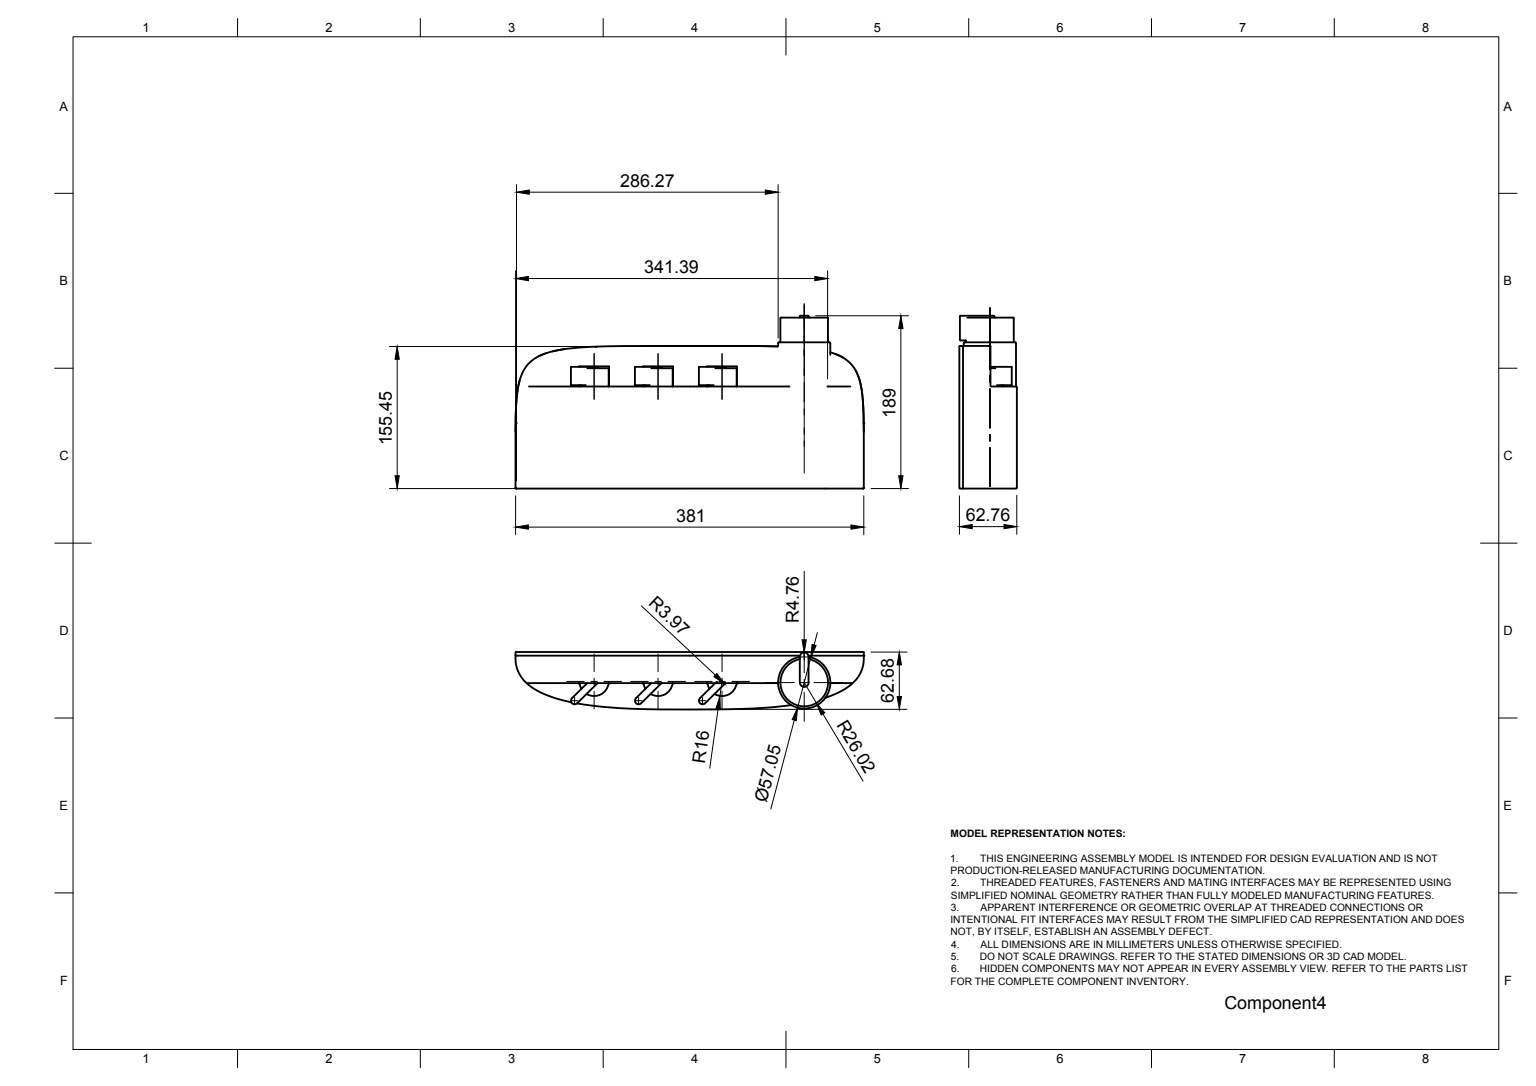
ISO-10303-21;
HEADER;
/* Generated by software containing ST-Developer
 * from STEP Tools, Inc. (www.steptools.com) 
 */

FILE_DESCRIPTION(
/* description */ ('STEP AP214'),
/* implementation_level */ '2;1');

FILE_NAME(
/* name */ 'Component4.step',
/* time_stamp */ '2026-10-06T11:02:40-07:00',
/* author */ (''),
/* organization */ (''),
/* preprocessor_version */ 'ST-DEVELOPER v20.2',
/* originating_system */ 'Autodesk Translation Framework v15.15.0.0',
/* authorisation */ '');

FILE_SCHEMA (('AUTOMOTIVE_DESIGN { 1 0 10303 214 3 1 1 }'));
ENDSEC;

DATA;
#10=MECHANICAL_DESIGN_GEOMETRIC_PRESENTATION_REPRESENTATION('',(#2939),#130910);
#50=B_SPLINE_SURFACE_WITH_KNOTS('',3,1,((#87618,#87619),(#87620,#87621),
(#87622,#87623),(#87624,#87625)),.UNSPECIFIED.,.F.,.F.,.F.,(4,4),(2,2),
(0.0749476459249852,1.),(0.,0.360000000000005),.UNSPECIFIED.);
#51=B_SPLINE_SURFACE_WITH_KNOTS('',3,1,((#88063,#88064),(#88065,#88066),
(#88067,#88068),(#88069,#88070)),.UNSPECIFIED.,.F.,.F.,.F.,(4,4),(2,2),
(0.,0.925052354075012),(0.,0.360000000000003),.UNSPECIFIED.);
#52=B_SPLINE_SURFACE_WITH_KNOTS('',3,1,((#96549,#96550),(#96551,#96552),
(#96553,#96554),(#96555,#96556)),.UNSPECIFIED.,.F.,.F.,.F.,(4,4),(2,2),
(0.0749476459249852,1.),(0.,3.46611820003485),.UNSPECIFIED.);
#53=B_SPLINE_SURFACE_WITH_KNOTS('',3,1,((#96558,#96559),(#96560,#96561),
(#96562,#96563),(#96564,#96565)),.UNSPECIFIED.,.F.,.F.,.F.,(4,4),(2,2),
(0.309194334580351,0.92505235407501),(0.,1.8569103791729),.UNSPECIFIED.);
#54=B_SPLINE_SURFACE_WITH_KNOTS('',3,1,((#96571,#96572),(#96573,#96574),
(#96575,#96576),(#96577,#96578)),.UNSPECIFIED.,.F.,.F.,.F.,(4,4),(2,2),
(0.62139116379009,1.),(0.,13.1529900906224),.UNSPECIFIED.);
#55=B_SPLINE_SURFACE_WITH_KNOTS('',3,1,((#96579,#96580),(#96581,#96582),
(#96583,#96584),(#96585,#96586)),.UNSPECIFIED.,.F.,.F.,.F.,(4,4),(2,2),
(0.,1.),(0.,13.1529900906224),.UNSPECIFIED.);
#56=B_SPLINE_SURFACE_WITH_KNOTS('',3,1,((#96901,#96902),(#96903,#96904),
(#96905,#96906),(#96907,#96908)),.UNSPECIFIED.,.F.,.F.,.F.,(4,4),(2,2),
(0.,0.448741420101952),(0.,13.1529900906224),.UNSPECIFIED.);
#57=B_SPLINE_SURFACE_WITH_KNOTS('',3,1,((#96909,#96910),(#96911,#96912),
(#96913,#96914),(#96915,#96916)),.UNSPECIFIED.,.F.,.F.,.F.,(4,4),(2,2),
(0.,0.274332977827422),(0.,3.42421373123634),.UNSPECIFIED.);
#60=SPHERICAL_SURFACE('',#48303,0.5);
#61=SPHERICAL_SURFACE('',#48305,0.5);
#62=SPHERICAL_SURFACE('',#48314,0.5);
#63=SPHERICAL_SURFACE('',#48316,0.5);
#64=SPHERICAL_SURFACE('',#48525,1.);
#65=SPHERICAL_SURFACE('',#48533,1.);
#717=FACE_BOUND('',#15125,.T.);
#718=FACE_BOUND('',#15135,.T.);
#719=FACE_BOUND('',#15136,.T.);
#720=FACE_BOUND('',#15137,.T.);
#1607=(
BOUNDED_SURFACE()
B_SPLINE_SURFACE(3,2,((#88517,#88518,#88519),(#88520,#88521,#88522),(#88523,
#88524,#88525),(#88526,#88527,#88528),(#88529,#88530,#88531),(#88532,#88533,
#88534),(#88535,#88536,#88537),(#88538,#88539,#88540),(#88541,#88542,#88543),
(#88544,#88545,#88546),(#88547,#88548,#88549),(#88550,#88551,#88552),(#88553,
#88554,#88555),(#88556,#88557,#88558),(#88559,#88560,#88561),(#88562,#88563,
#88564),(#88565,#88566,#88567),(#88568,#88569,#88570),(#88571,#88572,#88573),
(#88574,#88575,#88576),(#88577,#88578,#88579),(#88580,#88581,#88582),(#88583,
#88584,#88585),(#88586,#88587,#88588),(#88589,#88590,#88591),(#88592,#88593,
#88594),(#88595,#88596,#88597),(#88598,#88599,#88600),(#88601,#88602,#88603),
(#88604,#88605,#88606),(#88607,#88608,#88609),(#88610,#88611,#88612),(#88613,
#88614,#88615),(#88616,#88617,#88618),(#88619,#88620,#88621),(#88622,#88623,
#88624),(#88625,#88626,#88627),(#88628,#88629,#88630),(#88631,#88632,#88633),
(#88634,#88635,#88636),(#88637,#88638,#88639),(#88640,#88641,#88642),(#88643,
#88644,#88645),(#88646,#88647,#88648),(#88649,#88650,#88651),(#88652,#88653,
#88654),(#88655,#88656,#88657),(#88658,#88659,#88660),(#88661,#88662,#88663),
(#88664,#88665,#88666),(#88667,#88668,#88669),(#88670,#88671,#88672),(#88673,
#88674,#88675),(#88676,#88677,#88678),(#88679,#88680,#88681),(#88682,#88683,
#88684),(#88685,#88686,#88687),(#88688,#88689,#88690)),.UNSPECIFIED.,.F.,
 .F.,.F.)
B_SPLINE_SURFACE_WITH_KNOTS((4,2,2,2,2,2,2,2,2,2,2,2,2,2,2,2,2,2,2,2,2,
2,2,2,2,2,2,2,4),(3,3),(0.,0.0321349777273596,0.0642699554547192,0.080337444318399,
0.0964049331820788,0.112472422045759,0.128539910909438,0.136573655341278,
0.140590527557198,0.144607399773118,0.152641144204958,0.156658016420878,
0.160674888636798,0.168708633068638,0.172725505284558,0.174733941392518,
0.176742377500478,0.184776121932318,0.186784558040278,0.188792994148238,
0.192809866364158,0.200843610795998,0.204860483011918,0.208877355227837,
0.216911099659677,0.224944844091517,0.232978588523357,0.241012332955197,
0.25739509415827),(0.295972225728062,1.),.UNSPECIFIED.)
GEOMETRIC_REPRESENTATION_ITEM()
RATIONAL_B_SPLINE_SURFACE(((0.877938117508499,0.793795039059425,1.),(0.877938117508499,
0.793795039059425,1.),(0.877938117508498,0.793795039059421,1.),(0.877938117508498,
0.793795039059421,1.),(0.877938117508498,0.793795039059421,1.),(0.877938117508498,
0.793795039059421,1.),(0.877938117508498,0.793795039059421,1.),(0.877938117508498,
0.793795039059421,1.),(0.877938117508499,0.793795039059425,1.),(0.877938117508499,
0.793795039059425,1.),(0.877938117508489,0.793795039059407,1.),(0.877938117508489,
0.793795039059407,1.),(0.877938117508506,0.793795039059435,1.),(0.877938117508506,
0.793795039059435,1.),(0.877938117508499,0.793795039059425,1.),(0.877938117508499,
0.793795039059425,1.),(0.877938117508499,0.793795039059425,1.),(0.877938117508499,
0.793795039059425,1.),(0.877938117508498,0.793795039059421,1.),(0.877938117508498,
0.793795039059421,1.),(0.877938117508485,0.793795039059401,1.),(0.877938117508485,
0.793795039059401,1.),(0.877938117508505,0.793795039059434,1.),(0.877938117508505,
0.793795039059434,1.),(0.87793811750849,0.793795039059408,1.),(0.87793811750849,
0.793795039059408,1.),(0.87793811750849,0.793795039059409,1.),(0.87793811750849,
0.793795039059409,1.),(0.877938117508486,0.793795039059402,1.),(0.877938117508486,
0.793795039059402,1.),(0.877938117508504,0.793795039059432,1.),(0.877938117508504,
0.793795039059432,1.),(0.877938117508498,0.793795039059421,1.),(0.877938117508498,
0.793795039059421,1.),(0.877938117508506,0.793795039059436,1.),(0.877938117508506,
0.793795039059436,1.),(0.877938117508498,0.793795039059421,1.),(0.877938117508498,
0.793795039059421,1.),(0.877938117508493,0.793795039059414,1.),(0.877938117508493,
0.793795039059414,1.),(0.877938117508498,0.793795039059421,1.),(0.877938117508498,
0.793795039059421,1.),(0.877938117508498,0.793795039059421,1.),(0.877938117508498,
0.793795039059421,1.),(0.877938117508489,0.793795039059408,1.),(0.877938117508489,
0.793795039059408,1.),(0.877938117508506,0.793795039059435,1.),(0.877938117508506,
0.793795039059435,1.),(0.877938117508489,0.793795039059408,1.),(0.877938117508489,
0.793795039059408,1.),(0.877938117508498,0.793795039059421,1.),(0.877938117508498,
0.793795039059421,1.),(0.877938117508506,0.793795039059435,1.),(0.877938117508506,
0.793795039059435,1.),(0.877938117508506,0.793795039059435,1.),(0.877938117508506,
0.793795039059435,1.),(0.877938117508499,0.793795039059424,1.),(0.877938117508499,
0.793795039059425,1.)))
REPRESENTATION_ITEM('')
SURFACE()
);
#1608=(
BOUNDED_SURFACE()
B_SPLINE_SURFACE(3,2,((#88828,#88829,#88830),(#88831,#88832,#88833),(#88834,
#88835,#88836),(#88837,#88838,#88839),(#88840,#88841,#88842),(#88843,#88844,
#88845),(#88846,#88847,#88848),(#88849,#88850,#88851),(#88852,#88853,#88854),
(#88855,#88856,#88857),(#88858,#88859,#88860),(#88861,#88862,#88863),(#88864,
#88865,#88866),(#88867,#88868,#88869),(#88870,#88871,#88872),(#88873,#88874,
#88875),(#88876,#88877,#88878),(#88879,#88880,#88881),(#88882,#88883,#88884),
(#88885,#88886,#88887),(#88888,#88889,#88890),(#88891,#88892,#88893),(#88894,
#88895,#88896),(#88897,#88898,#88899),(#88900,#88901,#88902),(#88903,#88904,
#88905),(#88906,#88907,#88908),(#88909,#88910,#88911),(#88912,#88913,#88914),
(#88915,#88916,#88917),(#88918,#88919,#88920),(#88921,#88922,#88923),(#88924,
#88925,#88926),(#88927,#88928,#88929),(#88930,#88931,#88932),(#88933,#88934,
#88935),(#88936,#88937,#88938),(#88939,#88940,#88941),(#88942,#88943,#88944),
(#88945,#88946,#88947),(#88948,#88949,#88950),(#88951,#88952,#88953),(#88954,
#88955,#88956),(#88957,#88958,#88959),(#88960,#88961,#88962),(#88963,#88964,
#88965),(#88966,#88967,#88968),(#88969,#88970,#88971),(#88972,#88973,#88974),
(#88975,#88976,#88977),(#88978,#88979,#88980),(#88981,#88982,#88983),(#88984,
#88985,#88986),(#88987,#88988,#88989),(#88990,#88991,#88992),(#88993,#88994,
#88995)),.UNSPECIFIED.,.F.,.F.,.F.)
B_SPLINE_SURFACE_WITH_KNOTS((4,2,2,2,2,2,2,2,2,2,2,2,2,2,2,2,2,2,2,2,2,
2,2,2,2,2,2,4),(3,3),(0.,0.0161428187212414,0.0242142280818621,0.0322856374424828,
0.0403570468031035,0.0484284561637242,0.0564998655243449,0.0605355702046552,
0.0645712748849656,0.0686069795652759,0.0706248319054311,0.0726426842455863,
0.0807140936062069,0.0847497982865173,0.0867676506266725,0.0887855029668276,
0.0968569123274483,0.100892617007759,0.104928321688069,0.11299973104869,
0.12107114040931,0.129142549769931,0.145285368491173,0.161428187212414,
0.177571005933655,0.193713824654897,0.225999462097379,0.258285099539862),
(0.296287498067819,1.),.UNSPECIFIED.)
GEOMETRIC_REPRESENTATION_ITEM()
RATIONAL_B_SPLINE_SURFACE(((0.877862815112484,0.793887380189833,1.),(0.877862815112484,
0.793887380189833,1.),(0.877862815112466,0.793887380189802,1.),(0.877862815112466,
0.793887380189802,1.),(0.87786281511247,0.793887380189809,1.),(0.87786281511247,
0.793887380189809,1.),(0.877862815112476,0.793887380189819,1.),(0.877862815112476,
0.793887380189819,1.),(0.877862815112474,0.793887380189816,1.),(0.877862815112474,
0.793887380189816,1.),(0.877862815112474,0.793887380189816,1.),(0.877862815112474,
0.793887380189816,1.),(0.877862815112476,0.793887380189819,1.),(0.877862815112476,
0.793887380189819,1.),(0.877862815112474,0.793887380189816,1.),(0.877862815112474,
0.793887380189816,1.),(0.877862815112481,0.793887380189828,1.),(0.877862815112481,
0.793887380189828,1.),(0.877862815112485,0.793887380189834,1.),(0.877862815112485,
0.793887380189834,1.),(0.877862815112478,0.793887380189823,1.),(0.877862815112478,
0.793887380189823,1.),(0.877862815112464,0.7938873801898,1.),(0.877862815112464,
0.7938873801898,1.),(0.877862815112474,0.793887380189816,1.),(0.877862815112474,
0.793887380189816,1.),(0.877862815112474,0.793887380189816,1.),(0.877862815112474,
0.793887380189816,1.),(0.877862815112474,0.793887380189816,1.),(0.877862815112474,
0.793887380189816,1.),(0.877862815112474,0.793887380189816,1.),(0.877862815112474,
0.793887380189816,1.),(0.877862815112472,0.793887380189812,1.),(0.877862815112472,
0.793887380189812,1.),(0.877862815112482,0.793887380189829,1.),(0.877862815112482,
0.793887380189829,1.),(0.877862815112466,0.793887380189802,1.),(0.877862815112466,
0.793887380189802,1.),(0.877862815112476,0.793887380189819,1.),(0.877862815112476,
0.793887380189819,1.),(0.877862815112466,0.793887380189802,1.),(0.877862815112466,
0.793887380189802,1.),(0.877862815112474,0.793887380189816,1.),(0.877862815112474,
0.793887380189816,1.),(0.877862815112474,0.793887380189815,1.),(0.877862815112474,
0.793887380189815,1.),(0.877862815112484,0.793887380189833,1.),(0.877862815112484,
0.793887380189833,1.),(0.877862815112461,0.793887380189795,1.),(0.877862815112461,
0.793887380189795,1.),(0.877862815112466,0.793887380189802,1.),(0.877862815112466,
0.793887380189802,1.),(0.877862815112474,0.793887380189816,1.),(0.877862815112474,
0.793887380189816,1.),(0.877862815112476,0.793887380189819,1.),(0.877862815112476,
0.793887380189819,1.)))
REPRESENTATION_ITEM('')
SURFACE()
);
#1609=(
BOUNDED_SURFACE()
B_SPLINE_SURFACE(3,2,((#89355,#89356,#89357),(#89358,#89359,#89360),(#89361,
#89362,#89363),(#89364,#89365,#89366),(#89367,#89368,#89369),(#89370,#89371,
#89372),(#89373,#89374,#89375),(#89376,#89377,#89378),(#89379,#89380,#89381),
(#89382,#89383,#89384),(#89385,#89386,#89387),(#89388,#89389,#89390),(#89391,
#89392,#89393),(#89394,#89395,#89396),(#89397,#89398,#89399),(#89400,#89401,
#89402),(#89403,#89404,#89405),(#89406,#89407,#89408),(#89409,#89410,#89411),
(#89412,#89413,#89414),(#89415,#89416,#89417),(#89418,#89419,#89420),(#89421,
#89422,#89423),(#89424,#89425,#89426),(#89427,#89428,#89429),(#89430,#89431,
#89432),(#89433,#89434,#89435),(#89436,#89437,#89438),(#89439,#89440,#89441),
(#89442,#89443,#89444),(#89445,#89446,#89447),(#89448,#89449,#89450),(#89451,
#89452,#89453),(#89454,#89455,#89456),(#89457,#89458,#89459),(#89460,#89461,
#89462),(#89463,#89464,#89465),(#89466,#89467,#89468),(#89469,#89470,#89471),
(#89472,#89473,#89474),(#89475,#89476,#89477),(#89478,#89479,#89480),(#89481,
#89482,#89483),(#89484,#89485,#89486),(#89487,#89488,#89489),(#89490,#89491,
#89492),(#89493,#89494,#89495),(#89496,#89497,#89498),(#89499,#89500,#89501),
(#89502,#89503,#89504),(#89505,#89506,#89507),(#89508,#89509,#89510),(#89511,
#89512,#89513),(#89514,#89515,#89516),(#89517,#89518,#89519),(#89520,#89521,
#89522)),.UNSPECIFIED.,.F.,.F.,.F.)
B_SPLINE_SURFACE_WITH_KNOTS((4,2,2,2,2,2,2,2,2,2,2,2,2,2,2,2,2,2,2,2,2,
2,2,2,2,2,2,4),(3,3),(0.,0.0161428187212413,0.024214228081862,0.0322856374424827,
0.0403570468031034,0.048428456163724,0.0564998655243447,0.060535570204655,
0.0645712748849654,0.0686069795652757,0.0706248319054309,0.072642684245586,
0.0807140936062067,0.084749798286517,0.0867676506266722,0.0887855029668274,
0.0968569123274481,0.100892617007758,0.104928321688069,0.112999731048689,
0.12107114040931,0.129142549769931,0.145285368491172,0.161428187212413,
0.177571005933655,0.193713824654896,0.225999462097379,0.258285099539862),
(0.,1.),.UNSPECIFIED.)
GEOMETRIC_REPRESENTATION_ITEM()
RATIONAL_B_SPLINE_SURFACE(((1.,0.707106781186543,1.),(1.,0.707106781186543,
1.),(1.,0.707106781186528,1.),(1.,0.707106781186528,1.),(1.,0.707106781186548,
1.),(1.,0.707106781186548,1.),(1.,0.707106781186548,1.),(1.,0.707106781186548,
1.),(1.,0.707106781186533,1.),(1.,0.707106781186533,1.),(1.,0.707106781186557,
1.),(1.,0.707106781186557,1.),(1.,0.707106781186548,1.),(1.,0.707106781186548,
1.),(1.,0.707106781186548,1.),(1.,0.707106781186548,1.),(1.,0.707106781186548,
1.),(1.,0.707106781186548,1.),(1.,0.707106781186548,1.),(1.,0.707106781186548,
1.),(1.,0.707106781186564,1.),(1.,0.707106781186564,1.),(1.,0.707106781186562,
1.),(1.,0.707106781186562,1.),(1.,0.707106781186548,1.),(1.,0.707106781186548,
1.),(1.,0.707106781186559,1.),(1.,0.707106781186559,1.),(1.,0.707106781186537,
1.),(1.,0.707106781186537,1.),(1.,0.707106781186579,1.),(1.,0.707106781186579,
1.),(1.,0.707106781186543,1.),(1.,0.707106781186543,1.),(1.,0.707106781186548,
1.),(1.,0.707106781186548,1.),(1.,0.707106781186562,1.),(1.,0.707106781186562,
1.),(1.,0.707106781186533,1.),(1.,0.707106781186533,1.),(1.,0.707106781186562,
1.),(1.,0.707106781186562,1.),(1.,0.707106781186548,1.),(1.,0.707106781186548,
1.),(1.,0.707106781186548,1.),(1.,0.707106781186548,1.),(1.,0.707106781186547,
1.),(1.,0.707106781186547,1.),(1.,0.707106781186548,1.),(1.,0.707106781186548,
1.),(1.,0.707106781186548,1.),(1.,0.707106781186548,1.),(1.,0.707106781186543,
1.),(1.,0.707106781186543,1.),(1.,0.707106781186543,1.),(1.,0.707106781186543,
1.)))
REPRESENTATION_ITEM('')
SURFACE()
);
#1610=(
BOUNDED_SURFACE()
B_SPLINE_SURFACE(3,2,((#89524,#89525,#89526),(#89527,#89528,#89529),(#89530,
#89531,#89532),(#89533,#89534,#89535),(#89536,#89537,#89538),(#89539,#89540,
#89541),(#89542,#89543,#89544),(#89545,#89546,#89547),(#89548,#89549,#89550),
(#89551,#89552,#89553),(#89554,#89555,#89556),(#89557,#89558,#89559),(#89560,
#89561,#89562),(#89563,#89564,#89565),(#89566,#89567,#89568),(#89569,#89570,
#89571),(#89572,#89573,#89574),(#89575,#89576,#89577),(#89578,#89579,#89580),
(#89581,#89582,#89583),(#89584,#89585,#89586),(#89587,#89588,#89589),(#89590,
#89591,#89592),(#89593,#89594,#89595),(#89596,#89597,#89598),(#89599,#89600,
#89601),(#89602,#89603,#89604),(#89605,#89606,#89607),(#89608,#89609,#89610),
(#89611,#89612,#89613),(#89614,#89615,#89616),(#89617,#89618,#89619),(#89620,
#89621,#89622),(#89623,#89624,#89625),(#89626,#89627,#89628),(#89629,#89630,
#89631),(#89632,#89633,#89634),(#89635,#89636,#89637),(#89638,#89639,#89640),
(#89641,#89642,#89643),(#89644,#89645,#89646),(#89647,#89648,#89649),(#89650,
#89651,#89652),(#89653,#89654,#89655),(#89656,#89657,#89658),(#89659,#89660,
#89661),(#89662,#89663,#89664),(#89665,#89666,#89667),(#89668,#89669,#89670),
(#89671,#89672,#89673),(#89674,#89675,#89676),(#89677,#89678,#89679),(#89680,
#89681,#89682),(#89683,#89684,#89685),(#89686,#89687,#89688),(#89689,#89690,
#89691),(#89692,#89693,#89694),(#89695,#89696,#89697)),.UNSPECIFIED.,.F.,
 .F.,.F.)
B_SPLINE_SURFACE_WITH_KNOTS((4,2,2,2,2,2,2,2,2,2,2,2,2,2,2,2,2,2,2,2,2,
2,2,2,2,2,2,2,4),(3,3),(0.,0.0321349777273597,0.0642699554547194,0.0803374443183993,
0.0964049331820791,0.112472422045759,0.128539910909439,0.136573655341279,
0.140590527557199,0.144607399773119,0.152641144204959,0.156658016420879,
0.160674888636799,0.168708633068638,0.172725505284558,0.174733941392518,
0.176742377500478,0.184776121932318,0.186784558040278,0.188792994148238,
0.192809866364158,0.200843610795998,0.204860483011918,0.208877355227838,
0.216911099659678,0.224944844091518,0.232978588523358,0.241012332955198,
0.257079821818878),(0.,1.),.UNSPECIFIED.)
GEOMETRIC_REPRESENTATION_ITEM()
RATIONAL_B_SPLINE_SURFACE(((1.,0.707106781186543,1.),(1.,0.707106781186543,
1.),(1.,0.707106781186543,1.),(1.,0.707106781186543,1.),(1.,0.707106781186548,
1.),(1.,0.707106781186548,1.),(1.,0.707106781186548,1.),(1.,0.707106781186548,
1.),(1.,0.707106781186548,1.),(1.,0.707106781186548,1.),(1.,0.707106781186553,
1.),(1.,0.707106781186553,1.),(1.,0.707106781186567,1.),(1.,0.707106781186567,
1.),(1.,0.707106781186533,1.),(1.,0.707106781186533,1.),(1.,0.707106781186552,
1.),(1.,0.707106781186552,1.),(1.,0.707106781186572,1.),(1.,0.707106781186572,
1.),(1.,0.707106781186552,1.),(1.,0.707106781186552,1.),(1.,0.707106781186552,
1.),(1.,0.707106781186552,1.),(1.,0.707106781186561,1.),(1.,0.707106781186561,
1.),(1.,0.707106781186543,1.),(1.,0.707106781186543,1.),(1.,0.707106781186552,
1.),(1.,0.707106781186552,1.),(1.,0.707106781186558,1.),(1.,0.707106781186558,
1.),(1.,0.707106781186543,1.),(1.,0.707106781186543,1.),(1.,0.707106781186552,
1.),(1.,0.707106781186552,1.),(1.,0.707106781186532,1.),(1.,0.707106781186532,
1.),(1.,0.707106781186533,1.),(1.,0.707106781186533,1.),(1.,0.707106781186543,
1.),(1.,0.707106781186543,1.),(1.,0.707106781186543,1.),(1.,0.707106781186543,
1.),(1.,0.707106781186543,1.),(1.,0.707106781186543,1.),(1.,0.707106781186543,
1.),(1.,0.707106781186543,1.),(1.,0.707106781186538,1.),(1.,0.707106781186538,
1.),(1.,0.707106781186552,1.),(1.,0.707106781186552,1.),(1.,0.707106781186572,
1.),(1.,0.707106781186572,1.),(1.,0.707106781186552,1.),(1.,0.707106781186552,
1.),(1.,0.707106781186528,1.),(1.,0.707106781186528,1.)))
REPRESENTATION_ITEM('')
SURFACE()
);
#1611=(
BOUNDED_SURFACE()
B_SPLINE_SURFACE(3,2,((#89728,#89729,#89730),(#89731,#89732,#89733),(#89734,
#89735,#89736),(#89737,#89738,#89739),(#89740,#89741,#89742),(#89743,#89744,
#89745),(#89746,#89747,#89748),(#89749,#89750,#89751),(#89752,#89753,#89754),
(#89755,#89756,#89757),(#89758,#89759,#89760),(#89761,#89762,#89763)),
 .UNSPECIFIED.,.F.,.F.,.F.)
B_SPLINE_SURFACE_WITH_KNOTS((4,2,2,2,2,4),(3,3),(0.000926277054046903,0.00147787442090103,
0.00175367310432809,0.00202947178775516,0.00258106915460929,0.00313266652146341),
(0.,1.),.UNSPECIFIED.)
GEOMETRIC_REPRESENTATION_ITEM()
RATIONAL_B_SPLINE_SURFACE(((1.,0.775937515965206,1.),(1.,0.775965554436259,
1.),(1.,0.773720199380605,1.),(1.,0.767576773145645,1.),(1.,0.765096790635356,
1.),(1.,0.759365493434644,1.),(1.,0.756099558648518,1.),(1.,0.745708436761125,
1.),(1.,0.737726760693873,1.),(1.,0.721983931595965,1.),(1.,0.714015299600668,
1.),(1.,0.707106781186543,1.)))
REPRESENTATION_ITEM('')
SURFACE()
);
#1612=(
BOUNDED_SURFACE()
B_SPLINE_SURFACE(3,2,((#89809,#89810,#89811),(#89812,#89813,#89814),(#89815,
#89816,#89817),(#89818,#89819,#89820),(#89821,#89822,#89823),(#89824,#89825,
#89826),(#89827,#89828,#89829),(#89830,#89831,#89832),(#89833,#89834,#89835),
(#89836,#89837,#89838),(#89839,#89840,#89841),(#89842,#89843,#89844)),
 .UNSPECIFIED.,.F.,.F.,.F.)
B_SPLINE_SURFACE_WITH_KNOTS((4,2,2,2,2,4),(3,3),(0.000925070050461762,0.00147866127618651,
0.00175545688904888,0.00203225250191126,0.00258584372763601,0.00313943495336076),
(0.,1.),.UNSPECIFIED.)
GEOMETRIC_REPRESENTATION_ITEM()
RATIONAL_B_SPLINE_SURFACE(((1.,0.775937515965214,1.),(1.,0.775948908187678,
1.),(1.,0.7742815251738,1.),(1.,0.769435561772286,1.),(1.,0.767450319305812,
1.),(1.,0.762709308920971,1.),(1.,0.75994120696576,1.),(1.,0.750761268625032,
1.),(1.,0.743229618394193,1.),(1.,0.726398019745837,1.),(1.,0.716867225806667,
1.),(1.,0.707106781186526,1.)))
REPRESENTATION_ITEM('')
SURFACE()
);
#1613=(
BOUNDED_SURFACE()
B_SPLINE_SURFACE(3,2,((#89924,#89925,#89926),(#89927,#89928,#89929),(#89930,
#89931,#89932),(#89933,#89934,#89935),(#89936,#89937,#89938),(#89939,#89940,
#89941),(#89942,#89943,#89944),(#89945,#89946,#89947),(#89948,#89949,#89950),
(#89951,#89952,#89953),(#89954,#89955,#89956),(#89957,#89958,#89959)),
 .UNSPECIFIED.,.F.,.F.,.F.)
B_SPLINE_SURFACE_WITH_KNOTS((4,2,2,2,2,4),(3,3),(0.000954052972318673,0.00150562533929701,
0.00178141152278617,0.00205719770627534,0.00260877007325367,0.003160342440232),
(0.,1.),.UNSPECIFIED.)
GEOMETRIC_REPRESENTATION_ITEM()
RATIONAL_B_SPLINE_SURFACE(((1.,0.707106781186548,1.),(1.,0.714095715093505,
1.),(1.,0.721962502896922,1.),(1.,0.733852450860903,1.),(1.,0.737775695415353,
1.),(1.,0.745441210409867,1.),(1.,0.749210335263833,1.),(1.,0.759607646869478,
1.),(1.,0.765574863587299,1.),(1.,0.773709421852012,1.),(1.,0.775971965811445,
1.),(1.,0.775937515965212,1.)))
REPRESENTATION_ITEM('')
SURFACE()
);
#1614=(
BOUNDED_SURFACE()
B_SPLINE_SURFACE(3,2,((#90005,#90006,#90007),(#90008,#90009,#90010),(#90011,
#90012,#90013),(#90014,#90015,#90016),(#90017,#90018,#90019),(#90020,#90021,
#90022),(#90023,#90024,#90025),(#90026,#90027,#90028),(#90029,#90030,#90031),
(#90032,#90033,#90034),(#90035,#90036,#90037),(#90038,#90039,#90040)),
 .UNSPECIFIED.,.F.,.F.,.F.)
B_SPLINE_SURFACE_WITH_KNOTS((4,2,2,2,2,4),(3,3),(0.000982297288438947,0.0015357772992534,
0.00181251730466063,0.00208925731006786,0.00264273732088231,0.00319621733169676),
(0.,1.),.UNSPECIFIED.)
GEOMETRIC_REPRESENTATION_ITEM()
RATIONAL_B_SPLINE_SURFACE(((1.,0.707106781186548,1.),(1.,0.716971715675457,
1.),(1.,0.726372587537382,1.),(1.,0.739082989278526,1.),(1.,0.743030515251258,
1.),(1.,0.75040043255623,1.),(1.,0.753848954137035,1.),(1.,0.763039215535026,
1.),(1.,0.767853458839658,1.),(1.,0.774273736205767,1.),(1.,0.7759516406652,
1.),(1.,0.775937515965214,1.)))
REPRESENTATION_ITEM('')
SURFACE()
);
#1615=(
BOUNDED_SURFACE()
B_SPLINE_SURFACE(3,2,((#90152,#90153,#90154),(#90155,#90156,#90157),(#90158,
#90159,#90160),(#90161,#90162,#90163),(#90164,#90165,#90166),(#90167,#90168,
#90169),(#90170,#90171,#90172),(#90173,#90174,#90175),(#90176,#90177,#90178),
(#90179,#90180,#90181)),.UNSPECIFIED.,.F.,.F.,.F.)
B_SPLINE_SURFACE_WITH_KNOTS((4,2,2,2,4),(3,3),(0.000653855251160619,0.00105056734621481,
0.00144727944126899,0.00184399153632318,0.00224070363137736),(0.,1.),
 .UNSPECIFIED.)
GEOMETRIC_REPRESENTATION_ITEM()
RATIONAL_B_SPLINE_SURFACE(((1.,0.797116436093323,1.),(1.,0.797153870787656,
1.),(1.,0.794288909474886,1.),(1.,0.78384172562724,1.),(1.,0.776220388773547,
1.),(1.,0.758398453086649,1.),(1.,0.748065045409874,1.),(1.,0.727318436656279,
1.),(1.,0.716633802230093,1.),(1.,0.707106781186546,1.)))
REPRESENTATION_ITEM('')
SURFACE()
);
#1616=(
BOUNDED_SURFACE()
B_SPLINE_SURFACE(3,2,((#90227,#90228,#90229),(#90230,#90231,#90232),(#90233,
#90234,#90235),(#90236,#90237,#90238),(#90239,#90240,#90241),(#90242,#90243,
#90244),(#90245,#90246,#90247),(#90248,#90249,#90250),(#90251,#90252,#90253),
(#90254,#90255,#90256)),.UNSPECIFIED.,.F.,.F.,.F.)
B_SPLINE_SURFACE_WITH_KNOTS((4,2,2,2,4),(3,3),(0.000346079680846979,0.000742789375765937,
0.0011394990706849,0.00153620876560385,0.00193291846052281),(0.,1.),
 .UNSPECIFIED.)
GEOMETRIC_REPRESENTATION_ITEM()
RATIONAL_B_SPLINE_SURFACE(((1.,0.707106781186546,1.),(1.,0.716758952028491,
1.),(1.,0.727288011548078,1.),(1.,0.748184897298097,1.),(1.,0.758437122287583,
1.),(1.,0.776285930138696,1.),(1.,0.783895918656499,1.),(1.,0.794279688273945,
1.),(1.,0.797152913684426,1.),(1.,0.797116436093324,1.)))
REPRESENTATION_ITEM('')
SURFACE()
);
#1617=(
BOUNDED_SURFACE()
B_SPLINE_SURFACE(3,2,((#90319,#90320,#90321),(#90322,#90323,#90324),(#90325,
#90326,#90327),(#90328,#90329,#90330),(#90331,#90332,#90333),(#90334,#90335,
#90336),(#90337,#90338,#90339),(#90340,#90341,#90342),(#90343,#90344,#90345),
(#90346,#90347,#90348)),.UNSPECIFIED.,.F.,.F.,.F.)
B_SPLINE_SURFACE_WITH_KNOTS((4,2,2,2,4),(3,3),(0.000652435349851691,0.00105161226574612,
0.00145078918164054,0.00184996609753497,0.00224914301342939),(0.,1.),
 .UNSPECIFIED.)
GEOMETRIC_REPRESENTATION_ITEM()
RATIONAL_B_SPLINE_SURFACE(((1.,0.797116436093325,1.),(1.,0.797133991687376,
1.),(1.,0.794952627585106,1.),(1.,0.786540751799673,1.),(1.,0.780263959283907,
1.),(1.,0.764334803592024,1.),(1.,0.754537231252642,1.),(1.,0.73252430168142,
1.),(1.,0.720028936379281,1.),(1.,0.707106781186558,1.)))
REPRESENTATION_ITEM('')
SURFACE()
);
#1618=(
BOUNDED_SURFACE()
B_SPLINE_SURFACE(3,2,((#90394,#90395,#90396),(#90397,#90398,#90399),(#90400,
#90401,#90402),(#90403,#90404,#90405),(#90406,#90407,#90408),(#90409,#90410,
#90411),(#90412,#90413,#90414),(#90415,#90416,#90417),(#90418,#90419,#90420),
(#90421,#90422,#90423)),.UNSPECIFIED.,.F.,.F.,.F.)
B_SPLINE_SURFACE_WITH_KNOTS((4,2,2,2,4),(3,3),(0.000364014256986725,0.000763079051988796,
0.00116214384699087,0.00156120864199294,0.00196027343699501),(0.,1.),
 .UNSPECIFIED.)
GEOMETRIC_REPRESENTATION_ITEM()
RATIONAL_B_SPLINE_SURFACE(((1.,0.707106781186567,1.),(1.,0.720184284287166,
1.),(1.,0.73248314811275,1.),(1.,0.754654774294656,1.),(1.,0.764346716512339,
1.),(1.,0.780321857768423,1.),(1.,0.786575289610347,1.),(1.,0.794947899012155,
1.),(1.,0.797127700950814,1.),(1.,0.797116436093325,1.)))
REPRESENTATION_ITEM('')
SURFACE()
);
#1619=(
BOUNDED_SURFACE()
B_SPLINE_SURFACE(3,2,((#90516,#90517,#90518),(#90519,#90520,#90521),(#90522,
#90523,#90524),(#90525,#90526,#90527),(#90528,#90529,#90530),(#90531,#90532,
#90533),(#90534,#90535,#90536),(#90537,#90538,#90539),(#90540,#90541,#90542),
(#90543,#90544,#90545)),.UNSPECIFIED.,.F.,.F.,.F.)
B_SPLINE_SURFACE_WITH_KNOTS((4,2,2,2,4),(3,3),(0.000653855251160618,0.0010505673462148,
0.00144727944126899,0.00184399153632318,0.00224070363137736),(0.,1.),
 .UNSPECIFIED.)
GEOMETRIC_REPRESENTATION_ITEM()
RATIONAL_B_SPLINE_SURFACE(((1.,0.797116436093328,1.),(1.,0.797153870787879,
1.),(1.,0.794288909474585,1.),(1.,0.783841725627543,1.),(1.,0.776220388773417,
1.),(1.,0.758398453086769,1.),(1.,0.748065045410025,1.),(1.,0.727318436656137,
1.),(1.,0.7166338022302,1.),(1.,0.707106781186548,1.)))
REPRESENTATION_ITEM('')
SURFACE()
);
#1620=(
BOUNDED_SURFACE()
B_SPLINE_SURFACE(3,2,((#90591,#90592,#90593),(#90594,#90595,#90596),(#90597,
#90598,#90599),(#90600,#90601,#90602),(#90603,#90604,#90605),(#90606,#90607,
#90608),(#90609,#90610,#90611),(#90612,#90613,#90614),(#90615,#90616,#90617),
(#90618,#90619,#90620)),.UNSPECIFIED.,.F.,.F.,.F.)
B_SPLINE_SURFACE_WITH_KNOTS((4,2,2,2,4),(3,3),(0.000346079680846979,0.000742789375765937,
0.0011394990706849,0.00153620876560385,0.00193291846052281),(0.,1.),
 .UNSPECIFIED.)
GEOMETRIC_REPRESENTATION_ITEM()
RATIONAL_B_SPLINE_SURFACE(((1.,0.707106781186542,1.),(1.,0.716758952028229,
1.),(1.,0.727288011548429,1.),(1.,0.748184897297752,1.),(1.,0.758437122287011,
1.),(1.,0.776285930139258,1.),(1.,0.783895918655783,1.),(1.,0.794279688274653,
1.),(1.,0.797152913683895,1.),(1.,0.79711643609332,1.)))
REPRESENTATION_ITEM('')
SURFACE()
);
#1621=(
BOUNDED_SURFACE()
B_SPLINE_SURFACE(3,2,((#90683,#90684,#90685),(#90686,#90687,#90688),(#90689,
#90690,#90691),(#90692,#90693,#90694),(#90695,#90696,#90697),(#90698,#90699,
#90700),(#90701,#90702,#90703),(#90704,#90705,#90706),(#90707,#90708,#90709),
(#90710,#90711,#90712)),.UNSPECIFIED.,.F.,.F.,.F.)
B_SPLINE_SURFACE_WITH_KNOTS((4,2,2,2,4),(3,3),(0.000652435349851691,0.00105161226574612,
0.00145078918164054,0.00184996609753497,0.00224914301342939),(0.,1.),
 .UNSPECIFIED.)
GEOMETRIC_REPRESENTATION_ITEM()
RATIONAL_B_SPLINE_SURFACE(((1.,0.797116436093328,1.),(1.,0.797133991687402,
1.),(1.,0.79495262758507,1.),(1.,0.786540751799712,1.),(1.,0.780263959283842,
1.),(1.,0.764334803592092,1.),(1.,0.754537231252535,1.),(1.,0.732524301681536,
1.),(1.,0.720028936379193,1.),(1.,0.707106781186563,1.)))
REPRESENTATION_ITEM('')
SURFACE()
);
#1622=(
BOUNDED_SURFACE()
B_SPLINE_SURFACE(3,2,((#90758,#90759,#90760),(#90761,#90762,#90763),(#90764,
#90765,#90766),(#90767,#90768,#90769),(#90770,#90771,#90772),(#90773,#90774,
#90775),(#90776,#90777,#90778),(#90779,#90780,#90781),(#90782,#90783,#90784),
(#90785,#90786,#90787)),.UNSPECIFIED.,.F.,.F.,.F.)
B_SPLINE_SURFACE_WITH_KNOTS((4,2,2,2,4),(3,3),(0.000364014256986725,0.000763079051988796,
0.00116214384699087,0.00156120864199294,0.00196027343699501),(0.,1.),
 .UNSPECIFIED.)
GEOMETRIC_REPRESENTATION_ITEM()
RATIONAL_B_SPLINE_SURFACE(((1.,0.707106781186571,1.),(1.,0.72018428428724,
1.),(1.,0.732483148112645,1.),(1.,0.75465477429476,1.),(1.,0.764346716512432,
1.),(1.,0.780321857768337,1.),(1.,0.786575289610486,1.),(1.,0.794947899012013,
1.),(1.,0.797127700950917,1.),(1.,0.797116436093326,1.)))
REPRESENTATION_ITEM('')
SURFACE()
);
#1623=(
BOUNDED_SURFACE()
B_SPLINE_SURFACE(3,2,((#90880,#90881,#90882),(#90883,#90884,#90885),(#90886,
#90887,#90888),(#90889,#90890,#90891),(#90892,#90893,#90894),(#90895,#90896,
#90897),(#90898,#90899,#90900),(#90901,#90902,#90903),(#90904,#90905,#90906),
(#90907,#90908,#90909)),.UNSPECIFIED.,.F.,.F.,.F.)
B_SPLINE_SURFACE_WITH_KNOTS((4,2,2,2,4),(3,3),(0.000653855251160619,0.00105056734621481,
0.00144727944126899,0.00184399153632318,0.00224070363137737),(0.,1.),
 .UNSPECIFIED.)
GEOMETRIC_REPRESENTATION_ITEM()
RATIONAL_B_SPLINE_SURFACE(((1.,0.797116436093321,1.),(1.,0.797153870787877,
1.),(1.,0.794288909474591,1.),(1.,0.783841725627535,1.),(1.,0.776220388773692,
1.),(1.,0.7583984530865,1.),(1.,0.748065045409612,1.),(1.,0.727318436656547,
1.),(1.,0.716633802229892,1.),(1.,0.707106781186553,1.)))
REPRESENTATION_ITEM('')
SURFACE()
);
#1624=(
BOUNDED_SURFACE()
B_SPLINE_SURFACE(3,2,((#90955,#90956,#90957),(#90958,#90959,#90960),(#90961,
#90962,#90963),(#90964,#90965,#90966),(#90967,#90968,#90969),(#90970,#90971,
#90972),(#90973,#90974,#90975),(#90976,#90977,#90978),(#90979,#90980,#90981),
(#90982,#90983,#90984)),.UNSPECIFIED.,.F.,.F.,.F.)
B_SPLINE_SURFACE_WITH_KNOTS((4,2,2,2,4),(3,3),(0.000346079680846979,0.000742789375765937,
0.0011394990706849,0.00153620876560385,0.00193291846052281),(0.,1.),
 .UNSPECIFIED.)
GEOMETRIC_REPRESENTATION_ITEM()
RATIONAL_B_SPLINE_SURFACE(((1.,0.707106781186546,1.),(1.,0.716758952028333,
1.),(1.,0.727288011548303,1.),(1.,0.748184897297863,1.),(1.,0.758437122288391,
1.),(1.,0.776285930137885,1.),(1.,0.783895918656293,1.),(1.,0.79427968827415,
1.),(1.,0.797152913684263,1.),(1.,0.797116436093329,1.)))
REPRESENTATION_ITEM('')
SURFACE()
);
#1625=(
BOUNDED_SURFACE()
B_SPLINE_SURFACE(3,2,((#91047,#91048,#91049),(#91050,#91051,#91052),(#91053,
#91054,#91055),(#91056,#91057,#91058),(#91059,#91060,#91061),(#91062,#91063,
#91064),(#91065,#91066,#91067),(#91068,#91069,#91070),(#91071,#91072,#91073),
(#91074,#91075,#91076)),.UNSPECIFIED.,.F.,.F.,.F.)
B_SPLINE_SURFACE_WITH_KNOTS((4,2,2,2,4),(3,3),(0.000652435349851691,0.00105161226574612,
0.00145078918164054,0.00184996609753497,0.00224914301342939),(0.,1.),
 .UNSPECIFIED.)
GEOMETRIC_REPRESENTATION_ITEM()
RATIONAL_B_SPLINE_SURFACE(((1.,0.797116436093322,1.),(1.,0.79713399168744,
1.),(1.,0.794952627585016,1.),(1.,0.786540751799761,1.),(1.,0.780263959283671,
1.),(1.,0.764334803592261,1.),(1.,0.754537231253279,1.),(1.,0.732524301680786,
1.),(1.,0.720028936379745,1.),(1.,0.707106781186564,1.)))
REPRESENTATION_ITEM('')
SURFACE()
);
#1626=(
BOUNDED_SURFACE()
B_SPLINE_SURFACE(3,2,((#91122,#91123,#91124),(#91125,#91126,#91127),(#91128,
#91129,#91130),(#91131,#91132,#91133),(#91134,#91135,#91136),(#91137,#91138,
#91139),(#91140,#91141,#91142),(#91143,#91144,#91145),(#91146,#91147,#91148),
(#91149,#91150,#91151)),.UNSPECIFIED.,.F.,.F.,.F.)
B_SPLINE_SURFACE_WITH_KNOTS((4,2,2,2,4),(3,3),(0.000364014256986725,0.000763079051988796,
0.00116214384699087,0.00156120864199294,0.00196027343699501),(0.,1.),
 .UNSPECIFIED.)
GEOMETRIC_REPRESENTATION_ITEM()
RATIONAL_B_SPLINE_SURFACE(((1.,0.707106781186567,1.),(1.,0.720184284287246,
1.),(1.,0.732483148112649,1.),(1.,0.754654774294764,1.),(1.,0.76434671651307,
1.),(1.,0.780321857767699,1.),(1.,0.786575289610259,1.),(1.,0.79494789901223,
1.),(1.,0.797127700950757,1.),(1.,0.797116436093331,1.)))
REPRESENTATION_ITEM('')
SURFACE()
);
#1627=(
BOUNDED_SURFACE()
B_SPLINE_SURFACE(2,2,((#91239,#91240,#91241),(#91242,#91243,#91244),(#91245,
#91246,#91247)),.UNSPECIFIED.,.F.,.F.,.F.)
B_SPLINE_SURFACE_WITH_KNOTS((3,3),(3,3),(-1.11976951499864,0.),(0.,1.5707963267949),
 .UNSPECIFIED.)
GEOMETRIC_REPRESENTATION_ITEM()
RATIONAL_B_SPLINE_SURFACE(((1.,0.707106781186548,1.),(0.847316320613008,
0.599143116115493,0.847316320613008),(1.,0.707106781186548,1.)))
REPRESENTATION_ITEM('')
SURFACE()
);
#1628=(
BOUNDED_SURFACE()
B_SPLINE_SURFACE(3,2,((#91251,#91252,#91253),(#91254,#91255,#91256),(#91257,
#91258,#91259),(#91260,#91261,#91262),(#91263,#91264,#91265),(#91266,#91267,
#91268),(#91269,#91270,#91271),(#91272,#91273,#91274),(#91275,#91276,#91277),
(#91278,#91279,#91280),(#91281,#91282,#91283),(#91284,#91285,#91286),(#91287,
#91288,#91289),(#91290,#91291,#91292),(#91293,#91294,#91295),(#91296,#91297,
#91298),(#91299,#91300,#91301),(#91302,#91303,#91304),(#91305,#91306,#91307),
(#91308,#91309,#91310),(#91311,#91312,#91313),(#91314,#91315,#91316),(#91317,
#91318,#91319),(#91320,#91321,#91322),(#91323,#91324,#91325),(#91326,#91327,
#91328),(#91329,#91330,#91331),(#91332,#91333,#91334),(#91335,#91336,#91337),
(#91338,#91339,#91340),(#91341,#91342,#91343),(#91344,#91345,#91346),(#91347,
#91348,#91349),(#91350,#91351,#91352),(#91353,#91354,#91355),(#91356,#91357,
#91358),(#91359,#91360,#91361),(#91362,#91363,#91364),(#91365,#91366,#91367),
(#91368,#91369,#91370),(#91371,#91372,#91373),(#91374,#91375,#91376),(#91377,
#91378,#91379),(#91380,#91381,#91382),(#91383,#91384,#91385),(#91386,#91387,
#91388)),.UNSPECIFIED.,.F.,.F.,.F.)
B_SPLINE_SURFACE_WITH_KNOTS((4,2,2,2,2,2,2,2,2,2,2,2,2,2,2,2,2,2,2,2,2,
2,4),(3,3),(-0.000517275538890252,0.0157285769420072,0.0235928654130109,
0.0314571538840145,0.0393214423550181,0.0471857308260217,0.0550500192970254,
0.0570160914147763,0.0589821635325272,0.062914307768029,0.0707785962390326,
0.0727446683567835,0.0747107404745344,0.0786428847100362,0.082575028945538,
0.0845411010632889,0.0865071731810398,0.0943714616520435,0.102235750123047,
0.106167894358549,0.110100038594051,0.117964327065054,0.126345891074948),
(0.295770222528606,1.),.UNSPECIFIED.)
GEOMETRIC_REPRESENTATION_ITEM()
RATIONAL_B_SPLINE_SURFACE(((0.877986426924503,0.793735873692126,1.),(0.877986426924503,
0.793735873692126,1.),(0.877986426924503,0.793735873692126,1.),(0.877986426924503,
0.793735873692126,1.),(0.877986426924503,0.793735873692126,1.),(0.877986426924503,
0.793735873692126,1.),(0.877986426924503,0.793735873692126,1.),(0.877986426924503,
0.793735873692126,1.),(0.877986426924505,0.793735873692129,1.),(0.877986426924505,
0.793735873692129,1.),(0.877986426924511,0.793735873692139,1.),(0.877986426924511,
0.793735873692139,1.),(0.877986426924503,0.793735873692126,1.),(0.877986426924503,
0.793735873692126,1.),(0.877986426924503,0.793735873692126,1.),(0.877986426924503,
0.793735873692126,1.),(0.877986426924503,0.793735873692126,1.),(0.877986426924503,
0.793735873692126,1.),(0.877986426924503,0.793735873692126,1.),(0.877986426924503,
0.793735873692126,1.),(0.877986426924503,0.793735873692126,1.),(0.877986426924503,
0.793735873692126,1.),(0.877986426924492,0.793735873692107,1.),(0.877986426924492,
0.793735873692107,1.),(0.877986426924499,0.793735873692119,1.),(0.877986426924499,
0.793735873692119,1.),(0.877986426924505,0.793735873692129,1.),(0.877986426924505,
0.793735873692129,1.),(0.877986426924504,0.793735873692127,1.),(0.877986426924504,
0.793735873692127,1.),(0.877986426924488,0.793735873692099,1.),(0.877986426924488,
0.793735873692099,1.),(0.877986426924506,0.79373587369213,1.),(0.877986426924506,
0.79373587369213,1.),(0.877986426924503,0.793735873692126,1.),(0.877986426924503,
0.793735873692126,1.),(0.877986426924499,0.793735873692119,1.),(0.877986426924499,
0.793735873692119,1.),(0.877986426924503,0.793735873692126,1.),(0.877986426924503,
0.793735873692126,1.),(0.877986426924507,0.793735873692132,1.),(0.877986426924507,
0.793735873692132,1.),(0.877986426924503,0.793735873692126,1.),(0.877986426924503,
0.793735873692126,1.),(0.877986426924498,0.793735873692118,1.),(0.877986426924499,
0.793735873692119,1.)))
REPRESENTATION_ITEM('')
SURFACE()
);
#1629=(
BOUNDED_SURFACE()
B_SPLINE_SURFACE(3,2,((#91399,#91400,#91401),(#91402,#91403,#91404),(#91405,
#91406,#91407),(#91408,#91409,#91410),(#91411,#91412,#91413),(#91414,#91415,
#91416)),.UNSPECIFIED.,.F.,.F.,.F.)
B_SPLINE_SURFACE_WITH_KNOTS((4,2,4),(3,3),(0.,0.00187370917737372,0.00374741835474743),
(0.,0.715643358171679),.UNSPECIFIED.)
GEOMETRIC_REPRESENTATION_ITEM()
RATIONAL_B_SPLINE_SURFACE(((1.,0.868676996939189,0.925314863709635),(1.,
0.862154096139035,0.921605203376613),(1.,0.852620844137825,0.916183516327079),
(1.,0.826855889165617,0.901530644181569),(1.,0.81063530623189,0.892305783198504),
(1.,0.790392913302621,0.880793665446632)))
REPRESENTATION_ITEM('')
SURFACE()
);
#1630=(
BOUNDED_SURFACE()
B_SPLINE_SURFACE(2,2,((#91432,#91433,#91434),(#91435,#91436,#91437),(#91438,
#91439,#91440)),.UNSPECIFIED.,.F.,.F.,.F.)
B_SPLINE_SURFACE_WITH_KNOTS((3,3),(3,3),(-1.11976951499864,0.),(-1.5707963267949,
0.),.UNSPECIFIED.)
GEOMETRIC_REPRESENTATION_ITEM()
RATIONAL_B_SPLINE_SURFACE(((1.,0.707106781186548,1.),(0.847316320613008,
0.599143116115493,0.847316320613008),(1.,0.707106781186548,1.)))
REPRESENTATION_ITEM('')
SURFACE()
);
#1631=(
BOUNDED_SURFACE()
B_SPLINE_SURFACE(3,2,((#91444,#91445,#91446),(#91447,#91448,#91449),(#91450,
#91451,#91452),(#91453,#91454,#91455),(#91456,#91457,#91458),(#91459,#91460,
#91461)),.UNSPECIFIED.,.F.,.F.,.F.)
B_SPLINE_SURFACE_WITH_KNOTS((4,2,4),(3,3),(0.,0.00204073705610436,0.00408147411220872),
(0.,0.735738848586875),.UNSPECIFIED.)
GEOMETRIC_REPRESENTATION_ITEM()
RATIONAL_B_SPLINE_SURFACE(((1.,0.864989405740761,0.928643889816166),(1.,
0.872322079329199,0.932519371347001),(1.,0.875877893683041,0.934398698537716),
(1.,0.875878347808356,0.934398938553073),(1.,0.872319864193714,0.932518200598494),
(1.,0.864989405740073,0.928643889815803)))
REPRESENTATION_ITEM('')
SURFACE()
);
#1632=(
BOUNDED_SURFACE()
B_SPLINE_SURFACE(3,2,((#91474,#91475,#91476),(#91477,#91478,#91479),(#91480,
#91481,#91482),(#91483,#91484,#91485),(#91486,#91487,#91488),(#91489,#91490,
#91491)),.UNSPECIFIED.,.F.,.F.,.F.)
B_SPLINE_SURFACE_WITH_KNOTS((4,2,4),(3,3),(-4.33680868994202E-19,0.00187190510061502,
0.00374381020123004),(0.,0.715644139044445),.UNSPECIFIED.)
GEOMETRIC_REPRESENTATION_ITEM()
RATIONAL_B_SPLINE_SURFACE(((1.,0.790392684589732,0.880793862727862),(1.,
0.810642558292627,0.892310203269917),(1.,0.826863334737431,0.901535148972577),
(1.,0.852626485765744,0.916186954955745),(1.,0.862156703884265,0.921606901712117),
(1.,0.86867685364703,0.925314987310818)))
REPRESENTATION_ITEM('')
SURFACE()
);
#1633=(
BOUNDED_SURFACE()
B_SPLINE_SURFACE(3,2,((#91511,#91512,#91513),(#91514,#91515,#91516),(#91517,
#91518,#91519),(#91520,#91521,#91522),(#91523,#91524,#91525),(#91526,#91527,
#91528),(#91529,#91530,#91531),(#91532,#91533,#91534),(#91535,#91536,#91537),
(#91538,#91539,#91540),(#91541,#91542,#91543),(#91544,#91545,#91546),(#91547,
#91548,#91549),(#91550,#91551,#91552)),.UNSPECIFIED.,.F.,.F.,.F.)
B_SPLINE_SURFACE_WITH_KNOTS((4,2,2,2,2,2,4),(3,3),(-9.89281647458895E-5,
0.0149256238360901,0.0298512476721802,0.0447768715082703,0.0597024953443604,
0.0895537430165406,0.119503918899356),(0.296188569857101,1.),
 .UNSPECIFIED.)
GEOMETRIC_REPRESENTATION_ITEM()
RATIONAL_B_SPLINE_SURFACE(((0.877886431452041,0.793858404787744,1.),(0.877886431452041,
0.793858404787744,1.),(0.877886431452049,0.793858404787757,1.),(0.877886431452049,
0.793858404787757,1.),(0.877886431452045,0.79385840478775,1.),(0.877886431452045,
0.79385840478775,1.),(0.877886431452041,0.793858404787744,1.),(0.877886431452041,
0.793858404787744,1.),(0.877886431452041,0.793858404787744,1.),(0.877886431452041,
0.793858404787744,1.),(0.877886431452037,0.793858404787737,1.),(0.877886431452037,
0.793858404787737,1.),(0.877886431452041,0.793858404787744,1.),(0.877886431452041,
0.793858404787744,1.)))
REPRESENTATION_ITEM('')
SURFACE()
);
#1634=(
BOUNDED_SURFACE()
B_SPLINE_SURFACE(3,2,((#91583,#91584,#91585),(#91586,#91587,#91588),(#91589,
#91590,#91591),(#91592,#91593,#91594),(#91595,#91596,#91597),(#91598,#91599,
#91600),(#91601,#91602,#91603),(#91604,#91605,#91606),(#91607,#91608,#91609),
(#91610,#91611,#91612),(#91613,#91614,#91615),(#91616,#91617,#91618),(#91619,
#91620,#91621),(#91622,#91623,#91624),(#91625,#91626,#91627),(#91628,#91629,
#91630),(#91631,#91632,#91633),(#91634,#91635,#91636),(#91637,#91638,#91639),
(#91640,#91641,#91642),(#91643,#91644,#91645),(#91646,#91647,#91648),(#91649,
#91650,#91651),(#91652,#91653,#91654),(#91655,#91656,#91657),(#91658,#91659,
#91660),(#91661,#91662,#91663),(#91664,#91665,#91666),(#91667,#91668,#91669),
(#91670,#91671,#91672),(#91673,#91674,#91675),(#91676,#91677,#91678),(#91679,
#91680,#91681),(#91682,#91683,#91684),(#91685,#91686,#91687),(#91688,#91689,
#91690),(#91691,#91692,#91693),(#91694,#91695,#91696),(#91697,#91698,#91699),
(#91700,#91701,#91702),(#91703,#91704,#91705),(#91706,#91707,#91708),(#91709,
#91710,#91711),(#91712,#91713,#91714),(#91715,#91716,#91717),(#91718,#91719,
#91720),(#91721,#91722,#91723),(#91724,#91725,#91726),(#91727,#91728,#91729),
(#91730,#91731,#91732),(#91733,#91734,#91735),(#91736,#91737,#91738),(#91739,
#91740,#91741),(#91742,#91743,#91744),(#91745,#91746,#91747),(#91748,#91749,
#91750),(#91751,#91752,#91753),(#91754,#91755,#91756)),.UNSPECIFIED.,.F.,
 .F.,.F.)
B_SPLINE_SURFACE_WITH_KNOTS((4,2,2,2,2,2,2,2,2,2,2,2,2,2,2,2,2,2,2,2,2,
2,2,2,2,2,2,2,4),(3,3),(-0.000108339933889343,0.0321349777273597,0.0642699554547194,
0.0803374443183993,0.0964049331820792,0.112472422045759,0.128539910909439,
0.136573655341279,0.140590527557199,0.144607399773119,0.152641144204959,
0.156658016420879,0.160674888636799,0.168708633068639,0.172725505284558,
0.174733941392518,0.176742377500478,0.184776121932318,0.186784558040278,
0.188792994148238,0.192809866364158,0.200843610795998,0.204860483011918,
0.208877355227838,0.216911099659678,0.224944844091518,0.232978588523358,
0.241012332955198,0.257188161752767),(0.296179158133916,1.),
 .UNSPECIFIED.)
GEOMETRIC_REPRESENTATION_ITEM()
RATIONAL_B_SPLINE_SURFACE(((0.877888678834658,0.793855648157845,1.),(0.877888678834658,
0.793855648157845,1.),(0.877888678834658,0.793855648157845,1.),(0.877888678834658,
0.793855648157845,1.),(0.877888678834658,0.793855648157845,1.),(0.877888678834658,
0.793855648157845,1.),(0.877888678834658,0.793855648157845,1.),(0.877888678834658,
0.793855648157845,1.),(0.877888678834658,0.793855648157845,1.),(0.877888678834658,
0.793855648157845,1.),(0.877888678834658,0.793855648157846,1.),(0.877888678834658,
0.793855648157846,1.),(0.877888678834658,0.793855648157845,1.),(0.877888678834658,
0.793855648157845,1.),(0.877888678834649,0.793855648157832,1.),(0.877888678834649,
0.793855648157832,1.),(0.877888678834662,0.793855648157852,1.),(0.877888678834662,
0.793855648157852,1.),(0.87788867883467,0.793855648157866,1.),(0.87788867883467,
0.793855648157866,1.),(0.877888678834662,0.793855648157852,1.),(0.877888678834662,
0.793855648157852,1.),(0.877888678834658,0.793855648157845,1.),(0.877888678834658,
0.793855648157845,1.),(0.877888678834669,0.793855648157865,1.),(0.877888678834669,
0.793855648157865,1.),(0.877888678834662,0.793855648157852,1.),(0.877888678834662,
0.793855648157852,1.),(0.877888678834662,0.793855648157852,1.),(0.877888678834662,
0.793855648157852,1.),(0.877888678834667,0.793855648157861,1.),(0.877888678834667,
0.793855648157861,1.),(0.877888678834668,0.793855648157862,1.),(0.877888678834668,
0.793855648157862,1.),(0.877888678834658,0.793855648157845,1.),(0.877888678834658,
0.793855648157845,1.),(0.877888678834658,0.793855648157845,1.),(0.877888678834658,
0.793855648157845,1.),(0.877888678834658,0.793855648157845,1.),(0.877888678834658,
0.793855648157845,1.),(0.877888678834656,0.793855648157842,1.),(0.877888678834656,
0.793855648157842,1.),(0.877888678834663,0.793855648157855,1.),(0.877888678834663,
0.793855648157855,1.),(0.877888678834658,0.793855648157845,1.),(0.877888678834658,
0.793855648157845,1.),(0.877888678834662,0.793855648157852,1.),(0.877888678834662,
0.793855648157852,1.),(0.877888678834658,0.793855648157845,1.),(0.877888678834658,
0.793855648157845,1.),(0.877888678834662,0.793855648157852,1.),(0.877888678834662,
0.793855648157852,1.),(0.877888678834658,0.793855648157845,1.),(0.877888678834658,
0.793855648157845,1.),(0.877888678834664,0.793855648157856,1.),(0.877888678834664,
0.793855648157856,1.),(0.877888678834649,0.793855648157831,1.),(0.877888678834649,
0.793855648157831,1.)))
REPRESENTATION_ITEM('')
SURFACE()
);
#1635=(
BOUNDED_SURFACE()
B_SPLINE_SURFACE(3,2,((#91965,#91966,#91967),(#91968,#91969,#91970),(#91971,
#91972,#91973),(#91974,#91975,#91976),(#91977,#91978,#91979),(#91980,#91981,
#91982),(#91983,#91984,#91985),(#91986,#91987,#91988),(#91989,#91990,#91991),
(#91992,#91993,#91994),(#91995,#91996,#91997),(#91998,#91999,#92000),(#92001,
#92002,#92003),(#92004,#92005,#92006),(#92007,#92008,#92009),(#92010,#92011,
#92012),(#92013,#92014,#92015),(#92016,#92017,#92018),(#92019,#92020,#92021),
(#92022,#92023,#92024),(#92025,#92026,#92027),(#92028,#92029,#92030),(#92031,
#92032,#92033),(#92034,#92035,#92036),(#92037,#92038,#92039),(#92040,#92041,
#92042),(#92043,#92044,#92045),(#92046,#92047,#92048),(#92049,#92050,#92051),
(#92052,#92053,#92054),(#92055,#92056,#92057),(#92058,#92059,#92060),(#92061,
#92062,#92063),(#92064,#92065,#92066),(#92067,#92068,#92069),(#92070,#92071,
#92072),(#92073,#92074,#92075),(#92076,#92077,#92078),(#92079,#92080,#92081),
(#92082,#92083,#92084),(#92085,#92086,#92087),(#92088,#92089,#92090)),
 .UNSPECIFIED.,.F.,.F.,.F.)
B_SPLINE_SURFACE_WITH_KNOTS((4,2,2,2,2,2,2,2,2,2,2,2,2,2,2,2,2,2,2,2,4),
(3,3),(0.,0.0265419162547455,0.053083832509491,0.0796257487642365,0.0928967068916092,
0.106167665018982,0.119438623146355,0.132709581273727,0.139345060337414,
0.1459805394011,0.159251497528473,0.165886976592159,0.172522455655846,0.179157934719532,
0.185793413783218,0.189111153315062,0.192428892846905,0.199064371910591,
0.205699850974278,0.209017590506121,0.212335330037964),(0.,1.),
 .UNSPECIFIED.)
GEOMETRIC_REPRESENTATION_ITEM()
RATIONAL_B_SPLINE_SURFACE(((1.,0.707106781186547,1.),(1.,0.707106781186547,
1.),(1.,0.707106781186548,1.),(1.,0.707106781186548,1.),(1.,0.707106781186548,
1.),(1.,0.707106781186548,1.),(1.,0.707106781186543,1.),(1.,0.707106781186543,
1.),(1.,0.707106781186552,1.),(1.,0.707106781186552,1.),(1.,0.707106781186548,
1.),(1.,0.707106781186548,1.),(1.,0.707106781186548,1.),(1.,0.707106781186548,
1.),(1.,0.707106781186547,1.),(1.,0.707106781186547,1.),(1.,0.707106781186543,
1.),(1.,0.707106781186543,1.),(1.,0.707106781186548,1.),(1.,0.707106781186548,
1.),(1.,0.707106781186552,1.),(1.,0.707106781186552,1.),(1.,0.707106781186543,
1.),(1.,0.707106781186543,1.),(1.,0.707106781186547,1.),(1.,0.707106781186547,
1.),(1.,0.707106781186548,1.),(1.,0.707106781186548,1.),(1.,0.707106781186531,
1.),(1.,0.707106781186531,1.),(1.,0.707106781186543,1.),(1.,0.707106781186543,
1.),(1.,0.707106781186557,1.),(1.,0.707106781186557,1.),(1.,0.707106781186538,
1.),(1.,0.707106781186538,1.),(1.,0.707106781186548,1.),(1.,0.707106781186548,
1.),(1.,0.707106781186557,1.),(1.,0.707106781186557,1.),(1.,0.707106781186548,
1.),(1.,0.707106781186548,1.)))
REPRESENTATION_ITEM('')
SURFACE()
);
#1636=(
BOUNDED_SURFACE()
B_SPLINE_SURFACE(3,2,((#92408,#92409,#92410),(#92411,#92412,#92413),(#92414,
#92415,#92416),(#92417,#92418,#92419),(#92420,#92421,#92422),(#92423,#92424,
#92425),(#92426,#92427,#92428),(#92429,#92430,#92431),(#92432,#92433,#92434),
(#92435,#92436,#92437),(#92438,#92439,#92440),(#92441,#92442,#92443)),
 .UNSPECIFIED.,.F.,.F.,.F.)
B_SPLINE_SURFACE_WITH_KNOTS((4,2,2,2,2,4),(3,3),(0.,0.0276588530591966,
0.0553177061183932,0.0829765591775898,0.0968059857071881,0.110635412236786),
(0.,1.),.UNSPECIFIED.)
GEOMETRIC_REPRESENTATION_ITEM()
RATIONAL_B_SPLINE_SURFACE(((1.,0.707106781186547,1.),(1.,0.707106781186547,
1.),(1.,0.707106781186553,1.),(1.,0.707106781186553,1.),(1.,0.707106781186543,
1.),(1.,0.707106781186543,1.),(1.,0.707106781186548,1.),(1.,0.707106781186548,
1.),(1.,0.707106781186543,1.),(1.,0.707106781186543,1.),(1.,0.707106781186543,
1.),(1.,0.707106781186543,1.)))
REPRESENTATION_ITEM('')
SURFACE()
);
#1637=(
BOUNDED_SURFACE()
B_SPLINE_SURFACE(3,2,((#92543,#92544,#92545),(#92546,#92547,#92548),(#92549,
#92550,#92551),(#92552,#92553,#92554),(#92555,#92556,#92557),(#92558,#92559,
#92560),(#92561,#92562,#92563),(#92564,#92565,#92566),(#92567,#92568,#92569),
(#92570,#92571,#92572),(#92573,#92574,#92575),(#92576,#92577,#92578),(#92579,
#92580,#92581),(#92582,#92583,#92584)),.UNSPECIFIED.,.F.,.F.,.F.)
B_SPLINE_SURFACE_WITH_KNOTS((4,2,2,2,2,2,4),(3,3),(-2.75387351811318E-17,
0.000503019152578121,0.00100603830515627,0.00150905745773442,0.00201207661031257,
0.00301811491546887,0.00402415322062516),(0.,1.),.UNSPECIFIED.)
GEOMETRIC_REPRESENTATION_ITEM()
RATIONAL_B_SPLINE_SURFACE(((1.,0.947539216237274,1.),(1.,0.947529154337319,
1.),(1.,0.945092080349251,1.),(1.,0.936003138514207,1.),(1.,0.92961504518381,
1.),(1.,0.914166261177696,1.),(1.,0.905357494770243,1.),(1.,0.8860141198597,
1.),(1.,0.875396745378908,1.),(1.,0.842143074103383,1.),(1.,0.817763975573635,
1.),(1.,0.764845303360259,1.),(1.,0.736920996311044,1.),(1.,0.707106781186552,
1.)))
REPRESENTATION_ITEM('')
SURFACE()
);
#1638=(
BOUNDED_SURFACE()
B_SPLINE_SURFACE(3,2,((#92663,#92664,#92665),(#92666,#92667,#92668),(#92669,
#92670,#92671),(#92672,#92673,#92674),(#92675,#92676,#92677),(#92678,#92679,
#92680),(#92681,#92682,#92683),(#92684,#92685,#92686),(#92687,#92688,#92689),
(#92690,#92691,#92692),(#92693,#92694,#92695),(#92696,#92697,#92698),(#92699,
#92700,#92701),(#92702,#92703,#92704),(#92705,#92706,#92707),(#92708,#92709,
#92710),(#92711,#92712,#92713),(#92714,#92715,#92716),(#92717,#92718,#92719),
(#92720,#92721,#92722),(#92723,#92724,#92725),(#92726,#92727,#92728),(#92729,
#92730,#92731),(#92732,#92733,#92734),(#92735,#92736,#92737),(#92738,#92739,
#92740),(#92741,#92742,#92743),(#92744,#92745,#92746)),.UNSPECIFIED.,.F.,
 .F.,.F.)
B_SPLINE_SURFACE_WITH_KNOTS((4,2,2,2,2,2,2,2,2,2,2,2,2,4),(3,3),(0.,0.00784373710475995,
0.0117656056571399,0.0137265399333299,0.0156874742095199,0.0235312113142798,
0.0254921455904698,0.0274530798666598,0.0313749484190398,0.0392186855237997,
0.0431405540761797,0.0470624226285597,0.0549061597333196,0.0627498968380796),
(0.,1.),.UNSPECIFIED.)
GEOMETRIC_REPRESENTATION_ITEM()
RATIONAL_B_SPLINE_SURFACE(((1.,0.707106781186548,1.),(1.,0.707106781186548,
1.),(1.,0.707106781186548,1.),(1.,0.707106781186548,1.),(1.,0.707106781186548,
1.),(1.,0.707106781186548,1.),(1.,0.707106781186548,1.),(1.,0.707106781186548,
1.),(1.,0.707106781186539,1.),(1.,0.707106781186539,1.),(1.,0.707106781186558,
1.),(1.,0.707106781186558,1.),(1.,0.707106781186545,1.),(1.,0.707106781186545,
1.),(1.,0.70710678118655,1.),(1.,0.70710678118655,1.),(1.,0.707106781186557,
1.),(1.,0.707106781186557,1.),(1.,0.707106781186552,1.),(1.,0.707106781186552,
1.),(1.,0.707106781186543,1.),(1.,0.707106781186543,1.),(1.,0.707106781186538,
1.),(1.,0.707106781186538,1.),(1.,0.707106781186552,1.),(1.,0.707106781186552,
1.),(1.,0.707106781186552,1.),(1.,0.707106781186552,1.)))
REPRESENTATION_ITEM('')
SURFACE()
);
#1639=(
BOUNDED_SURFACE()
B_SPLINE_SURFACE(3,2,((#92883,#92884,#92885),(#92886,#92887,#92888),(#92889,
#92890,#92891),(#92892,#92893,#92894),(#92895,#92896,#92897),(#92898,#92899,
#92900),(#92901,#92902,#92903),(#92904,#92905,#92906),(#92907,#92908,#92909),
(#92910,#92911,#92912),(#92913,#92914,#92915),(#92916,#92917,#92918)),
 .UNSPECIFIED.,.F.,.F.,.F.)
B_SPLINE_SURFACE_WITH_KNOTS((4,2,2,2,2,4),(3,3),(-1.51788304147971E-17,
0.001026154090376,0.00205230818075201,0.00307846227112803,0.00359153931631603,
0.00410461636150404),(0.,1.),.UNSPECIFIED.)
GEOMETRIC_REPRESENTATION_ITEM()
RATIONAL_B_SPLINE_SURFACE(((1.,0.707106781186551,1.),(1.,0.737458539324085,
1.),(1.,0.765604818101815,1.),(1.,0.818578626740854,1.),(1.,0.843670764069377,
1.),(1.,0.88861714259258,1.),(1.,0.909068963683481,1.),(1.,0.932796796200486,
1.),(1.,0.939529068116547,1.),(1.,0.948990840857779,1.),(1.,0.951717595991349,
1.),(1.,0.951672260128341,1.)))
REPRESENTATION_ITEM('')
SURFACE()
);
#1640=(
BOUNDED_SURFACE()
B_SPLINE_SURFACE(3,2,((#93010,#93011,#93012),(#93013,#93014,#93015),(#93016,
#93017,#93018),(#93019,#93020,#93021),(#93022,#93023,#93024),(#93025,#93026,
#93027),(#93028,#93029,#93030),(#93031,#93032,#93033),(#93034,#93035,#93036),
(#93037,#93038,#93039),(#93040,#93041,#93042),(#93043,#93044,#93045),(#93046,
#93047,#93048),(#93049,#93050,#93051)),.UNSPECIFIED.,.F.,.F.,.F.)
B_SPLINE_SURFACE_WITH_KNOTS((4,2,2,2,2,2,4),(3,3),(-8.43509290193722E-17,
0.000727263540504352,0.00109089531075657,0.00145452708100879,0.00181815885126101,
0.00218179062151323,0.00290905416201766),(0.,1.),.UNSPECIFIED.)
GEOMETRIC_REPRESENTATION_ITEM()
RATIONAL_B_SPLINE_SURFACE(((1.,0.725721029069481,1.),(1.,0.724034693474907,
1.),(1.,0.721379296500622,1.),(1.,0.716422727384689,1.),(1.,0.714644097901878,
1.),(1.,0.710947104597259,1.),(1.,0.709008369219941,1.),(1.,0.705233944978655,
1.),(1.,0.703402722400818,1.),(1.,0.699997845626205,1.),(1.,0.698413596841744,
1.),(1.,0.694441904737375,1.),(1.,0.692773088959507,1.),(1.,0.69256010548478,
1.)))
REPRESENTATION_ITEM('')
SURFACE()
);
#1641=(
BOUNDED_SURFACE()
B_SPLINE_SURFACE(3,2,((#93095,#93096,#93097),(#93098,#93099,#93100),(#93101,
#93102,#93103),(#93104,#93105,#93106)),.UNSPECIFIED.,.F.,.F.,.F.)
B_SPLINE_SURFACE_WITH_KNOTS((4,4),(3,3),(-2.84494650060196E-16,0.00346720850760631),
(0.,1.),.UNSPECIFIED.)
GEOMETRIC_REPRESENTATION_ITEM()
RATIONAL_B_SPLINE_SURFACE(((1.,0.69256010548478,1.),(1.,0.692352515709661,
1.),(1.,0.693728033206585,1.),(1.,0.696613144076467,1.)))
REPRESENTATION_ITEM('')
SURFACE()
);
#1642=(
BOUNDED_SURFACE()
B_SPLINE_SURFACE(3,2,((#93116,#93117,#93118),(#93119,#93120,#93121),(#93122,
#93123,#93124),(#93125,#93126,#93127),(#93128,#93129,#93130),(#93131,#93132,
#93133),(#93134,#93135,#93136),(#93137,#93138,#93139)),.UNSPECIFIED.,.F.,
 .F.,.F.)
B_SPLINE_SURFACE_WITH_KNOTS((4,2,2,4),(3,3),(-2.56413813792822E-15,0.00117043131394467,
0.00175564697091828,0.0023408626278919),(0.,1.),.UNSPECIFIED.)
GEOMETRIC_REPRESENTATION_ITEM()
RATIONAL_B_SPLINE_SURFACE(((1.,0.829660876349343,1.),(1.,0.821608938591335,
1.),(1.,0.808805545265545,1.),(1.,0.782695994949833,1.),(1.,0.772729068233022,
1.),(1.,0.750888902265591,1.),(1.,0.738815967034684,1.),(1.,0.725721029069557,
1.)))
REPRESENTATION_ITEM('')
SURFACE()
);
#1643=(
BOUNDED_SURFACE()
B_SPLINE_SURFACE(3,2,((#93182,#93183,#93184),(#93185,#93186,#93187),(#93188,
#93189,#93190),(#93191,#93192,#93193),(#93194,#93195,#93196),(#93197,#93198,
#93199),(#93200,#93201,#93202),(#93203,#93204,#93205),(#93206,#93207,#93208),
(#93209,#93210,#93211),(#93212,#93213,#93214),(#93215,#93216,#93217),(#93218,
#93219,#93220),(#93221,#93222,#93223),(#93224,#93225,#93226),(#93227,#93228,
#93229),(#93230,#93231,#93232),(#93233,#93234,#93235),(#93236,#93237,#93238),
(#93239,#93240,#93241),(#93242,#93243,#93244),(#93245,#93246,#93247),(#93248,
#93249,#93250),(#93251,#93252,#93253),(#93254,#93255,#93256),(#93257,#93258,
#93259),(#93260,#93261,#93262),(#93263,#93264,#93265),(#93266,#93267,#93268),
(#93269,#93270,#93271)),.UNSPECIFIED.,.F.,.F.,.F.)
B_SPLINE_SURFACE_WITH_KNOTS((4,2,2,2,2,2,2,2,2,2,2,2,2,2,4),(3,3),(-2.39565312032397E-15,
0.00505776268902388,0.00758664403353702,0.0101155253780502,0.0151732880670764,
0.0177021694115896,0.0189666100838462,0.0202310507561027,0.025288813445129,
0.0278176947896421,0.0290821354618987,0.0303465761341553,0.0354043388231816,
0.0379332201676947,0.0404621015122078),(0.,1.),.UNSPECIFIED.)
GEOMETRIC_REPRESENTATION_ITEM()
RATIONAL_B_SPLINE_SURFACE(((1.,0.696613144076472,1.),(1.,0.696599130026136,
1.),(1.,0.696575727272268,1.),(1.,0.696538360390545,1.),(1.,0.696525560572403,
1.),(1.,0.696502310365975,1.),(1.,0.696491830261394,1.),(1.,0.696470340381519,
1.),(1.,0.696468946397757,1.),(1.,0.696519595395987,1.),(1.,0.696545414772987,
1.),(1.,0.696603616414338,1.),(1.,0.696626278754734,1.),(1.,0.696679373029936,
1.),(1.,0.696709897027162,1.),(1.,0.69688419627133,1.),(1.,0.697091091364156,
1.),(1.,0.697570485772635,1.),(1.,0.697758737895884,1.),(1.,0.698095724987984,
1.),(1.,0.698217184521284,1.),(1.,0.698480760086518,1.),(1.,0.698623206103489,
1.),(1.,0.699386462708979,1.),(1.,0.700161541053975,1.),(1.,0.701679166289421,
1.),(1.,0.702244592832563,1.),(1.,0.703518483373878,1.),(1.,0.704229250046039,
1.),(1.,0.705017710605485,1.)))
REPRESENTATION_ITEM('')
SURFACE()
);
#1644=(
BOUNDED_SURFACE()
B_SPLINE_SURFACE(3,2,((#93358,#93359,#93360),(#93361,#93362,#93363),(#93364,
#93365,#93366),(#93367,#93368,#93369),(#93370,#93371,#93372),(#93373,#93374,
#93375),(#93376,#93377,#93378),(#93379,#93380,#93381),(#93382,#93383,#93384),
(#93385,#93386,#93387),(#93388,#93389,#93390),(#93391,#93392,#93393)),
 .UNSPECIFIED.,.F.,.F.,.F.)
B_SPLINE_SURFACE_WITH_KNOTS((4,2,2,2,2,4),(3,3),(0.,0.00381964231177775,
0.0076392846235555,0.00954910577944438,0.0114589269353332,0.015278569247111),
(0.,1.),.UNSPECIFIED.)
GEOMETRIC_REPRESENTATION_ITEM()
RATIONAL_B_SPLINE_SURFACE(((1.,0.781244946784369,1.),(1.,0.781562440256923,
1.),(1.,0.783026424270278,1.),(1.,0.787952903484347,1.),(1.,0.791415097203598,
1.),(1.,0.797906633970797,1.),(1.,0.800295219844003,1.),(1.,0.805396324076371,
1.),(1.,0.808114271065591,1.),(1.,0.816694595542238,1.),(1.,0.822982727529132,
1.),(1.,0.829660876349356,1.)))
REPRESENTATION_ITEM('')
SURFACE()
);
#1645=(
BOUNDED_SURFACE()
B_SPLINE_SURFACE(3,2,((#93427,#93428,#93429),(#93430,#93431,#93432),(#93433,
#93434,#93435),(#93436,#93437,#93438),(#93439,#93440,#93441),(#93442,#93443,
#93444)),.UNSPECIFIED.,.F.,.F.,.F.)
B_SPLINE_SURFACE_WITH_KNOTS((4,2,4),(3,3),(0.00622093395683224,0.00836137417484186,
0.0105018143928515),(0.215795545199942,1.),.UNSPECIFIED.)
GEOMETRIC_REPRESENTATION_ITEM()
RATIONAL_B_SPLINE_SURFACE(((0.900161575810827,0.768673574571085,1.),(0.906212716749595,
0.782694116406556,1.),(0.909226759580194,0.789677677693251,1.),(0.909711211930778,
0.790800157654861,1.),(0.907180359960508,0.784936153446793,1.),(0.901691029052784,
0.772217329935776,1.)))
REPRESENTATION_ITEM('')
SURFACE()
);
#1646=(
BOUNDED_SURFACE()
B_SPLINE_SURFACE(3,2,((#93446,#93447,#93448),(#93449,#93450,#93451),(#93452,
#93453,#93454),(#93455,#93456,#93457),(#93458,#93459,#93460),(#93461,#93462,
#93463),(#93464,#93465,#93466),(#93467,#93468,#93469),(#93470,#93471,#93472),
(#93473,#93474,#93475),(#93476,#93477,#93478),(#93479,#93480,#93481),(#93482,
#93483,#93484),(#93485,#93486,#93487),(#93488,#93489,#93490),(#93491,#93492,
#93493),(#93494,#93495,#93496),(#93497,#93498,#93499),(#93500,#93501,#93502),
(#93503,#93504,#93505),(#93506,#93507,#93508),(#93509,#93510,#93511),(#93512,
#93513,#93514),(#93515,#93516,#93517)),.UNSPECIFIED.,.F.,.F.,.F.)
B_SPLINE_SURFACE_WITH_KNOTS((4,2,2,2,2,2,2,2,2,2,2,4),(3,3),(0.044623233310389,
0.0484077487639251,0.0503000064906932,0.0521922642174613,0.0559767796709975,
0.0578690373977656,0.0597612951245336,0.0635458105780698,0.067330326031606,
0.0692225837583741,0.0711148414851421,0.0748993569386783),(0.,1.),
 .UNSPECIFIED.)
GEOMETRIC_REPRESENTATION_ITEM()
RATIONAL_B_SPLINE_SURFACE(((1.,0.709536628273658,1.),(1.,0.711112477964268,
1.),(1.,0.712886961021962,1.),(1.,0.715904125550345,1.),(1.,0.716973272082696,
1.),(1.,0.71921250292588,1.),(1.,0.720383423890183,1.),(1.,0.724054149508398,
1.),(1.,0.726712444737782,1.),(1.,0.731025306021556,1.),(1.,0.732517045915888,
1.),(1.,0.735608355478324,1.),(1.,0.737211774675347,1.),(1.,0.742154682346366,
1.),(1.,0.74559035921566,1.),(1.,0.752655465612555,1.),(1.,0.756285259234572,
1.),(1.,0.761780390504015,1.),(1.,0.76362016208338,1.),(1.,0.767295160021535,
1.),(1.,0.769124263260604,1.),(1.,0.774512328170999,1.),(1.,0.77798836077047,
1.),(1.,0.781244946784368,1.)))
REPRESENTATION_ITEM('')
SURFACE()
);
#1647=(
BOUNDED_SURFACE()
B_SPLINE_SURFACE(3,2,((#93592,#93593,#93594),(#93595,#93596,#93597),(#93598,
#93599,#93600),(#93601,#93602,#93603),(#93604,#93605,#93606),(#93607,#93608,
#93609),(#93610,#93611,#93612),(#93613,#93614,#93615),(#93616,#93617,#93618),
(#93619,#93620,#93621),(#93622,#93623,#93624),(#93625,#93626,#93627),(#93628,
#93629,#93630),(#93631,#93632,#93633),(#93634,#93635,#93636),(#93637,#93638,
#93639),(#93640,#93641,#93642),(#93643,#93644,#93645),(#93646,#93647,#93648),
(#93649,#93650,#93651),(#93652,#93653,#93654),(#93655,#93656,#93657),(#93658,
#93659,#93660),(#93661,#93662,#93663),(#93664,#93665,#93666),(#93667,#93668,
#93669),(#93670,#93671,#93672),(#93673,#93674,#93675),(#93676,#93677,#93678),
(#93679,#93680,#93681),(#93682,#93683,#93684),(#93685,#93686,#93687),(#93688,
#93689,#93690),(#93691,#93692,#93693),(#93694,#93695,#93696),(#93697,#93698,
#93699),(#93700,#93701,#93702),(#93703,#93704,#93705),(#93706,#93707,#93708),
(#93709,#93710,#93711),(#93712,#93713,#93714),(#93715,#93716,#93717),(#93718,
#93719,#93720),(#93721,#93722,#93723),(#93724,#93725,#93726),(#93727,#93728,
#93729),(#93730,#93731,#93732),(#93733,#93734,#93735),(#93736,#93737,#93738),
(#93739,#93740,#93741),(#93742,#93743,#93744),(#93745,#93746,#93747)),
 .UNSPECIFIED.,.F.,.F.,.F.)
B_SPLINE_SURFACE_WITH_KNOTS((4,2,2,2,2,2,2,2,2,2,2,2,2,2,2,2,2,2,2,2,2,
2,2,2,2,4),(3,3),(0.,0.0246541424270968,0.0493082848541936,0.0739624272812903,
0.0862894984948387,0.0986165697083871,0.110943640921935,0.123270712135484,
0.129434247742258,0.135597783349032,0.141761318955806,0.144843086759194,
0.147924854562581,0.154088390169355,0.160251925776129,0.163333693579516,
0.16487457748121,0.166415461382903,0.172578996989677,0.175660764793065,
0.178742532596452,0.184906068203226,0.187987836006613,0.189528719908306,
0.19106960381,0.197233139416774),(0.,1.),.UNSPECIFIED.)
GEOMETRIC_REPRESENTATION_ITEM()
RATIONAL_B_SPLINE_SURFACE(((1.,0.709074301978794,1.),(1.,0.709074301978794,
1.),(1.,0.708963390930669,1.),(1.,0.710109418369442,1.),(1.,0.711345435969898,
1.),(1.,0.716322609340493,1.),(1.,0.720058949582277,1.),(1.,0.72837691193742,
1.),(1.,0.731601440707376,1.),(1.,0.739089721988529,1.),(1.,0.743354004659929,
1.),(1.,0.753044180212456,1.),(1.,0.758471196283739,1.),(1.,0.770572077971438,
1.),(1.,0.777247974837517,1.),(1.,0.788198389680482,1.),(1.,0.792007762550323,
1.),(1.,0.79989916400913,1.),(1.,0.803980722224322,1.),(1.,0.812377434705544,
1.),(1.,0.816692624895053,1.),(1.,0.82329981820533,1.),(1.,0.825524485365509,
1.),(1.,0.830009997246824,1.),(1.,0.832273217353446,1.),(1.,0.839066413030268,
1.),(1.,0.843609213674719,1.),(1.,0.852620563957069,1.),(1.,0.857088966114341,
1.),(1.,0.863655694461054,1.),(1.,0.86582194782431,1.),(1.,0.869027054063668,
1.),(1.,0.8700880407856,1.),(1.,0.872193462935808,1.),(1.,0.873239200602622,
1.),(1.,0.878385612494048,1.),(1.,0.882266154343622,1.),(1.,0.887638176463745,
1.),(1.,0.889353780493633,1.),(1.,0.892609052853279,1.),(1.,0.894152648985923,
1.),(1.,0.898377291742568,1.),(1.,0.900580262495945,1.),(1.,0.903583189673952,
1.),(1.,0.904578419755403,1.),(1.,0.906308844732561,1.),(1.,0.90692493411477,
1.),(1.,0.908224668315115,1.),(1.,0.90890921926144,1.),(1.,0.912472172767833,
1.),(1.,0.915754136767764,1.),(1.,0.918929033017135,1.)))
REPRESENTATION_ITEM('')
SURFACE()
);
#1648=(
BOUNDED_SURFACE()
B_SPLINE_SURFACE(3,2,((#94143,#94144,#94145),(#94146,#94147,#94148),(#94149,
#94150,#94151),(#94152,#94153,#94154),(#94155,#94156,#94157),(#94158,#94159,
#94160),(#94161,#94162,#94163),(#94164,#94165,#94166),(#94167,#94168,#94169),
(#94170,#94171,#94172),(#94173,#94174,#94175),(#94176,#94177,#94178),(#94179,
#94180,#94181),(#94182,#94183,#94184)),.UNSPECIFIED.,.F.,.F.,.F.)
B_SPLINE_SURFACE_WITH_KNOTS((4,2,2,2,2,2,4),(3,3),(0.00157084992542587,
0.00258948856452903,0.00355026347239947,0.00403065092633469,0.00451103838026991,
0.00499142583420513,0.00552967701937307),(0.,1.00005786373123),
 .UNSPECIFIED.)
GEOMETRIC_REPRESENTATION_ITEM()
RATIONAL_B_SPLINE_SURFACE(((1.,0.704737095511617,1.0000341700267),(1.,0.736101336346774,
1.00003054032269),(1.,0.764731830804985,1.00002722698822),(1.,0.815971505611802,
1.00002129715068),(1.,0.839121073814733,1.00001861810989),(1.,0.868723144579927,
1.00001519233736),(1.,0.877891123385711,1.00001413135044),(1.,0.893882869863667,
1.00001228066619),(1.,0.900743560306276,1.0000114866959),(1.,0.911766049485974,
1.0000102110912),(1.,0.915689588589873,1.00000975702997),(1.,0.920335904299819,
1.00000921932364),(1.,0.920452978363282,1.00000920577496),(1.,0.918312342823876,
1.00000945350528)))
REPRESENTATION_ITEM('')
SURFACE()
);
#1649=(
BOUNDED_SURFACE()
B_SPLINE_SURFACE(3,2,((#94281,#94282,#94283),(#94284,#94285,#94286),(#94287,
#94288,#94289),(#94290,#94291,#94292),(#94293,#94294,#94295),(#94296,#94297,
#94298),(#94299,#94300,#94301),(#94302,#94303,#94304),(#94305,#94306,#94307),
(#94308,#94309,#94310),(#94311,#94312,#94313),(#94314,#94315,#94316)),
 .UNSPECIFIED.,.F.,.F.,.F.)
B_SPLINE_SURFACE_WITH_KNOTS((4,2,2,2,2,4),(3,3),(0.,0.0240998197753932,
0.0481996395507863,0.0722994593261795,0.0843493692138761,0.0963992791015727),
(0.,1.),.UNSPECIFIED.)
GEOMETRIC_REPRESENTATION_ITEM()
RATIONAL_B_SPLINE_SURFACE(((1.,0.709074301978794,1.),(1.,0.709074301978794,
1.),(1.,0.708967090641946,1.),(1.,0.710030391587723,1.),(1.,0.711181727679598,
1.),(1.,0.715829967728869,1.),(1.,0.719322261302017,1.),(1.,0.727098307859076,
1.),(1.,0.730113359209246,1.),(1.,0.737118658661219,1.),(1.,0.741109043083379,
1.),(1.,0.745647926668359,1.)))
REPRESENTATION_ITEM('')
SURFACE()
);
#1650=(
BOUNDED_SURFACE()
B_SPLINE_SURFACE(3,2,((#94357,#94358,#94359),(#94360,#94361,#94362),(#94363,
#94364,#94365),(#94366,#94367,#94368)),.UNSPECIFIED.,.F.,.F.,.F.)
B_SPLINE_SURFACE_WITH_KNOTS((4,4),(3,3),(0.,0.000852897709755378),(0.,1.),
 .UNSPECIFIED.)
GEOMETRIC_REPRESENTATION_ITEM()
RATIONAL_B_SPLINE_SURFACE(((1.,0.707106781186548,1.),(1.,0.708115545993389,
1.),(1.,0.709103409674823,1.),(1.,0.710072428249471,1.)))
REPRESENTATION_ITEM('')
SURFACE()
);
#1651=(
BOUNDED_SURFACE()
B_SPLINE_SURFACE(3,2,((#94374,#94375,#94376),(#94377,#94378,#94379),(#94380,
#94381,#94382),(#94383,#94384,#94385),(#94386,#94387,#94388),(#94389,#94390,
#94391),(#94392,#94393,#94394),(#94395,#94396,#94397),(#94398,#94399,#94400),
(#94401,#94402,#94403),(#94404,#94405,#94406),(#94407,#94408,#94409),(#94410,
#94411,#94412),(#94413,#94414,#94415),(#94416,#94417,#94418),(#94419,#94420,
#94421)),.UNSPECIFIED.,.F.,.F.,.F.)
B_SPLINE_SURFACE_WITH_KNOTS((4,2,2,2,2,2,2,4),(3,3),(0.00112108086692784,
0.00160664620305947,0.00209221153919109,0.00257777687532272,0.00306334221145435,
0.00354890754758597,0.0040344728837176,0.00500560355598086),(0.,1.),
 .UNSPECIFIED.)
GEOMETRIC_REPRESENTATION_ITEM()
RATIONAL_B_SPLINE_SURFACE(((1.,0.918929033017135,1.),(1.,0.920406077770156,
1.),(1.,0.92007472019659,1.),(1.,0.915695855491378,1.),(1.,0.911745925902294,
1.),(1.,0.900758581231695,1.),(1.,0.893857751485131,1.),(1.,0.877902801467609,
1.),(1.,0.868723355189685,1.),(1.,0.849021030588752,1.),(1.,0.838418680991936,
1.),(1.,0.815752189451713,1.),(1.,0.803660285004169,1.),(1.,0.766185207769967,
1.),(1.,0.739276146867789,1.),(1.,0.710072428249468,1.)))
REPRESENTATION_ITEM('')
SURFACE()
);
#1652=(
BOUNDED_SURFACE()
B_SPLINE_SURFACE(3,2,((#94571,#94572,#94573),(#94574,#94575,#94576),(#94577,
#94578,#94579),(#94580,#94581,#94582),(#94583,#94584,#94585),(#94586,#94587,
#94588),(#94589,#94590,#94591),(#94592,#94593,#94594),(#94595,#94596,#94597),
(#94598,#94599,#94600),(#94601,#94602,#94603),(#94604,#94605,#94606),(#94607,
#94608,#94609),(#94610,#94611,#94612),(#94613,#94614,#94615),(#94616,#94617,
#94618),(#94619,#94620,#94621),(#94622,#94623,#94624),(#94625,#94626,#94627),
(#94628,#94629,#94630),(#94631,#94632,#94633),(#94634,#94635,#94636),(#94637,
#94638,#94639),(#94640,#94641,#94642),(#94643,#94644,#94645),(#94646,#94647,
#94648),(#94649,#94650,#94651),(#94652,#94653,#94654),(#94655,#94656,#94657),
(#94658,#94659,#94660),(#94661,#94662,#94663),(#94664,#94665,#94666)),
 .UNSPECIFIED.,.F.,.F.,.F.)
B_SPLINE_SURFACE_WITH_KNOTS((4,2,2,2,2,2,2,2,2,2,2,2,2,2,2,4),(3,3),(0.,
0.0224324402603045,0.044864880520609,0.0672973207809135,0.0785135409110657,
0.089729761041218,0.112162201301522,0.123378421431675,0.134594641561827,
0.140202751626903,0.145810861691979,0.157027081822131,0.168243301952284,
0.171047356984822,0.17385141201736,0.179459522082436),(0.,1.),
 .UNSPECIFIED.)
GEOMETRIC_REPRESENTATION_ITEM()
RATIONAL_B_SPLINE_SURFACE(((1.,0.707106781186547,1.),(1.,0.707106781186547,
1.),(1.,0.707106781186548,1.),(1.,0.707106781186548,1.),(1.,0.707106781186548,
1.),(1.,0.707106781186548,1.),(1.,0.707106781186548,1.),(1.,0.707106781186548,
1.),(1.,0.707106781186548,1.),(1.,0.707106781186548,1.),(1.,0.707106781186548,
1.),(1.,0.707106781186548,1.),(1.,0.707106781186548,1.),(1.,0.707106781186548,
1.),(1.,0.707106781186548,1.),(1.,0.707106781186548,1.),(1.,0.707106781186548,
1.),(1.,0.707106781186548,1.),(1.,0.707106781186548,1.),(1.,0.707106781186548,
1.),(1.,0.707106781186548,1.),(1.,0.707106781186548,1.),(1.,0.707106781186548,
1.),(1.,0.707106781186548,1.),(1.,0.707106781186548,1.),(1.,0.707106781186548,
1.),(1.,0.707106781186557,1.),(1.,0.707106781186557,1.),(1.,0.707106781186548,
1.),(1.,0.707106781186548,1.),(1.,0.707106781186554,1.),(1.,0.707106781186554,
1.)))
REPRESENTATION_ITEM('')
SURFACE()
);
#1653=(
BOUNDED_SURFACE()
B_SPLINE_SURFACE(3,2,((#94746,#94747,#94748),(#94749,#94750,#94751),(#94752,
#94753,#94754),(#94755,#94756,#94757)),.UNSPECIFIED.,.F.,.F.,.F.)
B_SPLINE_SURFACE_WITH_KNOTS((4,4),(3,3),(0.,0.000852980308014371),(0.,1.),
 .UNSPECIFIED.)
GEOMETRIC_REPRESENTATION_ITEM()
RATIONAL_B_SPLINE_SURFACE(((1.,0.70710678118654,1.),(1.,0.708115537335819,
1.),(1.,0.709103401373757,1.),(1.,0.710072428249464,1.)))
REPRESENTATION_ITEM('')
SURFACE()
);
#1654=(
BOUNDED_SURFACE()
B_SPLINE_SURFACE(3,2,((#94763,#94764,#94765),(#94766,#94767,#94768),(#94769,
#94770,#94771),(#94772,#94773,#94774),(#94775,#94776,#94777),(#94778,#94779,
#94780),(#94781,#94782,#94783),(#94784,#94785,#94786),(#94787,#94788,#94789),
(#94790,#94791,#94792)),.UNSPECIFIED.,.F.,.F.,.F.)
B_SPLINE_SURFACE_WITH_KNOTS((4,2,2,2,4),(3,3),(-9.09012448646607E-14,0.0074893773271988,
0.0149787546544885,0.0224681319817782,0.0299575093090679),(0.,1.),
 .UNSPECIFIED.)
GEOMETRIC_REPRESENTATION_ITEM()
RATIONAL_B_SPLINE_SURFACE(((1.,0.707106781186548,1.),(1.,0.707106781186548,
1.),(1.,0.707106781186553,1.),(1.,0.707106781186553,1.),(1.,0.707106781186547,
1.),(1.,0.707106781186547,1.),(1.,0.707106781186548,1.),(1.,0.707106781186548,
1.),(1.,0.707106781186548,1.),(1.,0.707106781186548,1.)))
REPRESENTATION_ITEM('')
SURFACE()
);
#1655=(
BOUNDED_SURFACE()
B_SPLINE_SURFACE(3,2,((#94873,#94874,#94875),(#94876,#94877,#94878),(#94879,
#94880,#94881),(#94882,#94883,#94884),(#94885,#94886,#94887),(#94888,#94889,
#94890),(#94891,#94892,#94893),(#94894,#94895,#94896),(#94897,#94898,#94899),
(#94900,#94901,#94902),(#94903,#94904,#94905),(#94906,#94907,#94908),(#94909,
#94910,#94911),(#94912,#94913,#94914),(#94915,#94916,#94917),(#94918,#94919,
#94920),(#94921,#94922,#94923),(#94924,#94925,#94926),(#94927,#94928,#94929),
(#94930,#94931,#94932),(#94933,#94934,#94935),(#94936,#94937,#94938),(#94939,
#94940,#94941),(#94942,#94943,#94944),(#94945,#94946,#94947),(#94948,#94949,
#94950),(#94951,#94952,#94953),(#94954,#94955,#94956),(#94957,#94958,#94959),
(#94960,#94961,#94962),(#94963,#94964,#94965),(#94966,#94967,#94968),(#94969,
#94970,#94971),(#94972,#94973,#94974),(#94975,#94976,#94977),(#94978,#94979,
#94980),(#94981,#94982,#94983),(#94984,#94985,#94986),(#94987,#94988,#94989),
(#94990,#94991,#94992),(#94993,#94994,#94995),(#94996,#94997,#94998),(#94999,
#95000,#95001),(#95002,#95003,#95004),(#95005,#95006,#95007),(#95008,#95009,
#95010),(#95011,#95012,#95013),(#95014,#95015,#95016),(#95017,#95018,#95019),
(#95020,#95021,#95022),(#95023,#95024,#95025),(#95026,#95027,#95028),(#95029,
#95030,#95031),(#95032,#95033,#95034),(#95035,#95036,#95037),(#95038,#95039,
#95040),(#95041,#95042,#95043),(#95044,#95045,#95046),(#95047,#95048,#95049),
(#95050,#95051,#95052),(#95053,#95054,#95055),(#95056,#95057,#95058),(#95059,
#95060,#95061),(#95062,#95063,#95064),(#95065,#95066,#95067),(#95068,#95069,
#95070),(#95071,#95072,#95073),(#95074,#95075,#95076),(#95077,#95078,#95079),
(#95080,#95081,#95082),(#95083,#95084,#95085),(#95086,#95087,#95088),(#95089,
#95090,#95091),(#95092,#95093,#95094),(#95095,#95096,#95097),(#95098,#95099,
#95100),(#95101,#95102,#95103),(#95104,#95105,#95106),(#95107,#95108,#95109),
(#95110,#95111,#95112),(#95113,#95114,#95115),(#95116,#95117,#95118),(#95119,
#95120,#95121),(#95122,#95123,#95124),(#95125,#95126,#95127),(#95128,#95129,
#95130),(#95131,#95132,#95133),(#95134,#95135,#95136),(#95137,#95138,#95139),
(#95140,#95141,#95142),(#95143,#95144,#95145),(#95146,#95147,#95148),(#95149,
#95150,#95151),(#95152,#95153,#95154),(#95155,#95156,#95157),(#95158,#95159,
#95160),(#95161,#95162,#95163),(#95164,#95165,#95166),(#95167,#95168,#95169),
(#95170,#95171,#95172),(#95173,#95174,#95175),(#95176,#95177,#95178),(#95179,
#95180,#95181),(#95182,#95183,#95184),(#95185,#95186,#95187),(#95188,#95189,
#95190),(#95191,#95192,#95193),(#95194,#95195,#95196),(#95197,#95198,#95199),
(#95200,#95201,#95202),(#95203,#95204,#95205),(#95206,#95207,#95208),(#95209,
#95210,#95211),(#95212,#95213,#95214),(#95215,#95216,#95217),(#95218,#95219,
#95220)),.UNSPECIFIED.,.F.,.F.,.F.)
B_SPLINE_SURFACE_WITH_KNOTS((4,2,2,2,2,2,2,2,2,2,2,2,2,2,2,2,2,2,2,2,2,
2,2,2,2,2,2,2,2,2,2,2,2,2,2,2,2,2,2,2,2,2,2,2,2,2,2,2,2,2,2,2,2,2,2,2,2,
4),(3,3),(-0.000159417639105601,5.25012345884415E-5,0.000105002469176911,
0.000210004938353849,0.000420009876707727,0.000840019753415481,0.00168003950683099,
0.00336007901366201,0.00504011852049303,0.00672015802732404,0.0100802370409861,
0.0134403160546481,0.0168003950683101,0.0201604740819722,0.0235205530956342,
0.0268806321092963,0.0302407111229583,0.0336007901366203,0.0369608691502824,
0.0403209481639444,0.0436810271776064,0.0453610666844374,0.0470411061912685,
0.0487211456980995,0.0504011852049305,0.051241204958346,0.0520812247117615,
0.052921244465177,0.0537612642185925,0.054601283972008,0.0550212938487158,
0.0554413037254236,0.0558613136021313,0.0562813234788391,0.0567013333555468,
0.0571213432322546,0.0579613629856701,0.0588013827390856,0.0596414024925011,
0.0604814222459166,0.0621614617527476,0.0638415012595786,0.0655215407664097,
0.0672015802732407,0.0705616592869027,0.0739217383005648,0.0772818173142268,
0.0806418963278888,0.0873620543552129,0.094082212382537,0.100802370409861,
0.107522528437185,0.120962844491833,0.134403160546481,0.14784347660113,
0.161283792655778,0.188164424765074,0.215204474513476),(0.,1.00049765253644),
 .UNSPECIFIED.)
GEOMETRIC_REPRESENTATION_ITEM()
RATIONAL_B_SPLINE_SURFACE(((1.,0.999949367340627,1.00000005039494),(1.,
1.00000292399598,0.999999997089732),(1.,1.00000065570695,0.999999999347372),
(1.,0.999995149653455,1.00000000482757),(1.,0.999993866690958,1.00000000610451),
(1.,0.999989925403203,1.0000000100273),(1.,0.999987096878001,1.00000001284254),
(1.,0.99997833469904,1.00000002156358),(1.,0.999972169356053,1.00000002769998),
(1.,0.999953092103803,1.00000004668767),(1.,0.999939523207601,1.00000006019286),
(1.,0.999896582312161,1.00000010293215),(1.,0.999865028402933,1.00000013433792),
(1.,0.99976109014112,1.00000023778819),(1.,0.999679452472188,1.00000031904258),
(1.,0.99948567066185,1.0000005119146),(1.,0.99937353290825,1.00000062352587),
(1.,0.999110700111499,1.00000088512469),(1.,0.998960025063699,1.00000103509233),
(1.,0.998434367260317,1.00000155828221),(1.,0.997987950051853,1.00000200260352),
(1.,0.996776052520384,1.00000320881128),(1.,0.996011341315486,1.00000396993222),
(1.,0.993955400376975,1.00000601622067),(1.,0.992659906297562,1.0000073056325),
(1.,0.989276125492113,1.0000106735267),(1.,0.987170900665479,1.00001276886765),
(1.,0.98215667507351,1.00001775955182),(1.,0.979261511224488,1.00002064112308),
(1.,0.973160709403129,1.00002671328208),(1.,0.969970805398307,1.00002988820972),
(1.,0.9635930773515,1.0000362359948),(1.,0.960398704296731,1.00003941537051),
(1.,0.954031963961403,1.00004575221946),(1.,0.95085609693907,1.00004891317602),
(1.,0.9444675189357,1.00005527176011),(1.,0.941254261837805,1.0000584699312),
(1.,0.934708472493586,1.00006498498854),(1.,0.931376690992807,1.00006830112757),
(1.,0.924480383729073,1.00007516505718),(1.,0.920918391836673,1.00007871032578),
(1.,0.915258653779197,1.00008434349178),(1.,0.913318538561208,1.0000862744983),
(1.,0.909289199099064,1.0000902849203),(1.,0.907200548321262,1.00009236376502),
(1.,0.902807624646881,1.00009673606423),(1.,0.900504791744677,1.0000990280855),
(1.,0.895564714735884,1.00010394496921),(1.,0.892926137783545,1.00010657115824),
(1.,0.888550840104385,1.00011092591421),(1.,0.887026301150163,1.00011244329557),
(1.,0.883791478576254,1.00011566293089),(1.,0.88208209272103,1.0001173642913),
(1.,0.878387519679857,1.00012104151859),(1.,0.876404617983387,1.00012301511071),
(1.,0.871992495379262,1.00012740651872),(1.,0.869569843109419,1.00012981779681),
(1.,0.863909422913507,1.00013545164175),(1.,0.860681833252753,1.00013866407811),
(1.,0.854578489267958,1.00014473876734),(1.,0.85234061153918,1.00014696613839),
(1.,0.847339711856798,1.00015194355922),(1.,0.844566230719838,1.00015470401906),
(1.,0.838556583919586,1.00016068545101),(1.,0.835325483162265,1.00016390138198),
(1.,0.828864063959496,1.00017033246529),(1.,0.825653137654185,1.00017352831653),
(1.,0.819601311538472,1.00017955172977),(1.,0.816754485958108,1.00018238518971),
(1.,0.811453866107576,1.00018766092354),(1.,0.808994767190061,1.00019010847716),
(1.,0.802099709928181,1.00019697116263),(1.,0.798172772551782,1.00020087966333),
(1.,0.791166169096681,1.00020785337129),(1.,0.788081780349506,1.00021092327906),
(1.,0.782459542826891,1.00021651912058),(1.,0.779924928789769,1.00021904183479),
(1.,0.775247221203772,1.00022369758088),(1.,0.773105531885213,1.00022582921512),
(1.,0.76712446186861,1.00023178220445),(1.,0.763721566682336,1.00023516912329),
(1.,0.757649562702981,1.00024121261966),(1.,0.754986501187558,1.00024386317829),
(1.,0.750176146086482,1.00024865094913),(1.,0.748029059539643,1.00025078795526),
(1.,0.744138354127913,1.00025466039409),(1.,0.742391880608881,1.00025639866805),
(1.,0.737599380181131,1.00026116866803),(1.,0.734992429078544,1.00026376337969),
(1.,0.730493964703101,1.0002682407241),(1.,0.728608199101415,1.00027011763617),
(1.,0.725314975577855,1.00027339539825),(1.,0.723909745358972,1.00027479403102),
(1.,0.721433553601674,1.00027725859724),(1.,0.720363611737886,1.0002783235158),
(1.,0.717515918379571,1.00028115783945),(1.,0.716092416594757,1.00028257465799),
(1.,0.713767134874405,1.00028488902269),(1.,0.712870679247257,1.00028578126952),
(1.,0.71140011759095,1.000287244927),(1.,0.710826151043487,1.00028781619881),
(1.,0.709874603825523,1.00028876327859),(1.,0.709498188857635,1.00028913792631),
(1.,0.708557794279807,1.00029007390581),(1.,0.708176463449255,1.00029045344632),
(1.,0.707619701944943,1.00029100759387),(1.,0.707449638803699,1.00029117685857),
(1.,0.707205802728201,1.00029141954986),(1.,0.707133872162536,1.00029149114271),
(1.,0.707034573241446,1.00029158997543),(1.,0.707007932052635,1.00029161649154),
(1.,0.706956830206343,1.00029166735347),(1.,0.706958779087662,1.00029166541374),
(1.,0.7069598146507,1.00029166438304),(1.,0.706961036516168,1.00029166316691),
(0.999999999999999,0.706961022005169,1.00029166318135)))
REPRESENTATION_ITEM('')
SURFACE()
);
#1656=(
BOUNDED_SURFACE()
B_SPLINE_SURFACE(3,2,((#95897,#95898,#95899),(#95900,#95901,#95902),(#95903,
#95904,#95905),(#95906,#95907,#95908),(#95909,#95910,#95911),(#95912,#95913,
#95914),(#95915,#95916,#95917),(#95918,#95919,#95920),(#95921,#95922,#95923),
(#95924,#95925,#95926),(#95927,#95928,#95929),(#95930,#95931,#95932),(#95933,
#95934,#95935),(#95936,#95937,#95938),(#95939,#95940,#95941),(#95942,#95943,
#95944),(#95945,#95946,#95947),(#95948,#95949,#95950),(#95951,#95952,#95953),
(#95954,#95955,#95956),(#95957,#95958,#95959),(#95960,#95961,#95962),(#95963,
#95964,#95965),(#95966,#95967,#95968),(#95969,#95970,#95971),(#95972,#95973,
#95974),(#95975,#95976,#95977),(#95978,#95979,#95980),(#95981,#95982,#95983),
(#95984,#95985,#95986),(#95987,#95988,#95989),(#95990,#95991,#95992),(#95993,
#95994,#95995),(#95996,#95997,#95998),(#95999,#96000,#96001),(#96002,#96003,
#96004),(#96005,#96006,#96007),(#96008,#96009,#96010),(#96011,#96012,#96013),
(#96014,#96015,#96016),(#96017,#96018,#96019),(#96020,#96021,#96022),(#96023,
#96024,#96025),(#96026,#96027,#96028),(#96029,#96030,#96031),(#96032,#96033,
#96034),(#96035,#96036,#96037),(#96038,#96039,#96040),(#96041,#96042,#96043),
(#96044,#96045,#96046),(#96047,#96048,#96049),(#96050,#96051,#96052),(#96053,
#96054,#96055),(#96056,#96057,#96058),(#96059,#96060,#96061),(#96062,#96063,
#96064),(#96065,#96066,#96067),(#96068,#96069,#96070),(#96071,#96072,#96073),
(#96074,#96075,#96076),(#96077,#96078,#96079),(#96080,#96081,#96082),(#96083,
#96084,#96085),(#96086,#96087,#96088),(#96089,#96090,#96091),(#96092,#96093,
#96094),(#96095,#96096,#96097),(#96098,#96099,#96100),(#96101,#96102,#96103),
(#96104,#96105,#96106),(#96107,#96108,#96109),(#96110,#96111,#96112),(#96113,
#96114,#96115),(#96116,#96117,#96118),(#96119,#96120,#96121),(#96122,#96123,
#96124),(#96125,#96126,#96127),(#96128,#96129,#96130),(#96131,#96132,#96133),
(#96134,#96135,#96136),(#96137,#96138,#96139),(#96140,#96141,#96142),(#96143,
#96144,#96145),(#96146,#96147,#96148),(#96149,#96150,#96151),(#96152,#96153,
#96154),(#96155,#96156,#96157),(#96158,#96159,#96160),(#96161,#96162,#96163),
(#96164,#96165,#96166),(#96167,#96168,#96169),(#96170,#96171,#96172),(#96173,
#96174,#96175),(#96176,#96177,#96178)),.UNSPECIFIED.,.F.,.F.,.F.)
B_SPLINE_SURFACE_WITH_KNOTS((4,2,2,2,2,2,2,2,2,2,2,2,2,2,2,2,2,2,2,2,2,
2,2,2,2,2,2,2,2,2,2,2,2,2,2,2,2,2,2,2,2,2,2,2,2,2,4),(3,3),(-0.000455987201348429,
6.77530739903753E-5,0.000135506147980765,0.000271012295961543,0.0005420245919231,
0.00108404918384621,0.00216809836769244,0.0043361967353849,0.00650429510307735,
0.00867239347076981,0.0130085902061547,0.0151766885738472,0.0173447869415396,
0.0195128853092321,0.0216809836769245,0.023849082044617,0.0260171804123094,
0.0303533771476944,0.0346895738830793,0.0390257706184642,0.0433619673538491,
0.0455300657215415,0.047698164089234,0.0498662624569264,0.0509503116407727,
0.0520343608246189,0.0531184100084651,0.0536604346003882,0.0542024591923114,
0.0547444837842345,0.055015496080196,0.0552865083761576,0.0555575206721191,
0.0558285329680807,0.0560995452640423,0.0563705575600038,0.0569125821519269,
0.05745460674385,0.0579966313357732,0.0585386559276963,0.0596227051115425,
0.0607067542953887,0.0617908034792349,0.0628748526630812,0.0650429510307736,
0.0672110493984661,0.0693791477661585),(-0.00105667980444056,1.),
 .UNSPECIFIED.)
GEOMETRIC_REPRESENTATION_ITEM()
RATIONAL_B_SPLINE_SURFACE(((1.00000122872547,0.999418591393398,1.),(0.999999970682267,
1.00001387257154,1.),(0.999999984891384,1.00000714909853,1.),(1.0000000133113,
0.999993701353975,1.),(1.0000000169606,0.999991974577991,1.),(1.00000002816705,
0.999986671909136,1.),(1.00000003618925,0.999982875963573,1.),(1.00000006084249,
0.99997121053403,1.),(1.00000007816967,0.99996301165573,1.),(1.00000013222322,
0.999937434583641,1.),(1.00000017108158,0.999919047579035,1.),(1.00000029529396,
0.999860272733172,1.),(1.00000038845866,0.999816189039171,1.),(1.00000070251841,
0.999667582170744,1.),(1.00000095771891,0.99954682633964,1.),(1.00000159059792,
0.999247360501307,1.),(1.00000196820243,0.999068685507852,1.),(1.0000028904322,
0.998632304607156,1.),(1.00000343484386,0.998374699769646,1.),(1.00000541275052,
0.99743879342894,1.),(1.00000717381538,0.996605492340337,1.),(1.00001110917801,
0.994743356518011,1.),(1.00001264120727,0.994018430551732,1.),(1.00001629437776,
0.992289822476323,1.),(1.00001841824292,0.991284851457104,1.),(1.00002338906489,
0.988932756739908,1.),(1.00002624044633,0.987583539396207,1.),(1.00003266989126,
0.984541253121083,1.),(1.00003624703493,0.982848619430627,1.),(1.00004391733999,
0.979219182668691,1.),(1.00004800332235,0.977285776567571,1.),(1.00005640354012,
0.973310959535482,1.),(1.00006071496906,0.97127087656586,1.),(1.00007372132053,
0.96511652809888,1.),(1.00008246110805,0.960981033372461,1.),(1.00009983287502,
0.952761056566164,1.),(1.00010849085217,0.94866427288905,1.),(1.00012601542624,
0.940371990780815,1.),(1.00013488263451,0.936176203071392,1.),(1.00015325734255,
0.927481654375009,1.),(1.00016275199041,0.922988974649895,1.),(1.0001780326614,
0.915758463134714,1.),(1.00018330226891,0.913264989006041,1.),(1.00019438183262,
0.90802235842585,1.),(1.00020018692943,0.905275501342365,1.),(1.00021268132342,
0.8993634010367,1.),(1.00021935337707,0.896206317112169,1.),(1.00023061024255,
0.890879790841062,1.),(1.00023457668858,0.889002946966943,1.),(1.0002430696063,
0.884984266152402,1.),(1.00024759861899,0.882841226853296,1.),(1.00025759604395,
0.878110642946419,1.),(1.00026304750707,0.875531118337484,1.),(1.00027254695219,
0.871036168645314,1.),(1.0002759382853,0.869431456840574,1.),(1.00028339567493,
0.865902767449779,1.),(1.00028745809758,0.863980509341721,1.),(1.00029664982192,
0.859631167041402,1.),(1.00030180427318,0.857192182572172,1.),(1.00031072607401,
0.852970562746628,1.),(1.00031389851946,0.851469424257118,1.),(1.0003207022979,
0.848250010763257,1.),(1.00032433622182,0.846530509782674,1.),(1.00033205991999,
0.842875808456326,1.),(1.00033615148806,0.840939759307718,1.),(1.00034464121058,
0.836922590395633,1.),(1.00034903560759,0.83484324857865,1.),(1.0003578501401,
0.830672385995587,1.),(1.00036226481903,0.828583447176264,1.),(1.00037087202048,
0.824510689556839,1.),(1.00037506411381,0.822527073841625,1.),(1.00038714159423,
0.816812248801122,1.),(1.00039451387087,0.81332383319144,1.),(1.00040797039675,
0.806956471094042,1.),(1.00041408703279,0.804062199804767,1.),(1.00042528086499,
0.798765499632482,1.),(1.00043037654998,0.796354322200385,1.),(1.00043983949878,
0.791876641849007,1.),(1.00044420538629,0.789810790164972,1.),(1.00045647509847,
0.78400500485181,1.),(1.0004635657767,0.780649836045255,1.),(1.00047637896645,
0.774586887889098,1.),(1.00048209039966,0.771884350569236,1.),(1.00049254768431,
0.766936170141906,1.),(1.00049728941638,0.764692476240422,1.),(1.00050605146711,
0.760546447002399,1.),(1.0005100700131,0.758644950456529,1.),(1.00052128416306,
0.753338636324398,1.),(1.00052765962714,0.750321892724031,1.),(1.00053892919238,
0.744989357174405,1.),(1.00054380318641,0.742683079527015,1.),(1.00055251252087,
0.73856199458653,1.),(1.00055634149899,0.736750197813865,1.),(1.00055979741554,
0.735114926399246,1.)))
REPRESENTATION_ITEM('')
SURFACE()
);
#1657=(
BOUNDED_SURFACE()
B_SPLINE_SURFACE(3,2,((#96588,#96589,#96590),(#96591,#96592,#96593),(#96594,
#96595,#96596),(#96597,#96598,#96599),(#96600,#96601,#96602),(#96603,#96604,
#96605),(#96606,#96607,#96608),(#96609,#96610,#96611),(#96612,#96613,#96614),
(#96615,#96616,#96617),(#96618,#96619,#96620),(#96621,#96622,#96623),(#96624,
#96625,#96626),(#96627,#96628,#96629),(#96630,#96631,#96632),(#96633,#96634,
#96635),(#96636,#96637,#96638),(#96639,#96640,#96641),(#96642,#96643,#96644),
(#96645,#96646,#96647),(#96648,#96649,#96650),(#96651,#96652,#96653),(#96654,
#96655,#96656),(#96657,#96658,#96659),(#96660,#96661,#96662),(#96663,#96664,
#96665)),.UNSPECIFIED.,.F.,.F.,.F.)
B_SPLINE_SURFACE_WITH_KNOTS((4,2,2,2,2,2,2,2,2,2,2,2,4),(3,3),(0.155017009813997,
0.160281319258347,0.165545628702697,0.170809938147046,0.173442092869221,
0.174758170230309,0.176074247591396,0.181338557035746,0.18397071175792,
0.185286789119008,0.186602866480095,0.191867175924445,0.19714352226199),
(0.,1.0000120368932),.UNSPECIFIED.)
GEOMETRIC_REPRESENTATION_ITEM()
RATIONAL_B_SPLINE_SURFACE(((1.,0.850111718516678,1.00000360837847),(1.,
0.853975052401841,1.0000035153734),(1.,0.85784940533772,1.00000342210305),
(1.,0.865373998108453,1.00000324095761),(1.,0.869032295171854,1.00000315288855),
(1.,0.876071575182358,1.00000298342643),(1.,0.87945336507496,1.00000290201394),
(1.,0.884260511104441,1.00000278628773),(1.,0.885818521137499,1.00000274878053),
(1.,0.888078501958785,1.00000269437424),(1.,0.888819457713693,1.00000267653663),
(1.,0.890260900245237,1.00000264183565),(1.,0.890962995541521,1.00000262493355),
(1.,0.894376106658767,1.00000254276705),(1.,0.896789199731204,1.00000248467476),
(1.,0.899867832814397,1.0000024105604),(1.,0.900801953241813,1.00000238807259),
(1.,0.9021344685165,1.0000023559939),(1.,0.902568647198769,1.00000234554158),
(1.,0.903435292916418,1.00000232467813),(1.,0.90386932572828,1.00000231422932),
(1.,0.906115157049724,1.00000226016365),(1.,0.908273545910519,1.00000220820306),
(1.,0.913356587833321,1.000002085835),(1.,0.916197241241691,1.00000201744971),
(1.,0.918946876765757,1.00000195125558)))
REPRESENTATION_ITEM('')
SURFACE()
);
#1658=(
BOUNDED_SURFACE()
B_SPLINE_SURFACE(3,2,((#96751,#96752,#96753),(#96754,#96755,#96756),(#96757,
#96758,#96759),(#96760,#96761,#96762),(#96763,#96764,#96765),(#96766,#96767,
#96768),(#96769,#96770,#96771),(#96772,#96773,#96774),(#96775,#96776,#96777),
(#96778,#96779,#96780),(#96781,#96782,#96783),(#96784,#96785,#96786)),
 .UNSPECIFIED.,.F.,.F.,.F.)
B_SPLINE_SURFACE_WITH_KNOTS((4,2,2,2,2,4),(3,3),(0.0678369045371883,0.0816632472223668,
0.0954895899075452,0.123142275277902,0.150794960648259,0.178447646018616),
(0.,1.),.UNSPECIFIED.)
GEOMETRIC_REPRESENTATION_ITEM()
RATIONAL_B_SPLINE_SURFACE(((1.,0.707106781186538,1.),(1.,0.707106781186538,
1.),(1.,0.707106781186548,1.),(1.,0.707106781186548,1.),(1.,0.707106781186548,
1.),(1.,0.707106781186548,1.),(1.,0.707106781186548,1.),(1.,0.707106781186548,
1.),(1.,0.707106781186547,1.),(1.,0.707106781186547,1.),(1.,0.707106781186547,
1.),(1.,0.707106781186547,1.)))
REPRESENTATION_ITEM('')
SURFACE()
);
#1659=(
BOUNDED_SURFACE()
B_SPLINE_SURFACE(3,2,((#96801,#96802,#96803),(#96804,#96805,#96806),(#96807,
#96808,#96809),(#96810,#96811,#96812),(#96813,#96814,#96815),(#96816,#96817,
#96818),(#96819,#96820,#96821),(#96822,#96823,#96824),(#96825,#96826,#96827),
(#96828,#96829,#96830),(#96831,#96832,#96833),(#96834,#96835,#96836),(#96837,
#96838,#96839),(#96840,#96841,#96842)),.UNSPECIFIED.,.F.,.F.,.F.)
B_SPLINE_SURFACE_WITH_KNOTS((4,2,2,2,2,2,4),(3,3),(0.118318550770891,0.130409364032191,
0.142500177293491,0.154590990554791,0.166681803816091,0.190863430338691,
0.215045056861291),(0.,0.0769991253144525),.UNSPECIFIED.)
GEOMETRIC_REPRESENTATION_ITEM()
RATIONAL_B_SPLINE_SURFACE(((1.,0.977533303103487,0.958526438226447),(1.,
0.977510801002336,0.958484899308358),(1.,0.977496043811651,0.958457657508537),
(1.,0.977474369053602,0.958417645867262),(1.,0.977467466178115,0.958404903147037),
(1.,0.977457506956036,0.958386518405656),(1.,0.977454497282011,0.958380962542142),
(1.,0.977450352423876,0.958373311126773),(1.,0.977449238571154,0.9583712549527),
(1.,0.97744714373703,0.958367387885243),(1.,0.977447298282621,0.958367673176674),
(1.,0.977447427205131,0.958367911167852),(1.,0.97744747834083,0.958368005564442),
(1.,0.97744747834083,0.958368005564442)))
REPRESENTATION_ITEM('')
SURFACE()
);
#2188=B_SPLINE_CURVE_WITH_KNOTS('',3,(#85962,#85963,#85964,#85965,#85966,
#85967,#85968,#85969,#85970,#85971,#85972,#85973,#85974,#85975,#85976,#85977,
#85978,#85979,#85980,#85981,#85982,#85983,#85984,#85985,#85986,#85987,#85988,
#85989,#85990,#85991,#85992,#85993,#85994,#85995,#85996,#85997,#85998,#85999,
#86000,#86001,#86002,#86003,#86004,#86005,#86006,#86007,#86008,#86009,#86010,
#86011,#86012,#86013,#86014,#86015,#86016),.UNSPECIFIED.,.F.,.F.,(4,3,3,
3,3,3,3,3,3,3,3,3,3,3,3,3,3,3,4),(0.000201753170275764,0.000391372308539321,
0.000584482554336057,0.000714496028078632,0.0008767415620752,0.0010625312444393,
0.00107365626679827,0.00127227482719147,0.00143589683236403,0.00155172995387464,
0.00173223334765279,0.00179960500601608,0.00198632247061839,0.00216599342059071,
0.00222671834567407,0.00240462689396127,0.00258342197686667,0.00276178812585047,
0.00290170673747351),.UNSPECIFIED.);
#2189=B_SPLINE_CURVE_WITH_KNOTS('',3,(#86022,#86023,#86024,#86025,#86026,
#86027,#86028,#86029,#86030,#86031,#86032,#86033,#86034,#86035,#86036,#86037,
#86038,#86039,#86040,#86041,#86042,#86043,#86044,#86045,#86046,#86047,#86048,
#86049,#86050,#86051,#86052,#86053,#86054,#86055,#86056,#86057,#86058,#86059,
#86060,#86061,#86062,#86063,#86064,#86065,#86066,#86067,#86068,#86069,#86070,
#86071,#86072,#86073,#86074,#86075,#86076,#86077,#86078,#86079),
 .UNSPECIFIED.,.F.,.F.,(4,3,3,3,3,3,3,3,3,3,3,3,3,3,3,3,3,3,3,4),(0.,0.000522356852536227,
0.000973581345339098,0.000984510290454162,0.00147422172391699,0.00195092533138153,
0.00196902058090832,0.00225002553935448,0.00244233119126233,0.00246127572613544,
0.00274151904332241,0.00293687568327876,0.00295353087136256,0.00317316065111924,
0.00336741647887176,0.00343557230408307,0.00344578601658967,0.00363646086434783,
0.00381869545059764,0.00393804116181679),.UNSPECIFIED.);
#2190=B_SPLINE_CURVE_WITH_KNOTS('',3,(#86087,#86088,#86089,#86090,#86091,
#86092,#86093,#86094,#86095,#86096,#86097,#86098,#86099,#86100,#86101,#86102,
#86103,#86104,#86105,#86106,#86107,#86108,#86109,#86110,#86111,#86112,#86113,
#86114,#86115,#86116,#86117,#86118,#86119,#86120,#86121,#86122,#86123,#86124,
#86125,#86126,#86127,#86128,#86129,#86130,#86131,#86132,#86133,#86134,#86135,
#86136,#86137,#86138,#86139,#86140,#86141),.UNSPECIFIED.,.F.,.F.,(4,3,3,
3,3,3,3,3,3,3,3,3,3,3,3,3,3,3,4),(0.,0.000132978696347368,0.000270241287995725,
0.000411196528084791,0.000507024332052189,0.000517726876311709,0.000779514505849355,
0.00101404866410438,0.00103112302519988,0.00132345052735938,0.00162877172921639,
0.0019603915463655,0.00202809732820876,0.00204614960503823,0.0024101150598867,
0.0028021558357775,0.00304214599231314,0.0030527561475232,0.00405619465641752),
 .UNSPECIFIED.);
#2191=B_SPLINE_CURVE_WITH_KNOTS('',3,(#86147,#86148,#86149,#86150,#86151,
#86152,#86153,#86154,#86155,#86156,#86157,#86158,#86159,#86160,#86161,#86162,
#86163,#86164,#86165,#86166,#86167,#86168,#86169,#86170,#86171,#86172,#86173,
#86174,#86175,#86176,#86177,#86178,#86179,#86180,#86181,#86182,#86183),
 .UNSPECIFIED.,.F.,.F.,(4,3,3,3,3,3,3,3,3,3,3,3,4),(0.,0.000314989845557401,
0.000586378060207524,0.000591775134429816,0.000903988302624528,0.00117275612041505,
0.00118112606261453,0.00147953454208657,0.00175913418062257,0.00192133188362462,
0.00208133452678515,0.00223644178065543,0.0023455122408301),
 .UNSPECIFIED.);
#2192=B_SPLINE_CURVE_WITH_KNOTS('',3,(#86190,#86191,#86192,#86193,#86194,
#86195,#86196,#86197,#86198,#86199,#86200,#86201),.UNSPECIFIED.,.F.,.F.,
(4,2,2,2,2,4),(0.00051471383035223,0.0041158554304885,0.00591642623055662,
0.00771699703062475,0.0113181386307609,0.0149192802308972),
 .UNSPECIFIED.);
#2193=B_SPLINE_CURVE_WITH_KNOTS('',3,(#86203,#86204,#86205,#86206,#86207,
#86208,#86209,#86210,#86211,#86212,#86213,#86214,#86215,#86216,#86217,#86218,
#86219,#86220,#86221,#86222,#86223,#86224,#86225,#86226,#86227,#86228,#86229,
#86230,#86231,#86232,#86233,#86234,#86235,#86236,#86237,#86238,#86239,#86240,
#86241,#86242,#86243,#86244,#86245,#86246,#86247,#86248,#86249,#86250,#86251,
#86252,#86253,#86254,#86255,#86256,#86257,#86258,#86259,#86260,#86261,#86262,
#86263,#86264,#86265,#86266),.UNSPECIFIED.,.F.,.F.,(4,3,3,3,3,3,3,3,3,3,
3,3,3,3,3,3,3,3,3,3,3,4),(0.,0.00369526538577179,0.0036953789086402,0.00554306836296028,
0.00554307302616271,0.00739075781728036,0.00739094612820333,0.0110861367259205,
0.0110867689982037,0.0147815156345607,0.0147825819056023,0.0166292050888808,
0.0166304351141471,0.018476894543201,0.0184782074975879,0.0221722734518412,
0.0221734986832148,0.0240199629061612,0.0240210156826648,0.0258676523604813,
0.025868445268313,0.0295630312691215),.UNSPECIFIED.);
#2194=B_SPLINE_CURVE_WITH_KNOTS('',3,(#86268,#86269,#86270,#86271,#86272,
#86273),.UNSPECIFIED.,.F.,.F.,(4,2,4),(0.,0.00201691944843358,0.00403383889686717),
 .UNSPECIFIED.);
#2195=B_SPLINE_CURVE_WITH_KNOTS('',3,(#86275,#86276,#86277,#86278,#86279,
#86280,#86281,#86282,#86283,#86284,#86285,#86286,#86287,#86288,#86289,#86290,
#86291,#86292,#86293,#86294,#86295,#86296,#86297,#86298,#86299,#86300,#86301,
#86302,#86303,#86304,#86305,#86306,#86307,#86308,#86309,#86310,#86311,#86312,
#86313,#86314,#86315,#86316,#86317,#86318,#86319,#86320,#86321,#86322,#86323,
#86324,#86325,#86326,#86327,#86328,#86329,#86330,#86331,#86332,#86333,#86334,
#86335,#86336,#86337,#86338,#86339,#86340,#86341,#86342,#86343,#86344,#86345,
#86346,#86347,#86348,#86349,#86350,#86351,#86352,#86353,#86354,#86355,#86356,
#86357,#86358,#86359,#86360,#86361,#86362,#86363,#86364,#86365,#86366,#86367,
#86368),.UNSPECIFIED.,.F.,.F.,(4,3,3,3,3,3,3,3,3,3,3,3,3,3,3,3,3,3,3,3,
3,3,3,3,3,3,3,3,3,3,3,4),(0.0336249043084812,0.0343340923276341,0.0348588967541102,
0.0357053672787823,0.0360928891997393,0.0360932923083427,0.0385608740909975,
0.0385615770429876,0.0434968438735138,0.043497886927775,0.0447308363191429,
0.0447319180031058,0.045964828764772,0.0459659358769334,0.0484328136560302,
0.0484339372781486,0.0533687834385465,0.0533698239727818,0.0546027758841757,
0.0546037755549375,0.0558367683298048,0.055837722246927,0.058304753221063,
0.0583056028338379,0.0632407230035794,0.0632413203753338,0.0657087078948376,
0.0657091630133129,0.0681766927860958,0.0681770006224813,0.0720142225821143,
0.0731126625686122),.UNSPECIFIED.);
#2196=B_SPLINE_CURVE_WITH_KNOTS('',3,(#86370,#86371,#86372,#86373,#86374,
#86375,#86376),.UNSPECIFIED.,.F.,.F.,(4,3,4),(0.,0.0026726882593627,0.00335009582233665),
 .UNSPECIFIED.);
#2197=B_SPLINE_CURVE_WITH_KNOTS('',3,(#86389,#86390,#86391,#86392,#86393,
#86394,#86395,#86396,#86397,#86398),.UNSPECIFIED.,.F.,.F.,(4,2,2,2,4),(0.,
0.0376344322078685,0.075268864415737,0.113378213559111,0.151487562702486),
 .UNSPECIFIED.);
#2198=B_SPLINE_CURVE_WITH_KNOTS('',3,(#86402,#86403,#86404,#86405,#86406,
#86407,#86408,#86409,#86410,#86411),.UNSPECIFIED.,.F.,.F.,(4,2,2,2,4),(0.455861178528749,
0.493970527672123,0.532079876815497,0.569714309023366,0.607348741231234),
 .UNSPECIFIED.);
#2199=B_SPLINE_CURVE_WITH_KNOTS('',3,(#86420,#86421,#86422,#86423,#86424,
#86425,#86426,#86427,#86428,#86429),.UNSPECIFIED.,.F.,.F.,(4,2,2,2,4),(0.,
0.0376344322078685,0.075268864415737,0.113378213559111,0.151487562702485),
 .UNSPECIFIED.);
#2200=B_SPLINE_CURVE_WITH_KNOTS('',3,(#86433,#86434,#86435,#86436,#86437,
#86438,#86439,#86440,#86441,#86442),.UNSPECIFIED.,.F.,.F.,(4,2,2,2,4),(0.455861178528749,
0.493970527672123,0.532079876815497,0.569714309023366,0.607348741231234),
 .UNSPECIFIED.);
#2201=B_SPLINE_CURVE_WITH_KNOTS('',3,(#86451,#86452,#86453,#86454,#86455,
#86456,#86457,#86458,#86459,#86460),.UNSPECIFIED.,.F.,.F.,(4,2,2,2,4),(0.,
0.0376344322078685,0.075268864415737,0.113378213559111,0.151487562702486),
 .UNSPECIFIED.);
#2202=B_SPLINE_CURVE_WITH_KNOTS('',3,(#86464,#86465,#86466,#86467,#86468,
#86469,#86470,#86471,#86472,#86473),.UNSPECIFIED.,.F.,.F.,(4,2,2,2,4),(0.455861178528749,
0.493970527672123,0.532079876815497,0.569714309023366,0.607348741231234),
 .UNSPECIFIED.);
#2203=B_SPLINE_CURVE_WITH_KNOTS('',3,(#86486,#86487,#86488,#86489,#86490,
#86491,#86492,#86493,#86494,#86495,#86496,#86497,#86498,#86499,#86500,#86501,
#86502,#86503,#86504,#86505,#86506,#86507,#86508,#86509,#86510,#86511,#86512,
#86513,#86514,#86515,#86516,#86517,#86518,#86519,#86520,#86521,#86522,#86523,
#86524,#86525,#86526,#86527,#86528,#86529,#86530,#86531,#86532,#86533,#86534),
 .UNSPECIFIED.,.F.,.F.,(4,3,3,3,3,3,3,3,3,3,3,3,3,3,3,3,4),(0.,0.000109821895971414,
0.000223718409793574,0.000340120943679785,0.000386128285975577,0.000392555857712287,
0.000584663348330143,0.000759528189981808,0.000776770838947999,0.000785111715424574,
0.000978472745646417,0.00117183377586826,0.00117766757313686,0.00129027810656827,
0.00140353834105485,0.00151434258567243,0.00157022343084915),
 .UNSPECIFIED.);
#2204=B_SPLINE_CURVE_WITH_KNOTS('',3,(#86538,#86539,#86540,#86541,#86542,
#86543,#86544,#86545,#86546,#86547,#86548,#86549,#86550,#86551,#86552,#86553,
#86554,#86555,#86556,#86557,#86558,#86559,#86560,#86561,#86562,#86563,#86564,
#86565,#86566,#86567,#86568,#86569,#86570,#86571,#86572,#86573,#86574,#86575,
#86576,#86577,#86578,#86579,#86580,#86581,#86582,#86583,#86584,#86585,#86586,
#86587,#86588,#86589,#86590,#86591,#86592,#86593,#86594,#86595),
 .UNSPECIFIED.,.F.,.F.,(4,3,3,3,3,3,3,3,3,3,3,3,3,3,3,3,3,3,3,4),(0.,0.000111469447673193,
0.000178663865080732,0.000294336346988578,0.000331041450458318,0.000388183044974913,
0.000398191848878749,0.000413182492575923,0.000536788127134726,0.000600678349583499,
0.000694426278087287,0.000788174206591076,0.000795149710050332,0.000971945613108558,
0.00115606563722798,0.00118226130988662,0.00118727564039461,0.00131748712639905,
0.00144691776979061,0.00157634841318217),.UNSPECIFIED.);
#2205=B_SPLINE_CURVE_WITH_KNOTS('',3,(#86617,#86618,#86619,#86620,#86621,
#86622,#86623,#86624,#86625,#86626,#86627,#86628,#86629,#86630,#86631,#86632,
#86633,#86634,#86635,#86636,#86637,#86638,#86639,#86640,#86641,#86642,#86643,
#86644,#86645,#86646,#86647,#86648,#86649,#86650,#86651,#86652,#86653,#86654,
#86655,#86656,#86657,#86658,#86659),.UNSPECIFIED.,.F.,.F.,(4,3,3,3,3,3,
3,3,3,3,3,3,3,3,4),(0.,9.24121435778908E-5,0.000182286807566461,0.00022129722760121,
0.000307679864338664,0.000389567696567305,0.000421720982923359,0.000436387456642549,
0.000526984691978052,0.000610982297301783,0.000642714900038087,0.000669097214438017,
0.000737690381912385,0.000803424779895835,0.000843441965846719),
 .UNSPECIFIED.);
#2206=B_SPLINE_CURVE_WITH_KNOTS('',3,(#86662,#86663,#86664,#86665,#86666,
#86667,#86668,#86669,#86670,#86671,#86672,#86673,#86674,#86675,#86676,#86677,
#86678,#86679,#86680,#86681,#86682,#86683,#86684,#86685,#86686,#86687,#86688,
#86689,#86690,#86691,#86692,#86693,#86694,#86695,#86696,#86697,#86698,#86699,
#86700,#86701,#86702,#86703,#86704,#86705,#86706,#86707),.UNSPECIFIED.,
 .F.,.F.,(4,3,3,3,3,3,3,3,3,3,3,3,3,3,3,4),(0.,6.65927751009938E-5,0.000136207087983939,
0.00015351019459415,0.000200453902910958,0.000220309690001092,0.000313539212629657,
0.000400256492199074,0.000406768735258222,0.000420708176221917,0.000497485021765038,
0.000579980519596234,0.000621930854547057,0.000707656251985938,0.000795542926537232,
0.000841416352443835),.UNSPECIFIED.);
#2207=B_SPLINE_CURVE_WITH_KNOTS('',3,(#86729,#86730,#86731,#86732,#86733,
#86734,#86735,#86736,#86737,#86738,#86739,#86740,#86741,#86742,#86743,#86744,
#86745,#86746,#86747,#86748,#86749,#86750,#86751,#86752,#86753,#86754,#86755,
#86756,#86757,#86758,#86759,#86760,#86761,#86762,#86763,#86764,#86765,#86766,
#86767,#86768,#86769,#86770,#86771,#86772,#86773,#86774,#86775,#86776,#86777),
 .UNSPECIFIED.,.F.,.F.,(4,3,3,3,3,3,3,3,3,3,3,3,3,3,3,3,4),(0.,0.000109821895962571,
0.000223718409775525,0.000340120943651616,0.000386128285975588,0.000392555857712286,
0.000584663348330096,0.000759528190225243,0.000776770838947905,0.000785111715424573,
0.000978472745646407,0.00117183377586824,0.00117766757313686,0.00129027810657364,
0.00140353834106094,0.00151434258567274,0.00157022343084915),
 .UNSPECIFIED.);
#2208=B_SPLINE_CURVE_WITH_KNOTS('',3,(#86781,#86782,#86783,#86784,#86785,
#86786,#86787,#86788,#86789,#86790,#86791,#86792,#86793,#86794,#86795,#86796,
#86797,#86798,#86799,#86800,#86801,#86802,#86803,#86804,#86805,#86806,#86807,
#86808,#86809,#86810,#86811,#86812,#86813,#86814,#86815,#86816,#86817,#86818,
#86819,#86820,#86821,#86822,#86823,#86824,#86825,#86826,#86827,#86828,#86829,
#86830,#86831,#86832,#86833,#86834,#86835,#86836,#86837,#86838),
 .UNSPECIFIED.,.F.,.F.,(4,3,3,3,3,3,3,3,3,3,3,3,3,3,3,3,3,3,3,4),(0.,0.00011146944768469,
0.000178663865080786,0.000294336346967297,0.000331041450458361,0.000388183044974952,
0.000398191848878757,0.00041318249257596,0.00053678812714408,0.000600678349583523,
0.000694426278087305,0.000788174206591086,0.000795149710050351,0.000971945613065413,
0.00115606563713422,0.00118226130988663,0.00118727564039461,0.00131748712642929,
0.00144691776980573,0.00157634841318217),.UNSPECIFIED.);
#2209=B_SPLINE_CURVE_WITH_KNOTS('',3,(#86860,#86861,#86862,#86863,#86864,
#86865,#86866,#86867,#86868,#86869,#86870,#86871,#86872,#86873,#86874,#86875,
#86876,#86877,#86878,#86879,#86880,#86881,#86882,#86883,#86884,#86885,#86886,
#86887,#86888,#86889,#86890,#86891,#86892,#86893,#86894,#86895,#86896,#86897,
#86898,#86899,#86900,#86901,#86902),.UNSPECIFIED.,.F.,.F.,(4,3,3,3,3,3,
3,3,3,3,3,3,3,3,4),(0.,9.2412143565261E-5,0.000182286807543989,0.000221297227600963,
0.000307679864329089,0.000389567696548903,0.000421720982923359,0.000436387456642595,
0.00052698469192393,0.000610982297301772,0.000642714900038126,0.000669097214438008,
0.000737690381855536,0.000803424779780432,0.000843441965846718),
 .UNSPECIFIED.);
#2210=B_SPLINE_CURVE_WITH_KNOTS('',3,(#86905,#86906,#86907,#86908,#86909,
#86910,#86911,#86912,#86913,#86914,#86915,#86916,#86917,#86918,#86919,#86920,
#86921,#86922,#86923,#86924,#86925,#86926,#86927,#86928,#86929,#86930,#86931,
#86932,#86933,#86934,#86935,#86936,#86937,#86938,#86939,#86940,#86941,#86942,
#86943,#86944,#86945,#86946,#86947,#86948,#86949,#86950),.UNSPECIFIED.,
 .F.,.F.,(4,3,3,3,3,3,3,3,3,3,3,3,3,3,3,4),(0.,6.65927750353964E-5,0.00013620708785258,
0.000153510194594128,0.000200453902910995,0.000220309690001075,0.000313539212629635,
0.000400256492216322,0.000406768735258194,0.000420708176221917,0.00049748502176149,
0.000579980519588019,0.000621930854547426,0.000707656251980385,0.000795542926521112,
0.000841416352443835),.UNSPECIFIED.);
#2211=B_SPLINE_CURVE_WITH_KNOTS('',3,(#86972,#86973,#86974,#86975,#86976,
#86977,#86978,#86979,#86980,#86981,#86982,#86983,#86984,#86985,#86986,#86987,
#86988,#86989,#86990,#86991,#86992,#86993,#86994,#86995,#86996,#86997,#86998,
#86999,#87000,#87001,#87002,#87003,#87004,#87005,#87006,#87007,#87008,#87009,
#87010,#87011,#87012,#87013,#87014,#87015,#87016,#87017,#87018,#87019,#87020),
 .UNSPECIFIED.,.F.,.F.,(4,3,3,3,3,3,3,3,3,3,3,3,3,3,3,3,4),(0.,0.000109821895955179,
0.000223718409760101,0.000340120943627297,0.000386128285975582,0.000392555857712287,
0.000584663348330105,0.000759528190240281,0.000776770838947923,0.000785111715424574,
0.000978472745646415,0.00117183377586826,0.00117766757313686,0.0012902781065717,
0.00140353834105677,0.00151434258566574,0.00157022343084915),
 .UNSPECIFIED.);
#2212=B_SPLINE_CURVE_WITH_KNOTS('',3,(#87024,#87025,#87026,#87027,#87028,
#87029,#87030,#87031,#87032,#87033,#87034,#87035,#87036,#87037,#87038,#87039,
#87040,#87041,#87042,#87043,#87044,#87045,#87046,#87047,#87048,#87049,#87050,
#87051,#87052,#87053,#87054,#87055,#87056,#87057,#87058,#87059,#87060,#87061,
#87062,#87063,#87064,#87065,#87066,#87067,#87068,#87069,#87070,#87071,#87072,
#87073,#87074,#87075,#87076,#87077,#87078,#87079,#87080,#87081),
 .UNSPECIFIED.,.F.,.F.,(4,3,3,3,3,3,3,3,3,3,3,3,3,3,3,3,3,3,3,4),(0.,0.000111469447679236,
0.000178663865080771,0.000294336346982952,0.000331041450458349,0.000388183044974941,
0.000398191848878742,0.00041318249257595,0.000536788127148723,0.000600678349583517,
0.000694426278087301,0.000788174206591084,0.000795149710050379,0.000971945613071812,
0.00115606563714846,0.00118226130988662,0.00118727564039459,0.00131748712641446,
0.00144691776979831,0.00157634841318216),.UNSPECIFIED.);
#2213=B_SPLINE_CURVE_WITH_KNOTS('',3,(#87103,#87104,#87105,#87106,#87107,
#87108,#87109,#87110,#87111,#87112,#87113,#87114,#87115,#87116,#87117,#87118,
#87119,#87120,#87121,#87122,#87123,#87124,#87125,#87126,#87127,#87128,#87129,
#87130,#87131,#87132,#87133,#87134,#87135,#87136,#87137,#87138,#87139,#87140,
#87141,#87142,#87143,#87144,#87145),.UNSPECIFIED.,.F.,.F.,(4,3,3,3,3,3,
3,3,3,3,3,3,3,3,4),(0.,9.24121435661261E-5,0.000182286807546301,0.000221297227601306,
0.00030767986433129,0.000389567696553656,0.000421720982923359,0.000436387456642586,
0.000526984691977222,0.000610982297301761,0.000642714900038117,0.000669097214438,
0.000737690381925544,0.000803424779913494,0.000843441965846718),
 .UNSPECIFIED.);
#2214=B_SPLINE_CURVE_WITH_KNOTS('',3,(#87148,#87149,#87150,#87151,#87152,
#87153,#87154,#87155,#87156,#87157,#87158,#87159,#87160,#87161,#87162,#87163,
#87164,#87165,#87166,#87167,#87168,#87169,#87170,#87171,#87172,#87173,#87174,
#87175,#87176,#87177,#87178,#87179,#87180,#87181,#87182,#87183,#87184,#87185,
#87186,#87187,#87188,#87189,#87190,#87191,#87192,#87193),.UNSPECIFIED.,
 .F.,.F.,(4,3,3,3,3,3,3,3,3,3,3,3,3,3,3,4),(0.,6.65927750433562E-5,0.000136207087870291,
0.000153510194594151,0.000200453902910911,0.000220309690001092,0.000313539212629646,
0.000400256492213659,0.000406768735258199,0.000420708176221917,0.000497485021762217,
0.000579980519589639,0.000621930854547661,0.000707656251980853,0.000795542926521681,
0.000841416352443835),.UNSPECIFIED.);
#2215=B_SPLINE_CURVE_WITH_KNOTS('',3,(#87214,#87215,#87216,#87217,#87218,
#87219,#87220,#87221,#87222,#87223,#87224,#87225,#87226,#87227,#87228,#87229,
#87230,#87231,#87232,#87233,#87234,#87235,#87236,#87237,#87238,#87239,#87240,
#87241,#87242,#87243,#87244,#87245,#87246,#87247,#87248,#87249,#87250,#87251,
#87252,#87253,#87254,#87255,#87256,#87257,#87258,#87259,#87260,#87261,#87262,
#87263,#87264,#87265,#87266,#87267,#87268,#87269,#87270,#87271),
 .UNSPECIFIED.,.F.,.F.,(4,3,3,3,3,3,3,3,3,3,3,3,3,3,3,3,3,3,3,4),(0.,0.000142427063094415,
0.000289764879815003,0.0004406238037737,0.000539597691306959,0.000547604890660785,
0.000777640858258875,0.000994951020817798,0.0010850065158908,0.00109520978132157,
0.00129973831583479,0.00135974988827171,0.00136901222665201,0.0016002541036825,
0.00163575977437615,0.00164281467198245,0.00178996226046791,0.00193796990731151,
0.00208341869133047,0.00219041956264326),.UNSPECIFIED.);
#2216=B_SPLINE_CURVE_WITH_KNOTS('',3,(#87275,#87276,#87277,#87278,#87279,
#87280,#87281,#87282,#87283,#87284,#87285,#87286,#87287,#87288,#87289,#87290,
#87291,#87292,#87293,#87294,#87295,#87296,#87297,#87298,#87299,#87300,#87301,
#87302,#87303,#87304,#87305,#87306,#87307,#87308,#87309,#87310,#87311,#87312,
#87313,#87314,#87315,#87316,#87317,#87318,#87319,#87320,#87321,#87322,#87323,
#87324,#87325,#87326,#87327,#87328,#87329),.UNSPECIFIED.,.F.,.F.,(4,3,3,
3,3,3,3,3,3,3,3,3,3,3,3,3,3,3,4),(0.,0.000149745139195585,0.000303435116966849,
0.000457535596445036,0.00054874626362146,0.00055385056701855,0.000825671547130735,
0.00109749252724292,0.00110571813660245,0.0012824107487252,0.00137186565905368,
0.00137959364926584,0.00162472087354463,0.00164623879086444,0.00165222802848104,
0.00181217997322851,0.00197175562074787,0.00212790425251907,0.00219498505448598),
 .UNSPECIFIED.);
#2217=B_SPLINE_CURVE_WITH_KNOTS('',3,(#87335,#87336,#87337,#87338,#87339,
#87340,#87341,#87342,#87343,#87344,#87345,#87346,#87347,#87348,#87349,#87350,
#87351,#87352,#87353,#87354,#87355,#87356,#87357,#87358,#87359,#87360,#87361,
#87362,#87363,#87364,#87365,#87366,#87367,#87368,#87369,#87370,#87371,#87372,
#87373,#87374,#87375,#87376,#87377,#87378,#87379,#87380,#87381,#87382,#87383),
 .UNSPECIFIED.,.F.,.F.,(4,3,3,3,3,3,3,3,3,3,3,3,3,3,3,3,4),(0.,8.13766152637004E-5,
0.000166095243180767,0.000231150059491329,0.000279600583482743,0.000370403859907583,
0.000403777499519012,0.000524287940974636,0.000564363768371529,0.000576404939546696,
0.000685318810052787,0.000709431730850445,0.000855957854003566,0.000864607409320044,
0.000958227502067959,0.00105551869058068,0.00115280987909339),
 .UNSPECIFIED.);
#2218=B_SPLINE_CURVE_WITH_KNOTS('',3,(#87386,#87387,#87388,#87389,#87390,
#87391,#87392,#87393,#87394,#87395,#87396,#87397,#87398,#87399,#87400,#87401,
#87402,#87403,#87404,#87405,#87406,#87407,#87408,#87409,#87410,#87411,#87412,
#87413,#87414,#87415,#87416,#87417,#87418,#87419,#87420,#87421,#87422,#87423,
#87424,#87425,#87426,#87427,#87428),.UNSPECIFIED.,.F.,.F.,(4,3,3,3,3,3,
3,3,3,3,3,3,3,3,4),(0.,9.08098863106932E-5,0.000185034709549021,0.000277456643574092,
0.000285171347001819,0.000417664071564358,0.000524072108197603,0.00055944501884406,
0.000570342694003638,0.000673602018050586,0.000783825143420611,0.000848914171300631,
0.000962109447417837,0.00107297388323492,0.00114068538800723),
 .UNSPECIFIED.);
#2219=B_SPLINE_CURVE_WITH_KNOTS('',3,(#87434,#87435,#87436,#87437,#87438,
#87439,#87440,#87441,#87442,#87443,#87444,#87445,#87446,#87447,#87448,#87449,
#87450,#87451,#87452,#87453,#87454,#87455,#87456,#87457,#87458,#87459,#87460,
#87461,#87462,#87463,#87464,#87465,#87466,#87467,#87468,#87469,#87470,#87471,
#87472,#87473,#87474,#87475,#87476,#87477,#87478,#87479,#87480,#87481,#87482,
#87483,#87484,#87485,#87486,#87487,#87488,#87489,#87490,#87491,#87492,#87493,
#87494,#87495,#87496,#87497,#87498,#87499,#87500,#87501,#87502,#87503,#87504,
#87505,#87506,#87507,#87508,#87509,#87510,#87511,#87512,#87513,#87514,#87515,
#87516,#87517,#87518),.UNSPECIFIED.,.F.,.F.,(4,3,3,3,3,3,3,3,3,3,3,3,3,
3,3,3,3,3,3,3,3,3,3,3,3,3,3,3,4),(0.,0.015926332992886,0.023889499489329,
0.031852665985772,0.039815832482215,0.0477789989786579,0.0517605822268794,
0.0557421654751008,0.0637053319715438,0.0676869152197653,0.0696777068438761,
0.0716684984679868,0.0796316649644298,0.0816224565885406,0.0836132482126513,
0.0875948314608729,0.0955579979573159,0.0995395812055374,0.103521164453759,
0.111484330950202,0.115465914198423,0.119447497446645,0.127410663943087,
0.143336996935973,0.159263329928859,0.175189662921744,0.19111599591463,
0.222968661900401,0.254821327886172),.UNSPECIFIED.);
#2220=B_SPLINE_CURVE_WITH_KNOTS('',3,(#87520,#87521,#87522,#87523,#87524,
#87525,#87526,#87527,#87528,#87529,#87530,#87531,#87532,#87533,#87534,#87535,
#87536,#87537,#87538,#87539,#87540,#87541,#87542,#87543,#87544,#87545,#87546,
#87547,#87548,#87549,#87550,#87551,#87552,#87553,#87554,#87555,#87556,#87557,
#87558,#87559,#87560,#87561,#87562,#87563,#87564,#87565,#87566,#87567,#87568,
#87569,#87570,#87571,#87572,#87573,#87574,#87575,#87576,#87577,#87578,#87579,
#87580,#87581,#87582,#87583,#87584,#87585,#87586,#87587,#87588,#87589,#87590,
#87591,#87592,#87593,#87594,#87595,#87596,#87597,#87598,#87599,#87600,#87601),
 .UNSPECIFIED.,.F.,.F.,(4,3,3,3,3,3,3,3,3,3,3,3,3,3,3,3,3,3,3,3,3,3,3,3,
3,3,3,4),(0.,0.0319823773664769,0.0639647547329538,0.0799559434161923,0.0959471320994307,
0.111938320782669,0.127929509465908,0.135925103807527,0.143920698149146,
0.151916292490765,0.155914089661575,0.159911886832385,0.167907481174004,
0.169906379759409,0.171905278344814,0.175903075515623,0.183898669857243,
0.185897568442648,0.187896467028052,0.191894264198862,0.195892061369672,
0.199889858540482,0.207885452882102,0.215881047223722,0.223876641565341,
0.231872235906961,0.239867830248581,0.25585901893182),.UNSPECIFIED.);
#2221=B_SPLINE_CURVE_WITH_KNOTS('',3,(#87629,#87630,#87631,#87632,#87633,
#87634,#87635,#87636,#87637,#87638,#87639,#87640,#87641,#87642,#87643,#87644,
#87645,#87646,#87647,#87648,#87649,#87650,#87651,#87652,#87653,#87654,#87655,
#87656,#87657,#87658,#87659,#87660,#87661,#87662,#87663,#87664,#87665,#87666,
#87667,#87668,#87669,#87670,#87671,#87672,#87673,#87674,#87675,#87676,#87677,
#87678,#87679,#87680,#87681,#87682,#87683,#87684,#87685,#87686,#87687,#87688,
#87689,#87690,#87691,#87692,#87693,#87694,#87695,#87696,#87697,#87698,#87699,
#87700,#87701,#87702,#87703,#87704,#87705,#87706,#87707,#87708,#87709,#87710,
#87711,#87712,#87713,#87714,#87715,#87716,#87717,#87718,#87719,#87720,#87721,
#87722,#87723,#87724,#87725,#87726,#87727,#87728,#87729,#87730,#87731,#87732,
#87733,#87734,#87735,#87736,#87737,#87738,#87739,#87740,#87741,#87742,#87743,
#87744,#87745,#87746,#87747,#87748,#87749,#87750,#87751,#87752,#87753,#87754,
#87755,#87756,#87757,#87758,#87759,#87760,#87761,#87762,#87763,#87764,#87765,
#87766,#87767,#87768,#87769,#87770,#87771,#87772,#87773,#87774,#87775,#87776,
#87777,#87778,#87779,#87780,#87781,#87782,#87783,#87784,#87785,#87786,#87787,
#87788,#87789,#87790,#87791,#87792,#87793,#87794,#87795,#87796,#87797,#87798,
#87799,#87800,#87801,#87802,#87803,#87804,#87805,#87806,#87807,#87808,#87809,
#87810,#87811,#87812,#87813,#87814,#87815,#87816,#87817,#87818,#87819,#87820,
#87821,#87822,#87823,#87824,#87825,#87826,#87827,#87828,#87829,#87830),
 .UNSPECIFIED.,.F.,.F.,(4,3,3,3,3,3,3,3,3,3,3,3,3,3,3,3,3,3,3,3,3,3,3,3,
3,3,3,3,3,3,3,3,3,3,3,3,3,3,3,3,3,3,3,3,3,3,3,3,3,3,3,3,3,3,3,3,3,3,3,3,
3,3,3,3,3,3,3,4),(0.,0.0321347663513911,0.0495590544123357,0.0642731458325226,
0.08034498525143,0.0862931788198439,0.096420051205167,0.104175959222532,
0.112500619108118,0.118863546557499,0.127099328679868,0.128591290601529,
0.134437145537029,0.13664323902993,0.137833345962692,0.140671729597307,
0.141438649477965,0.144702441480307,0.145881989700091,0.150173982122068,
0.15277262499039,0.153697717723032,0.156609795436613,0.156813504295752,
0.157452006785746,0.160140339134182,0.160859452487887,0.161815966928969,
0.165392978615863,0.168754753105444,0.168969990302757,0.172572899244027,
0.173035427576007,0.17347524134314,0.174874914490513,0.175070484733593,
0.175252929180179,0.175430745910084,0.176752761163085,0.177106662985369,
0.177544810736285,0.180196510461824,0.182865217256473,0.185255162170941,
0.187290885676172,0.188723431177471,0.189325249765294,0.191782739905368,
0.193388999062593,0.196260693769467,0.199201867815336,0.201293292290039,
0.201495395322361,0.203648653929001,0.205190627207978,0.20553912739097,
0.208511016314483,0.20957779685043,0.213946752277146,0.217643568734126,
0.223067791290745,0.225698462781859,0.232343117717054,0.23374618069259,
0.240117376236147,0.24178905493371,0.252643459611325,0.257865728390371),
 .UNSPECIFIED.);
#2222=B_SPLINE_CURVE_WITH_KNOTS('',3,(#87831,#87832,#87833,#87834,#87835,
#87836,#87837,#87838,#87839,#87840,#87841,#87842,#87843,#87844,#87845,#87846,
#87847,#87848,#87849,#87850,#87851,#87852,#87853,#87854,#87855,#87856,#87857,
#87858,#87859,#87860,#87861,#87862,#87863,#87864,#87865,#87866,#87867,#87868,
#87869,#87870,#87871,#87872,#87873,#87874,#87875,#87876,#87877,#87878,#87879,
#87880,#87881,#87882,#87883,#87884,#87885,#87886,#87887,#87888,#87889,#87890,
#87891,#87892,#87893,#87894,#87895,#87896,#87897,#87898,#87899,#87900,#87901,
#87902,#87903,#87904,#87905,#87906,#87907,#87908,#87909,#87910,#87911,#87912,
#87913,#87914,#87915,#87916,#87917,#87918,#87919,#87920,#87921,#87922,#87923,
#87924,#87925,#87926,#87927,#87928,#87929,#87930,#87931,#87932,#87933,#87934,
#87935,#87936,#87937,#87938,#87939,#87940,#87941,#87942,#87943,#87944,#87945,
#87946,#87947,#87948,#87949,#87950,#87951,#87952,#87953,#87954,#87955,#87956,
#87957,#87958,#87959,#87960,#87961,#87962,#87963,#87964,#87965,#87966,#87967,
#87968,#87969,#87970,#87971,#87972,#87973,#87974,#87975,#87976,#87977,#87978,
#87979,#87980,#87981,#87982,#87983,#87984,#87985,#87986,#87987,#87988,#87989,
#87990,#87991,#87992,#87993,#87994,#87995,#87996,#87997,#87998,#87999,#88000,
#88001,#88002,#88003,#88004,#88005,#88006,#88007,#88008,#88009,#88010,#88011,
#88012,#88013,#88014,#88015,#88016,#88017,#88018,#88019,#88020,#88021,#88022,
#88023,#88024,#88025,#88026,#88027,#88028,#88029,#88030,#88031,#88032,#88033,
#88034,#88035,#88036,#88037,#88038,#88039,#88040,#88041,#88042,#88043,#88044,
#88045,#88046,#88047,#88048,#88049,#88050,#88051,#88052,#88053),
 .UNSPECIFIED.,.F.,.F.,(4,3,3,3,3,3,3,3,3,3,3,3,3,3,3,3,3,3,3,3,3,3,3,3,
3,3,3,3,3,3,3,3,3,3,3,3,3,3,3,3,3,3,3,3,3,3,3,3,3,3,3,3,3,3,3,3,3,3,3,3,
3,3,3,3,3,3,3,3,3,3,3,3,3,3,4),(1.38777878078145E-17,0.0106941639093447,
0.0161523461777034,0.0227402015251543,0.024233158169914,0.0280246446205861,
0.032318957692043,0.0343085312999032,0.039439559310476,0.040412204119208,
0.0438163939820961,0.0480516959393415,0.0485168201369417,0.0521392406465668,
0.0556011264251879,0.0566387545963194,0.0595190127146115,0.0607085988403213,
0.0641053404658499,0.0647854729869067,0.0683552918842684,0.0688694798512335,
0.0705958462991164,0.0709138855415459,0.0721915283538115,0.0729595587907659,
0.0756454538405821,0.0783958280485235,0.0811462022564649,0.083190893065739,
0.084213238470376,0.0847448494708462,0.085235583875013,0.0862567993079951,
0.0867688029516202,0.0869883753967039,0.0871941013119647,0.0872780147409773,
0.0882984146107854,0.0889848264050506,0.0893188144805935,0.0925804399340324,
0.095871378192766,0.0974647550772858,0.0994966706183769,0.100770759871012,
0.101528586159468,0.103558015878763,0.104572730738411,0.105084838473142,
0.105497282385778,0.105587445598059,0.109640760080191,0.111667417321258,
0.11305254753347,0.113694074562324,0.119113264047518,0.121790080016155,
0.128084746183264,0.129879086061019,0.138165401946804,0.144801674340403,
0.146044239431815,0.15806298841324,0.162199498439194,0.170274193011518,
0.174902658669718,0.177996378870079,0.178348887583842,0.189957445534057,
0.19449377824725,0.210635725330604,0.221799181517672,0.226777672413958,
0.259058112487482),.UNSPECIFIED.);
#2223=B_SPLINE_CURVE_WITH_KNOTS('',3,(#88071,#88072,#88073,#88074,#88075,
#88076,#88077,#88078,#88079,#88080,#88081,#88082,#88083,#88084,#88085,#88086,
#88087,#88088,#88089,#88090,#88091,#88092,#88093,#88094,#88095,#88096,#88097,
#88098,#88099,#88100,#88101,#88102,#88103,#88104,#88105,#88106,#88107,#88108,
#88109,#88110,#88111,#88112,#88113,#88114,#88115,#88116,#88117,#88118,#88119,
#88120,#88121,#88122,#88123,#88124,#88125,#88126,#88127,#88128,#88129,#88130,
#88131,#88132,#88133,#88134,#88135,#88136,#88137,#88138,#88139,#88140,#88141,
#88142,#88143,#88144,#88145,#88146,#88147,#88148,#88149,#88150,#88151,#88152,
#88153,#88154,#88155,#88156,#88157,#88158,#88159,#88160,#88161,#88162,#88163,
#88164,#88165,#88166,#88167,#88168,#88169,#88170,#88171,#88172,#88173,#88174,
#88175,#88176,#88177,#88178,#88179,#88180,#88181,#88182,#88183,#88184,#88185,
#88186,#88187,#88188,#88189,#88190,#88191,#88192,#88193,#88194,#88195,#88196,
#88197,#88198,#88199,#88200,#88201,#88202,#88203,#88204,#88205,#88206,#88207,
#88208,#88209,#88210,#88211,#88212,#88213,#88214,#88215,#88216,#88217,#88218,
#88219,#88220,#88221,#88222,#88223,#88224,#88225,#88226,#88227,#88228,#88229,
#88230,#88231,#88232,#88233,#88234,#88235,#88236,#88237,#88238,#88239,#88240,
#88241,#88242,#88243,#88244,#88245,#88246,#88247,#88248,#88249,#88250,#88251,
#88252,#88253,#88254,#88255,#88256,#88257,#88258,#88259,#88260,#88261,#88262,
#88263,#88264,#88265,#88266,#88267,#88268,#88269,#88270,#88271,#88272,#88273,
#88274,#88275,#88276,#88277,#88278,#88279,#88280,#88281,#88282,#88283,#88284,
#88285,#88286,#88287,#88288,#88289,#88290,#88291,#88292,#88293),
 .UNSPECIFIED.,.F.,.F.,(4,3,3,3,3,3,3,3,3,3,3,3,3,3,3,3,3,3,3,3,3,3,3,3,
3,3,3,3,3,3,3,3,3,3,3,3,3,3,3,3,3,3,3,3,3,3,3,3,3,3,3,3,3,3,3,3,3,3,3,3,
3,3,3,3,3,3,3,3,3,3,3,3,3,3,4),(0.,0.0106941636076985,0.0161523461777031,
0.0227402277212279,0.0242331581699135,0.028024634482012,0.0323189576920425,
0.0343085308806789,0.0394395588329036,0.0404122041192073,0.043816391934837,
0.0480516939348734,0.048516820136941,0.0521392405666208,0.0556011263566289,
0.0566387545963185,0.059519013554307,0.0607085988403205,0.0641053384666623,
0.0647854729869058,0.0683553012725267,0.0688694798512329,0.0705958456560103,
0.0709138855415449,0.0721915282587155,0.0729595587907649,0.0756454538060452,
0.078395828031255,0.0811462022564647,0.0831908930657383,0.0842132384703751,
0.0847448494807507,0.0852355838750119,0.0862567993079953,0.0867688029457022,
0.0869883753565705,0.0871941012416039,0.0872780147409787,0.0882984146107866,
0.0889848263941232,0.0893188144805945,0.0925804399957425,0.0958713775988918,
0.0974647550772867,0.0994966706183765,0.100770759912968,0.101528586159466,
0.10355801587876,0.104572730738408,0.105084838501772,0.105497282404785,
0.105587445598055,0.109640760080188,0.111667417321254,0.113052547649134,
0.113694074562321,0.119113264976225,0.121790080016154,0.128084747049764,
0.129879086061018,0.138165402400325,0.14480167568036,0.146044239431815,
0.158062989096084,0.162199498439194,0.170274193011518,0.174902656539617,
0.17799637619432,0.178348887583842,0.189957483032288,0.194493778247249,
0.210635725330603,0.22179915802068,0.226777672413957,0.259058112487481),
 .UNSPECIFIED.);
#2224=B_SPLINE_CURVE_WITH_KNOTS('',3,(#88294,#88295,#88296,#88297,#88298,
#88299,#88300,#88301,#88302,#88303,#88304,#88305,#88306,#88307,#88308,#88309,
#88310,#88311,#88312,#88313,#88314,#88315,#88316,#88317,#88318,#88319,#88320,
#88321,#88322,#88323,#88324,#88325,#88326,#88327,#88328,#88329,#88330,#88331,
#88332,#88333,#88334,#88335,#88336,#88337,#88338,#88339,#88340,#88341,#88342,
#88343,#88344,#88345,#88346,#88347,#88348,#88349,#88350,#88351,#88352,#88353,
#88354,#88355,#88356,#88357,#88358,#88359,#88360,#88361,#88362,#88363,#88364,
#88365,#88366,#88367,#88368,#88369,#88370,#88371,#88372,#88373,#88374,#88375,
#88376,#88377,#88378,#88379,#88380,#88381,#88382,#88383,#88384,#88385,#88386,
#88387,#88388,#88389,#88390,#88391,#88392,#88393,#88394,#88395,#88396,#88397,
#88398,#88399,#88400,#88401,#88402,#88403,#88404,#88405,#88406,#88407,#88408,
#88409,#88410,#88411,#88412,#88413,#88414,#88415,#88416,#88417,#88418,#88419,
#88420,#88421,#88422,#88423,#88424,#88425,#88426,#88427,#88428,#88429,#88430,
#88431,#88432,#88433,#88434,#88435,#88436,#88437,#88438,#88439,#88440,#88441,
#88442,#88443,#88444,#88445,#88446,#88447,#88448,#88449,#88450,#88451,#88452,
#88453,#88454,#88455,#88456,#88457,#88458,#88459,#88460,#88461,#88462,#88463,
#88464,#88465,#88466,#88467,#88468,#88469,#88470,#88471,#88472,#88473,#88474,
#88475,#88476,#88477,#88478,#88479,#88480,#88481,#88482,#88483,#88484,#88485,
#88486,#88487,#88488,#88489,#88490,#88491,#88492,#88493,#88494,#88495),
 .UNSPECIFIED.,.F.,.F.,(4,3,3,3,3,3,3,3,3,3,3,3,3,3,3,3,3,3,3,3,3,3,3,3,
3,3,3,3,3,3,3,3,3,3,3,3,3,3,3,3,3,3,3,3,3,3,3,3,3,3,3,3,3,3,3,3,3,3,3,3,
3,3,3,3,3,3,3,4),(6.16297582203915E-33,0.0321347663513911,0.0495589744394204,
0.0642731458325225,0.0803449852514303,0.0862931668316303,0.0964200512051673,
0.104175946597151,0.112500619108118,0.11886353125611,0.127099313737542,
0.12859129060153,0.134437149230977,0.136643239029932,0.137833345642357,
0.140671729597306,0.14143864949136,0.144702441480305,0.145881990070148,
0.150173982655845,0.152772624990387,0.15369771794186,0.156609795765364,
0.156813504295751,0.157452006799269,0.160140339164123,0.160859452487887,
0.161815966913,0.165392978607879,0.168754753103115,0.168969990302757,0.17257289992554,
0.173035427576007,0.173475241346685,0.174874914500988,0.175070484733593,
0.17525292917881,0.175430745909119,0.176752761147611,0.177106662985368,
0.177544810722352,0.180196510450715,0.18286521724812,0.185255162170942,
0.187290885676172,0.188723431189574,0.189325249765294,0.191782743547589,
0.193388999062593,0.196260694481045,0.199201866898202,0.201293290007858,
0.201495395322361,0.203648653861136,0.205190627103753,0.20553912739097,
0.208511015022924,0.20957779685043,0.213946752579418,0.217643568734125,
0.223067792625719,0.225698462781859,0.232343125900126,0.23374618069259,
0.240117367875956,0.24178905493371,0.252643459758372,0.257865728390371),
 .UNSPECIFIED.);
#2225=B_SPLINE_CURVE_WITH_KNOTS('',3,(#88693,#88694,#88695,#88696,#88697,
#88698,#88699,#88700,#88701,#88702,#88703,#88704,#88705,#88706,#88707,#88708,
#88709,#88710,#88711,#88712,#88713,#88714,#88715,#88716,#88717,#88718,#88719,
#88720,#88721,#88722,#88723,#88724,#88725,#88726,#88727,#88728,#88729,#88730,
#88731,#88732),.UNSPECIFIED.,.F.,.F.,(4,3,3,3,3,3,3,3,3,3,3,3,3,4),(0.000395514605004968,
0.00735803993026417,0.0147386515350848,0.0193564268053037,0.0234273968067644,
0.0287669019918199,0.0316481254819651,0.0395037906813469,0.0451972349114162,
0.0555782389740722,0.060131141684423,0.0877234345305647,0.0899989552304367,
0.11986676877645),.UNSPECIFIED.);
#2226=B_SPLINE_CURVE_WITH_KNOTS('',3,(#88734,#88735,#88736,#88737),
 .UNSPECIFIED.,.F.,.F.,(4,4),(3.69657704960075E-5,0.00377790776151813),
 .UNSPECIFIED.);
#2227=B_SPLINE_CURVE_WITH_KNOTS('',3,(#88739,#88740,#88741,#88742,#88743,
#88744,#88745,#88746,#88747,#88748,#88749,#88750,#88751,#88752,#88753,#88754,
#88755,#88756),.UNSPECIFIED.,.F.,.F.,(4,2,2,2,2,2,2,2,4),(3.84557724733612E-8,
0.0945840906584437,0.156697190455936,0.184260984131437,0.204445099552682,
0.225130065891661,0.254993330497327,0.329798839730618,0.408766486569211),
 .UNSPECIFIED.);
#2228=B_SPLINE_CURVE_WITH_KNOTS('',3,(#88758,#88759,#88760,#88761,#88762,
#88763,#88764,#88765,#88766,#88767,#88768,#88769,#88770,#88771,#88772,#88773,
#88774,#88775,#88776,#88777,#88778,#88779,#88780,#88781,#88782),
 .UNSPECIFIED.,.F.,.F.,(4,3,3,3,3,3,3,3,4),(5.10853787706198E-5,0.00062493792641946,
0.000987407891113938,0.00133852883324268,0.00149214424542401,0.00192050093150165,
0.00259944460152424,0.00332768414277843,0.00379637501318569),
 .UNSPECIFIED.);
#2229=B_SPLINE_CURVE_WITH_KNOTS('',3,(#88784,#88785,#88786,#88787,#88788,
#88789,#88790,#88791,#88792,#88793,#88794,#88795,#88796,#88797,#88798,#88799,
#88800,#88801,#88802,#88803,#88804,#88805,#88806,#88807,#88808,#88809,#88810,
#88811,#88812,#88813,#88814,#88815,#88816,#88817,#88818,#88819,#88820,#88821,
#88822,#88823,#88824,#88825),.UNSPECIFIED.,.F.,.F.,(4,2,2,2,2,2,2,2,2,2,
2,2,2,2,2,2,2,2,2,2,4),(0.00244866002632205,0.0182112504277692,0.0260925456284927,
0.0339738408292162,0.0418551360299397,0.0497364312306633,0.0576177264313868,
0.0654990216321103,0.0694396692324721,0.0733803168328338,0.0773209644331956,
0.0792912882333765,0.0812616120335574,0.0891429072342809,0.0930835548346426,
0.0970242024350043,0.104905497635728,0.112786792836451,0.116727440436813,
0.120668088037175,0.128549383237898),.UNSPECIFIED.);
#2230=B_SPLINE_CURVE_WITH_KNOTS('',3,(#88997,#88998,#88999,#89000,#89001,
#89002,#89003,#89004,#89005,#89006,#89007,#89008,#89009,#89010,#89011,#89012,
#89013,#89014,#89015,#89016,#89017,#89018,#89019,#89020,#89021,#89022,#89023,
#89024,#89025,#89026,#89027,#89028,#89029,#89030,#89031,#89032,#89033,#89034,
#89035,#89036,#89037,#89038,#89039,#89040,#89041,#89042,#89043,#89044,#89045,
#89046,#89047,#89048,#89049,#89050,#89051,#89052,#89053,#89054,#89055,#89056,
#89057,#89058,#89059,#89060,#89061,#89062,#89063,#89064,#89065,#89066,#89067,
#89068,#89069,#89070,#89071,#89072,#89073,#89074,#89075,#89076,#89077,#89078,
#89079,#89080,#89081,#89082,#89083,#89084,#89085,#89086,#89087,#89088,#89089,
#89090,#89091,#89092,#89093,#89094,#89095,#89096,#89097,#89098,#89099,#89100,
#89101,#89102,#89103,#89104,#89105,#89106,#89107,#89108,#89109,#89110,#89111,
#89112,#89113,#89114,#89115,#89116,#89117,#89118,#89119,#89120,#89121,#89122,
#89123,#89124,#89125,#89126,#89127,#89128,#89129,#89130,#89131,#89132,#89133,
#89134,#89135,#89136,#89137,#89138,#89139,#89140,#89141,#89142,#89143,#89144,
#89145,#89146,#89147,#89148,#89149,#89150,#89151,#89152,#89153,#89154,#89155,
#89156,#89157,#89158,#89159,#89160,#89161,#89162,#89163,#89164,#89165,#89166,
#89167,#89168,#89169,#89170,#89171,#89172,#89173,#89174,#89175,#89176,#89177,
#89178,#89179,#89180,#89181,#89182,#89183,#89184,#89185,#89186,#89187,#89188,
#89189,#89190,#89191,#89192,#89193,#89194,#89195,#89196,#89197,#89198,#89199,
#89200,#89201,#89202,#89203,#89204,#89205,#89206,#89207,#89208,#89209,#89210,
#89211,#89212,#89213,#89214,#89215,#89216,#89217,#89218,#89219,#89220,#89221,
#89222,#89223,#89224,#89225,#89226,#89227,#89228,#89229,#89230,#89231,#89232,
#89233,#89234,#89235,#89236,#89237,#89238,#89239,#89240,#89241,#89242,#89243,
#89244,#89245,#89246,#89247,#89248,#89249,#89250,#89251,#89252,#89253,#89254,
#89255,#89256,#89257,#89258,#89259,#89260,#89261,#89262,#89263,#89264),
 .UNSPECIFIED.,.F.,.F.,(4,3,3,3,3,3,3,3,3,3,3,3,3,3,3,3,3,3,3,3,3,3,3,3,
3,3,3,3,3,3,3,3,3,3,3,3,3,3,3,3,3,3,3,3,3,3,3,3,3,3,3,3,3,3,3,3,3,3,3,3,
3,3,3,3,3,3,3,3,3,3,3,3,3,3,3,3,3,3,3,3,3,3,3,3,3,3,3,3,3,4),(0.00290000689679031,
0.0348826539958882,0.0350963826156628,0.0668668642324351,0.0672927583345353,
0.082860078071171,0.0833909461939715,0.0945706526654511,0.0988570416155822,
0.0994891340534077,0.110217632937352,0.114848443355895,0.115587321912844,
0.123621459932078,0.130825599159465,0.13168550977228,0.137907945927169,
0.138805785100152,0.139734603701998,0.142569338258938,0.145202261479709,
0.146788974383255,0.147783697631716,0.151528124751556,0.154835996905122,
0.155832791561434,0.157625464684268,0.158877559866273,0.159857338526293,
0.161374923374203,0.162784053106398,0.162892508222113,0.163881885491152,
0.166084679257195,0.168252123500641,0.170375742136789,0.170967585801291,
0.17193097942087,0.172948658231983,0.17300624347377,0.174025064253037,0.174961804199926,
0.175043885032305,0.175955526385729,0.176776567282671,0.177588295814947,
0.177967799868159,0.179058628275698,0.179980073350588,0.181933154415629,
0.183873304502664,0.185793614314497,0.187147307106593,0.188029167280306,
0.188897271074614,0.189178590123301,0.190041440762736,0.191196751699605,
0.192053714245165,0.194476618658257,0.195242705240045,0.196078261210024,
0.197610910808871,0.199202289441857,0.199305039765874,0.200979572980401,
0.20270812750911,0.203367880943842,0.204127355139742,0.205268535517417,
0.206139628622172,0.208151902104601,0.210715513500852,0.211463812165016,
0.21217644906946,0.215080533727073,0.218147052981163,0.219623796694952,
0.220225542999178,0.223743899304297,0.227811751274587,0.228274636928896,
0.234017162824901,0.235987273171213,0.236323730858614,0.243348196588658,
0.244153738737961,0.244372824788332,0.25381684351193,0.260471012647768),
 .UNSPECIFIED.);
#2231=B_SPLINE_CURVE_WITH_KNOTS('',3,(#89277,#89278,#89279,#89280,#89281,
#89282),.UNSPECIFIED.,.F.,.F.,(4,2,4),(-0.370409044038645,-0.349794382456071,
-0.288542083039148),.UNSPECIFIED.);
#2232=B_SPLINE_CURVE_WITH_KNOTS('',3,(#89290,#89291,#89292,#89293,#89294,
#89295,#89296,#89297),.UNSPECIFIED.,.F.,.F.,(4,2,2,4),(-0.28854208306912,
-0.285779192265103,-0.236097520538759,-0.207305103379315),.UNSPECIFIED.);
#2233=B_SPLINE_CURVE_WITH_KNOTS('',3,(#89301,#89302,#89303,#89304,#89305,
#89306),.UNSPECIFIED.,.F.,.F.,(4,2,4),(-0.370409029704745,-0.349794370647721,
-0.288542073385836),.UNSPECIFIED.);
#2234=B_SPLINE_CURVE_WITH_KNOTS('',3,(#89311,#89312,#89313,#89314,#89315,
#89316,#89317,#89318),.UNSPECIFIED.,.F.,.F.,(4,2,2,4),(-0.288542084579862,
-0.285779193751398,-0.236097521603963,-0.20730510422017),.UNSPECIFIED.);
#2235=B_SPLINE_CURVE_WITH_KNOTS('',3,(#89321,#89322,#89323,#89324,#89325,
#89326),.UNSPECIFIED.,.F.,.F.,(4,2,4),(0.0586376217690057,0.0656506321388606,
0.0726636425083133),.UNSPECIFIED.);
#2236=B_SPLINE_CURVE_WITH_KNOTS('',3,(#89329,#89330,#89331,#89332,#89333,
#89334),.UNSPECIFIED.,.F.,.F.,(4,2,4),(0.0586376217689954,0.0656506321388567,
0.0726636425085365),.UNSPECIFIED.);
#2237=B_SPLINE_CURVE_WITH_KNOTS('',3,(#89766,#89767,#89768,#89769,#89770,
#89771,#89772,#89773,#89774,#89775,#89776,#89777,#89778,#89779,#89780,#89781,
#89782,#89783,#89784,#89785,#89786,#89787,#89788,#89789,#89790,#89791,#89792,
#89793,#89794,#89795,#89796,#89797,#89798,#89799,#89800,#89801,#89802,#89803,
#89804,#89805,#89806,#89807,#89808),.UNSPECIFIED.,.F.,.F.,(4,3,3,3,3,3,
3,3,3,3,3,3,3,3,4),(0.,8.9705753555212E-5,0.000183089135322613,0.000276472517090014,
0.000281553305630493,0.000416119195405342,0.000530992189354976,0.000557015156113086,
0.000563106611260986,0.000666450358589742,0.000774434672098113,0.000842506489703533,
0.000949864819656856,0.00104944593936403,0.00112621322252192),
 .UNSPECIFIED.);
#2238=B_SPLINE_CURVE_WITH_KNOTS('',3,(#89847,#89848,#89849,#89850,#89851,
#89852,#89853,#89854,#89855,#89856,#89857,#89858,#89859,#89860,#89861,#89862,
#89863,#89864,#89865,#89866,#89867,#89868,#89869,#89870,#89871,#89872,#89873,
#89874,#89875,#89876,#89877,#89878,#89879,#89880,#89881,#89882,#89883,#89884,
#89885,#89886,#89887,#89888,#89889,#89890,#89891,#89892,#89893,#89894,#89895,
#89896,#89897,#89898,#89899,#89900,#89901),.UNSPECIFIED.,.F.,.F.,(4,3,3,
3,3,3,3,3,3,3,3,3,3,3,3,3,3,3,4),(0.,0.000143392181484494,0.000291008849434949,
0.000439783745059069,0.000555292712107868,0.000556789243875147,0.00099691583468798,
0.00111258082262434,0.00111357848775029,0.0013912248898476,0.00139197310968786,
0.00166986892675867,0.00167036773162542,0.00178582121038124,0.00190189432266007,
0.00194876235356299,0.00206633842710468,0.00218183211487081,0.00222715697550056),
 .UNSPECIFIED.);
#2239=B_SPLINE_CURVE_WITH_KNOTS('',3,(#89962,#89963,#89964,#89965,#89966,
#89967,#89968,#89969,#89970,#89971,#89972,#89973,#89974,#89975,#89976,#89977,
#89978,#89979,#89980,#89981,#89982,#89983,#89984,#89985,#89986,#89987,#89988,
#89989,#89990,#89991,#89992,#89993,#89994,#89995,#89996,#89997,#89998,#89999,
#90000,#90001,#90002,#90003,#90004),.UNSPECIFIED.,.F.,.F.,(4,3,3,3,3,3,
3,3,3,3,3,3,3,3,4),(0.,9.05348581213434E-5,0.000186230685823136,0.000281926513524929,
0.000285981344804193,0.000428798602281781,0.000551039228772444,0.000563853027049858,
0.000571011012586812,0.000700764976115681,0.000820908721173626,0.000852457805291007,
0.000968426992556637,0.00107689164183138,0.00112770605409983),
 .UNSPECIFIED.);
#2240=B_SPLINE_CURVE_WITH_KNOTS('',3,(#90043,#90044,#90045,#90046,#90047,
#90048,#90049,#90050,#90051,#90052,#90053,#90054,#90055,#90056,#90057,#90058,
#90059,#90060,#90061,#90062,#90063,#90064,#90065,#90066,#90067,#90068,#90069,
#90070,#90071,#90072,#90073,#90074,#90075,#90076,#90077,#90078,#90079,#90080,
#90081,#90082,#90083,#90084,#90085,#90086,#90087,#90088,#90089,#90090,#90091,
#90092,#90093,#90094,#90095,#90096,#90097,#90098,#90099,#90100,#90101,#90102,
#90103),.UNSPECIFIED.,.F.,.F.,(4,3,3,3,3,3,3,3,3,3,3,3,3,3,3,3,3,3,3,3,
4),(0.,0.000156013234498623,0.00031658985362754,0.000479148774670394,0.000556927769468564,
0.00055839865504465,0.000679544683456882,0.000802052832349284,0.000837597982566976,
0.000954893942540085,0.00107174028492991,0.00111581667603572,0.0011167973100893,
0.00139526120827785,0.00139599663761163,0.00167470569152652,0.00167519596513395,
0.00183768579152785,0.0020007981043495,0.00216182265289023,0.00223359462017865),
 .UNSPECIFIED.);
#2241=B_SPLINE_CURVE_WITH_KNOTS('',3,(#90184,#90185,#90186,#90187,#90188,
#90189,#90190,#90191,#90192,#90193,#90194,#90195,#90196,#90197,#90198,#90199,
#90200,#90201,#90202,#90203,#90204,#90205,#90206,#90207,#90208,#90209,#90210,
#90211,#90212,#90213,#90214,#90215,#90216,#90217,#90218,#90219,#90220,#90221,
#90222,#90223,#90224,#90225,#90226),.UNSPECIFIED.,.F.,.F.,(4,3,3,3,3,3,
3,3,3,3,3,3,3,3,4),(0.,6.67265512522049E-5,0.000136622019400954,0.000153029544754912,
0.00019924472822554,0.000217818617549667,0.000312328270306139,0.000403808730923921,
0.000412185835933932,0.000489165233070777,0.00057076509789447,0.000614356689352663,
0.000696473891804212,0.000772875577879106,0.000824371671867865),
 .UNSPECIFIED.);
#2242=B_SPLINE_CURVE_WITH_KNOTS('',3,(#90259,#90260,#90261,#90262,#90263,
#90264,#90265,#90266,#90267,#90268,#90269,#90270,#90271,#90272,#90273,#90274,
#90275,#90276,#90277,#90278,#90279,#90280,#90281,#90282,#90283,#90284,#90285,
#90286,#90287,#90288,#90289,#90290,#90291,#90292,#90293,#90294,#90295,#90296,
#90297,#90298),.UNSPECIFIED.,.F.,.F.,(4,3,3,3,3,3,3,3,3,3,3,3,3,4),(0.,
8.52389357182548E-5,0.000172733323547372,0.000211640487491587,0.000298212835710885,
0.000380876745557343,0.000413153329460335,0.000422318843197918,0.000516826234508421,
0.000606276517040864,0.000627441770070006,0.00071476091751551,0.000798063637109017,
0.00082630665892067),.UNSPECIFIED.);
#2243=B_SPLINE_CURVE_WITH_KNOTS('',3,(#90351,#90352,#90353,#90354,#90355,
#90356,#90357,#90358,#90359,#90360,#90361,#90362,#90363,#90364,#90365,#90366,
#90367,#90368,#90369,#90370,#90371,#90372,#90373,#90374,#90375,#90376,#90377,
#90378,#90379,#90380,#90381,#90382,#90383,#90384,#90385,#90386,#90387,#90388,
#90389,#90390),.UNSPECIFIED.,.F.,.F.,(4,3,3,3,3,3,3,3,3,3,3,3,3,4),(0.,
0.00011221574809149,0.000227726453824885,0.000343358926450897,0.000400006487034198,
0.000401026826947022,0.000801373468181378,0.000802053653894043,0.00120274039453808,
0.00120308048084106,0.00131908058326075,0.001435186796666,0.00154804834527591,
0.00160410730778809),.UNSPECIFIED.);
#2244=B_SPLINE_CURVE_WITH_KNOTS('',3,(#90426,#90427,#90428,#90429,#90430,
#90431,#90432,#90433,#90434,#90435,#90436,#90437,#90438,#90439,#90440,#90441,
#90442,#90443,#90444,#90445,#90446,#90447,#90448,#90449,#90450,#90451,#90452,
#90453,#90454,#90455,#90456,#90457,#90458,#90459,#90460,#90461,#90462,#90463,
#90464,#90465,#90466,#90467,#90468,#90469,#90470,#90471,#90472,#90473,#90474,
#90475,#90476,#90477,#90478,#90479,#90480),.UNSPECIFIED.,.F.,.F.,(4,3,3,
3,3,3,3,3,3,3,3,3,3,3,3,3,3,3,4),(0.,0.000114915791844144,0.000172822750101235,
0.000292298157290126,0.00033117836085677,0.000390561714890095,0.000402052540286958,
0.000416541932279675,0.000550281559212149,0.000611393562701525,0.000745898236157288,
0.000805581435491517,0.000806245193123375,0.00116372865527049,0.00120903591007228,
0.00120936778968506,0.0013421660310875,0.00147732820866712,0.00161249038624675),
 .UNSPECIFIED.);
#2245=B_SPLINE_CURVE_WITH_KNOTS('',3,(#90548,#90549,#90550,#90551,#90552,
#90553,#90554,#90555,#90556,#90557,#90558,#90559,#90560,#90561,#90562,#90563,
#90564,#90565,#90566,#90567,#90568,#90569,#90570,#90571,#90572,#90573,#90574,
#90575,#90576,#90577,#90578,#90579,#90580,#90581,#90582,#90583,#90584,#90585,
#90586,#90587,#90588,#90589,#90590),.UNSPECIFIED.,.F.,.F.,(4,3,3,3,3,3,
3,3,3,3,3,3,3,3,4),(0.,6.67265512633752E-5,0.000136622019425751,0.000153029544754895,
0.000199244728225524,0.000217818617549654,0.000312328270310071,0.000403808730923931,
0.000412185835933931,0.000489165233073854,0.000570765097900325,0.0006143566893525,
0.000696473891807362,0.000772875577886235,0.000824371671867863),
 .UNSPECIFIED.);
#2246=B_SPLINE_CURVE_WITH_KNOTS('',3,(#90623,#90624,#90625,#90626,#90627,
#90628,#90629,#90630,#90631,#90632,#90633,#90634,#90635,#90636,#90637,#90638,
#90639,#90640,#90641,#90642,#90643,#90644,#90645,#90646,#90647,#90648,#90649,
#90650,#90651,#90652,#90653,#90654,#90655,#90656,#90657,#90658,#90659,#90660,
#90661,#90662),.UNSPECIFIED.,.F.,.F.,(4,3,3,3,3,3,3,3,3,3,3,3,3,4),(0.,
8.52389357147525E-5,0.000172733323539415,0.000211640487491721,0.000298212835707085,
0.000380876745550233,0.000413153329460335,0.000422318843197926,0.000516826234503452,
0.000606276517025046,0.000627441770069871,0.000714760917507696,0.000798063637099582,
0.00082630665892067),.UNSPECIFIED.);
#2247=B_SPLINE_CURVE_WITH_KNOTS('',3,(#90715,#90716,#90717,#90718,#90719,
#90720,#90721,#90722,#90723,#90724,#90725,#90726,#90727,#90728,#90729,#90730,
#90731,#90732,#90733,#90734,#90735,#90736,#90737,#90738,#90739,#90740,#90741,
#90742,#90743,#90744,#90745,#90746,#90747,#90748,#90749,#90750,#90751,#90752,
#90753,#90754),.UNSPECIFIED.,.F.,.F.,(4,3,3,3,3,3,3,3,3,3,3,3,3,4),(0.,
0.000112215748106196,0.000227726453854894,0.000343358926496841,0.000400006487034196,
0.000401026826947021,0.000801373468181415,0.000802053653894042,0.00120274039453804,
0.00120308048084106,0.00131908058325572,0.00143518679665637,0.00154804834526206,
0.00160410730778808),.UNSPECIFIED.);
#2248=B_SPLINE_CURVE_WITH_KNOTS('',3,(#90790,#90791,#90792,#90793,#90794,
#90795,#90796,#90797,#90798,#90799,#90800,#90801,#90802,#90803,#90804,#90805,
#90806,#90807,#90808,#90809,#90810,#90811,#90812,#90813,#90814,#90815,#90816,
#90817,#90818,#90819,#90820,#90821,#90822,#90823,#90824,#90825,#90826,#90827,
#90828,#90829,#90830,#90831,#90832,#90833,#90834,#90835,#90836,#90837,#90838,
#90839,#90840,#90841,#90842,#90843,#90844),.UNSPECIFIED.,.F.,.F.,(4,3,3,
3,3,3,3,3,3,3,3,3,3,3,3,3,3,3,4),(0.,0.000114915791837638,0.000172822750101249,
0.000292298157306797,0.00033117836085678,0.000390561714890105,0.000402052540286979,
0.000416541932279684,0.000550281559217109,0.00061139356270153,0.000745898236163757,
0.00080558143549149,0.000806245193123376,0.00116372865379815,0.00120903591007227,
0.00120936778968506,0.00134216603106807,0.00147732820865741,0.00161249038624675),
 .UNSPECIFIED.);
#2249=B_SPLINE_CURVE_WITH_KNOTS('',3,(#90912,#90913,#90914,#90915,#90916,
#90917,#90918,#90919,#90920,#90921,#90922,#90923,#90924,#90925,#90926,#90927,
#90928,#90929,#90930,#90931,#90932,#90933,#90934,#90935,#90936,#90937,#90938,
#90939,#90940,#90941,#90942,#90943,#90944,#90945,#90946,#90947,#90948,#90949,
#90950,#90951,#90952,#90953,#90954),.UNSPECIFIED.,.F.,.F.,(4,3,3,3,3,3,
3,3,3,3,3,3,3,3,4),(0.,6.67265512482609E-5,0.000136622019394041,0.000153029544754874,
0.000199244728225511,0.000217818617549638,0.000312328270301001,0.000403808730923887,
0.000412185835933931,0.000489165233063715,0.000570765097881359,0.000614356689352532,
0.00069647389179857,0.000772875577868274,0.000824371671867862),
 .UNSPECIFIED.);
#2250=B_SPLINE_CURVE_WITH_KNOTS('',3,(#90987,#90988,#90989,#90990,#90991,
#90992,#90993,#90994,#90995,#90996,#90997,#90998,#90999,#91000,#91001,#91002,
#91003,#91004,#91005,#91006,#91007,#91008,#91009,#91010,#91011,#91012,#91013,
#91014,#91015,#91016,#91017,#91018,#91019,#91020,#91021,#91022,#91023,#91024,
#91025,#91026),.UNSPECIFIED.,.F.,.F.,(4,3,3,3,3,3,3,3,3,3,3,3,3,4),(0.,
8.5238935718577E-5,0.000172733323546976,0.000211640487491245,0.000298212835710136,
0.000380876745556722,0.000413153329460335,0.000422318843197919,0.000516826234506355,
0.000606276517037616,0.000627441770070124,0.000714760917514443,0.000798063637110687,
0.00082630665892067),.UNSPECIFIED.);
#2251=B_SPLINE_CURVE_WITH_KNOTS('',3,(#91079,#91080,#91081,#91082,#91083,
#91084,#91085,#91086,#91087,#91088,#91089,#91090,#91091,#91092,#91093,#91094,
#91095,#91096,#91097,#91098,#91099,#91100,#91101,#91102,#91103,#91104,#91105,
#91106,#91107,#91108,#91109,#91110,#91111,#91112,#91113,#91114,#91115,#91116,
#91117,#91118),.UNSPECIFIED.,.F.,.F.,(4,3,3,3,3,3,3,3,3,3,3,3,3,4),(0.,
0.000112215748089412,0.000227726453820774,0.000343358926444529,0.000400006487034207,
0.000401026826947022,0.000801373468181404,0.000802053653894045,0.00120274039453804,
0.00120308048084107,0.00131908058325539,0.00143518679665721,0.00154804834526584,
0.00160410730778809),.UNSPECIFIED.);
#2252=B_SPLINE_CURVE_WITH_KNOTS('',3,(#91154,#91155,#91156,#91157,#91158,
#91159,#91160,#91161,#91162,#91163,#91164,#91165,#91166,#91167,#91168,#91169,
#91170,#91171,#91172,#91173,#91174,#91175,#91176,#91177,#91178,#91179,#91180,
#91181,#91182,#91183,#91184,#91185,#91186,#91187,#91188,#91189,#91190,#91191,
#91192,#91193,#91194,#91195,#91196,#91197,#91198,#91199,#91200,#91201,#91202,
#91203,#91204,#91205,#91206,#91207,#91208),.UNSPECIFIED.,.F.,.F.,(4,3,3,
3,3,3,3,3,3,3,3,3,3,3,3,3,3,3,4),(0.,0.000114915791794343,0.000172822750101289,
0.000292298157340931,0.000331178360856813,0.000390561714890135,0.00040205254028697,
0.000416541932279713,0.00055028155921315,0.000611393562701549,0.000745898236154648,
0.000805581435491558,0.000806245193123386,0.00116372865600683,0.00120903591007228,
0.00120936778968507,0.00134216603108612,0.00147732820866644,0.00161249038624675),
 .UNSPECIFIED.);
#2253=B_SPLINE_CURVE_WITH_KNOTS('',3,(#91391,#91392,#91393,#91394),
 .UNSPECIFIED.,.F.,.F.,(4,4),(-0.92505235407501,-0.312867444040557),
 .UNSPECIFIED.);
#2254=B_SPLINE_CURVE_WITH_KNOTS('',3,(#91419,#91420,#91421,#91422,#91423,
#91424,#91425,#91426,#91427,#91428,#91429,#91430,#91431),.UNSPECIFIED.,
 .F.,.F.,(4,3,3,3,4),(2.77555756156289E-17,0.00107584967114952,0.00186640722503582,
0.00326502442945365,0.00374644515873592),.UNSPECIFIED.);
#2255=B_SPLINE_CURVE_WITH_KNOTS('',3,(#91464,#91465,#91466,#91467,#91468,
#91469),.UNSPECIFIED.,.F.,.F.,(4,2,4),(0.,0.00205629279785326,0.00411258559570652),
 .UNSPECIFIED.);
#2256=B_SPLINE_CURVE_WITH_KNOTS('',3,(#91494,#91495,#91496,#91497,#91498,
#91499,#91500,#91501,#91502,#91503,#91504,#91505,#91506),.UNSPECIFIED.,
 .F.,.F.,(4,3,3,3,4),(0.,0.00135643839013762,0.00187754543955613,0.00293345159169245,
0.00374102163234538),.UNSPECIFIED.);
#2257=B_SPLINE_CURVE_WITH_KNOTS('',3,(#91555,#91556,#91557,#91558,#91559,
#91560,#91561,#91562,#91563,#91564,#91565,#91566,#91567,#91568,#91569,#91570,
#91571,#91572,#91573,#91574,#91575,#91576,#91577,#91578,#91579,#91580,#91581,
#91582),.UNSPECIFIED.,.F.,.F.,(4,3,3,3,3,3,3,3,3,4),(0.,0.00952633528178463,
0.0149413816810589,0.027827346998543,0.0298764199626499,0.044807721980472,
0.0597366932955049,0.0825180253977875,0.0895905783515619,0.119441539355168),
 .UNSPECIFIED.);
#2258=B_SPLINE_CURVE_WITH_KNOTS('',3,(#91757,#91758,#91759,#91760,#91761,
#91762,#91763,#91764,#91765,#91766,#91767,#91768,#91769,#91770,#91771,#91772,
#91773,#91774,#91775,#91776,#91777,#91778,#91779,#91780,#91781,#91782,#91783,
#91784,#91785,#91786,#91787,#91788,#91789,#91790,#91791,#91792,#91793,#91794,
#91795,#91796,#91797,#91798,#91799,#91800,#91801,#91802,#91803,#91804,#91805,
#91806,#91807,#91808,#91809,#91810,#91811,#91812,#91813,#91814,#91815,#91816,
#91817,#91818,#91819,#91820,#91821,#91822,#91823,#91824,#91825,#91826,#91827,
#91828,#91829,#91830,#91831,#91832,#91833,#91834,#91835,#91836,#91837,#91838,
#91839,#91840,#91841,#91842,#91843,#91844,#91845,#91846,#91847,#91848,#91849,
#91850,#91851,#91852,#91853,#91854,#91855,#91856,#91857,#91858,#91859,#91860,
#91861,#91862,#91863,#91864,#91865,#91866,#91867,#91868,#91869,#91870,#91871,
#91872,#91873,#91874,#91875,#91876,#91877,#91878,#91879,#91880,#91881,#91882,
#91883,#91884,#91885,#91886,#91887,#91888,#91889,#91890,#91891,#91892,#91893,
#91894,#91895,#91896,#91897,#91898,#91899,#91900,#91901,#91902,#91903,#91904,
#91905,#91906,#91907,#91908,#91909,#91910,#91911,#91912,#91913,#91914,#91915,
#91916,#91917,#91918,#91919,#91920,#91921,#91922,#91923,#91924,#91925,#91926,
#91927,#91928,#91929,#91930,#91931,#91932,#91933,#91934,#91935,#91936,#91937,
#91938,#91939,#91940,#91941,#91942,#91943,#91944,#91945,#91946,#91947,#91948,
#91949,#91950,#91951,#91952,#91953,#91954,#91955,#91956,#91957,#91958),
 .UNSPECIFIED.,.F.,.F.,(4,3,3,3,3,3,3,3,3,3,3,3,3,3,3,3,3,3,3,3,3,3,3,3,
3,3,3,3,3,3,3,3,3,3,3,3,3,3,3,3,3,3,3,3,3,3,3,3,3,3,3,3,3,3,3,3,3,3,3,3,
3,3,3,3,3,3,3,4),(0.,0.0321347663513911,0.0495590971962858,0.0642731458325224,
0.0803449852514299,0.0862931845746985,0.0964200512051668,0.10417597746563,
0.112500619108118,0.1188635453537,0.127099327263411,0.12859129060153,0.134437158235721,
0.136643239029931,0.137833345921669,0.140671729597307,0.141438649477679,
0.144702441480307,0.145881989724134,0.150173982146214,0.15277262499039,
0.153697717707011,0.156609795439022,0.156813504295751,0.157452006796345,
0.160140339175471,0.160859452487887,0.161815966934324,0.165392978618541,
0.168754753030431,0.168969990302759,0.172572893113886,0.173035427576006,
0.17347524133991,0.174874914476304,0.175070484733593,0.17525292917978,0.175430745909724,
0.176752761166982,0.177106662985369,0.177544810746771,0.180196510508637,
0.182865217339906,0.185255162170942,0.187290885676172,0.188723430659198,
0.189325249765294,0.191782738213962,0.193388999062593,0.196260696109834,
0.199201866293497,0.201293287365534,0.201495395322362,0.203648653252632,
0.205190626206137,0.20553912739097,0.208511013889035,0.20957779685043,0.213946752682742,
0.217643568734126,0.2230677928992,0.22569846278186,0.23234312451842,0.233746180692591,
0.24011738396337,0.24178905493371,0.25264345913106,0.257865728390371),
 .UNSPECIFIED.);
#2259=B_SPLINE_CURVE_WITH_KNOTS('',3,(#92094,#92095,#92096,#92097,#92098,
#92099,#92100,#92101,#92102,#92103,#92104,#92105,#92106,#92107,#92108,#92109,
#92110,#92111,#92112,#92113,#92114,#92115,#92116,#92117,#92118,#92119,#92120,
#92121,#92122,#92123,#92124,#92125,#92126,#92127,#92128,#92129,#92130,#92131,
#92132,#92133,#92134,#92135,#92136,#92137,#92138,#92139,#92140,#92141,#92142,
#92143,#92144,#92145,#92146,#92147,#92148,#92149,#92150,#92151,#92152,#92153,
#92154,#92155,#92156,#92157,#92158,#92159,#92160,#92161,#92162,#92163,#92164,
#92165,#92166,#92167,#92168,#92169,#92170,#92171,#92172,#92173,#92174,#92175,
#92176,#92177,#92178,#92179,#92180,#92181,#92182,#92183,#92184,#92185,#92186,
#92187,#92188,#92189,#92190,#92191,#92192,#92193,#92194,#92195,#92196,#92197,
#92198,#92199,#92200,#92201,#92202,#92203,#92204,#92205,#92206,#92207,#92208,
#92209,#92210,#92211,#92212,#92213,#92214,#92215,#92216,#92217,#92218,#92219,
#92220,#92221,#92222,#92223,#92224,#92225,#92226,#92227,#92228,#92229,#92230,
#92231,#92232,#92233,#92234,#92235,#92236,#92237,#92238,#92239,#92240,#92241,
#92242,#92243,#92244,#92245,#92246,#92247,#92248,#92249,#92250,#92251,#92252,
#92253,#92254,#92255,#92256,#92257,#92258,#92259,#92260,#92261,#92262,#92263,
#92264,#92265,#92266,#92267,#92268,#92269,#92270,#92271,#92272,#92273,#92274,
#92275,#92276,#92277,#92278,#92279,#92280,#92281,#92282,#92283,#92284,#92285,
#92286,#92287,#92288,#92289,#92290,#92291,#92292,#92293,#92294,#92295,#92296,
#92297,#92298,#92299,#92300,#92301,#92302,#92303,#92304,#92305,#92306,#92307,
#92308,#92309,#92310,#92311,#92312,#92313,#92314,#92315,#92316,#92317,#92318,
#92319,#92320,#92321,#92322,#92323,#92324,#92325,#92326,#92327,#92328,#92329,
#92330,#92331,#92332,#92333,#92334,#92335,#92336,#92337,#92338,#92339,#92340,
#92341,#92342,#92343),.UNSPECIFIED.,.F.,.F.,(4,3,3,3,3,3,3,3,3,3,3,3,3,
3,3,3,3,3,3,3,3,3,3,3,3,3,3,3,3,3,3,3,3,3,3,3,3,3,3,3,3,3,3,3,3,3,3,3,3,
3,3,3,3,3,3,3,3,3,3,3,3,3,3,3,3,3,3,3,3,3,3,3,3,3,3,3,3,3,3,3,3,3,3,4),
(-5.99999999961901E-8,0.00205213753470555,0.00346047691825982,0.00549976480516702,
0.00684933075492668,0.00692828170882304,0.00947037504164401,0.0116737828388313,
0.0127754867374249,0.0134477508061639,0.0137277075245536,0.0138771906360185,
0.0147454865964315,0.0152762362074286,0.0156228660994763,0.0176161119027071,
0.0192198351110147,0.0202986140975471,0.0208235583193224,0.0225611142429988,
0.0236071707918062,0.0239227132772834,0.0242885895794692,0.025152866209584,
0.0255712676146208,0.0266029893184477,0.0268886660138179,0.0271218002136788,
0.0272592346694993,0.0277456960999287,0.0299580577697661,0.032296502762021,
0.0335558689820468,0.0343992850002989,0.0346349477542758,0.0377731272866975,
0.040976446705338,0.0414941580473473,0.0449116181533913,0.0473261513120718,
0.0480896243204303,0.0483290782594353,0.0500331936258331,0.0510138895980884,
0.0534411134522563,0.0551455397250265,0.0597641814744442,0.0642522681203356,
0.0665629408104305,0.0677395126638232,0.0685561850589512,0.068740354766227,
0.0721325097284016,0.073828587209489,0.0746119055671886,0.0750773246746244,
0.0755246646905763,0.0789136615920156,0.0808492608585523,0.082302658493455,
0.0899824409819067,0.095845006466064,0.102609655818586,0.106117423701975,
0.108183528611815,0.109374305171108,0.116134326690507,0.119525294284937,
0.122087358326956,0.122894348209906,0.12964774211714,0.133677826490132,
0.136177104645105,0.136401136024373,0.147704077365847,0.15553974506886,
0.159457578920367,0.161717990371485,0.163099656918869,0.163375412771874,
0.181117111195966,0.190331075834418,0.210237730720008,0.217279461675811),
 .UNSPECIFIED.);
#2260=B_SPLINE_CURVE_WITH_KNOTS('',3,(#92344,#92345,#92346,#92347,#92348,
#92349,#92350,#92351,#92352,#92353,#92354,#92355,#92356,#92357,#92358,#92359,
#92360,#92361,#92362,#92363,#92364,#92365,#92366,#92367,#92368,#92369,#92370,
#92371,#92372,#92373,#92374,#92375,#92376,#92377,#92378,#92379,#92380,#92381,
#92382,#92383,#92384,#92385,#92386,#92387,#92388,#92389,#92390,#92391,#92392,
#92393,#92394,#92395,#92396,#92397,#92398,#92399,#92400,#92401,#92402,#92403,
#92404,#92405,#92406,#92407),.UNSPECIFIED.,.F.,.F.,(4,3,3,3,3,3,3,3,3,3,
3,3,3,3,3,3,3,3,3,3,3,4),(0.,0.0265419162547455,0.0530838325094911,0.0796257487642366,
0.0928967068916094,0.106167665018982,0.119438623146355,0.132709581273728,
0.139345060337414,0.145980539401101,0.159251497528473,0.16588697659216,
0.172522455655846,0.179157934719533,0.185793413783219,0.189111153315062,
0.192428892846905,0.199064371910592,0.205699850974278,0.209017590506122,
0.21076098823351,0.212335330037965),.UNSPECIFIED.);
#2261=B_SPLINE_CURVE_WITH_KNOTS('',3,(#92447,#92448,#92449,#92450,#92451,
#92452,#92453,#92454,#92455,#92456,#92457,#92458,#92459,#92460,#92461,#92462,
#92463,#92464,#92465,#92466,#92467,#92468,#92469,#92470,#92471,#92472,#92473,
#92474,#92475,#92476,#92477,#92478,#92479,#92480,#92481,#92482,#92483,#92484,
#92485,#92486,#92487,#92488,#92489),.UNSPECIFIED.,.F.,.F.,(4,3,3,3,3,3,
3,3,3,3,3,3,3,3,4),(0.,0.0174818147702963,0.0276661561951365,0.0466085742141883,
0.0553487132947371,0.0706615640779338,0.083047726575705,0.0850821797454832,
0.0909913302116415,0.0939459054447206,0.0954294830608625,0.0964768515157899,
0.0969004806777997,0.107725903082733,0.110740358368174),.UNSPECIFIED.);
#2262=B_SPLINE_CURVE_WITH_KNOTS('',3,(#92490,#92491,#92492,#92493,#92494,
#92495,#92496,#92497,#92498,#92499,#92500,#92501,#92502,#92503,#92504,#92505,
#92506,#92507,#92508,#92509,#92510,#92511,#92512,#92513,#92514,#92515,#92516,
#92517,#92518,#92519,#92520,#92521,#92522,#92523),.UNSPECIFIED.,.F.,.F.,
(4,3,3,3,3,3,3,3,3,3,3,4),(0.,0.00853528476678784,0.0138219837281452,0.0138424585775806,
0.0212354389568398,0.0276642139270636,0.0276849171551612,0.0553560321602673,
0.0553698343103225,0.0830478503904525,0.0830547514654838,0.110739668620645),
 .UNSPECIFIED.);
#2263=B_SPLINE_CURVE_WITH_KNOTS('',3,(#92587,#92588,#92589,#92590,#92591,
#92592,#92593,#92594,#92595,#92596,#92597,#92598,#92599,#92600,#92601,#92602,
#92603,#92604,#92605,#92606,#92607,#92608,#92609,#92610,#92611,#92612,#92613,
#92614,#92615,#92616,#92617,#92618,#92619,#92620,#92621,#92622,#92623,#92624,
#92625,#92626,#92627,#92628,#92629,#92630,#92631,#92632,#92633,#92634,#92635,
#92636,#92637,#92638,#92639,#92640,#92641,#92642,#92643,#92644,#92645,#92646,
#92647,#92648,#92649,#92650,#92651,#92652,#92653,#92654,#92655,#92656,#92657,
#92658,#92659,#92660,#92661,#92662),.UNSPECIFIED.,.F.,.F.,(4,3,3,3,3,3,
3,3,3,3,3,3,3,3,3,3,3,3,3,3,3,3,3,3,3,4),(2.00078531959267E-15,6.27245974407096E-5,
0.00012523366663523,0.000168194487246218,0.000208019821857731,0.000263919656744897,
0.000292924598205694,0.000363889403564607,0.000377194267852935,0.000453363357768638,
0.000533936193646606,0.000576783819641349,0.000670776831385002,0.000735149291962565,
0.000856545197961509,0.000932596455777723,0.00105992985614175,0.00120019572685142,
0.00131573376212713,0.00147029858392507,0.00170701877802783,0.00195809484060081,
0.00211995765409861,0.00220544787588757,0.00284725701195324,0.00294057482639061),
 .UNSPECIFIED.);
#2264=B_SPLINE_CURVE_WITH_KNOTS('',3,(#92750,#92751,#92752,#92753,#92754,
#92755,#92756,#92757,#92758,#92759,#92760,#92761,#92762,#92763,#92764,#92765,
#92766,#92767,#92768,#92769,#92770,#92771,#92772,#92773,#92774,#92775,#92776,
#92777),.UNSPECIFIED.,.F.,.F.,(4,2,2,2,2,2,2,2,2,2,2,2,2,4),(1.73472347597681E-18,
0.00801632890443165,0.0160326578088633,0.0200408222610791,0.0240489867132949,
0.0320653156177267,0.0360734800699425,0.0380775622960505,0.0400816445221584,
0.0480979734265901,0.0501020556526981,0.052106137878806,0.0561143023310219,
0.0641306312354537),.UNSPECIFIED.);
#2265=B_SPLINE_CURVE_WITH_KNOTS('',3,(#92778,#92779,#92780,#92781,#92782,
#92783,#92784,#92785,#92786,#92787,#92788,#92789,#92790,#92791,#92792,#92793,
#92794,#92795,#92796,#92797,#92798,#92799,#92800,#92801,#92802,#92803,#92804,
#92805,#92806,#92807,#92808,#92809,#92810,#92811,#92812,#92813,#92814,#92815,
#92816,#92817,#92818,#92819,#92820,#92821,#92822,#92823,#92824,#92825,#92826,
#92827,#92828,#92829,#92830,#92831,#92832,#92833,#92834,#92835,#92836,#92837,
#92838,#92839,#92840,#92841,#92842,#92843,#92844,#92845,#92846,#92847,#92848,
#92849,#92850,#92851,#92852,#92853,#92854,#92855,#92856,#92857,#92858,#92859,
#92860,#92861,#92862,#92863,#92864,#92865,#92866,#92867,#92868,#92869,#92870,
#92871),.UNSPECIFIED.,.F.,.F.,(4,3,3,3,3,3,3,3,3,3,3,3,3,3,3,3,3,3,3,3,
3,3,3,3,3,3,3,3,3,3,3,4),(0.,0.00674763364146324,0.00782968911952726,0.00784373710529933,
0.0117445336792909,0.0117656056534845,0.0137019559591727,0.0137265401335389,
0.0156593782390545,0.0156874742092816,0.0234890673585819,0.0235312113204749,
0.0254464896384637,0.0254921454471888,0.0274039119183456,0.0274530829252165,
0.0303049604471932,0.0313187564781093,0.0313749484131831,0.0391484455976365,
0.0392186860654585,0.0416267378991184,0.0430632901574002,0.0431404818311709,
0.0469781347171638,0.0470560909016423,0.0506039903695911,0.0542607409119146,
0.0548078238366911,0.0548609217456285,0.0590992763654095,0.0626375129562184),
 .UNSPECIFIED.);
#2266=B_SPLINE_CURVE_WITH_KNOTS('',3,(#92921,#92922,#92923,#92924,#92925,
#92926,#92927,#92928,#92929,#92930,#92931,#92932,#92933,#92934,#92935,#92936,
#92937,#92938,#92939,#92940,#92941,#92942,#92943,#92944,#92945,#92946,#92947,
#92948,#92949,#92950,#92951,#92952,#92953,#92954,#92955,#92956,#92957,#92958,
#92959,#92960,#92961,#92962,#92963,#92964,#92965,#92966,#92967,#92968,#92969,
#92970,#92971,#92972,#92973,#92974,#92975,#92976,#92977,#92978,#92979,#92980,
#92981,#92982,#92983,#92984,#92985,#92986,#92987,#92988,#92989,#92990,#92991,
#92992,#92993),.UNSPECIFIED.,.F.,.F.,(4,3,3,3,3,3,3,3,3,3,3,3,3,3,3,3,3,
3,3,3,3,3,3,3,4),(2.53193767630367E-8,0.000761602148823654,0.000848295295233062,
0.00109951708486985,0.00132392636131809,0.0015232042976473,0.00168207255245941,
0.00185215920385473,0.00190400537205915,0.00204222878317895,0.00217140981375754,
0.00228480644647099,0.00238367032878988,0.00244986162048359,0.0025321966759578,
0.00260949404176403,0.00266560752088284,0.00272802392810674,0.00276080778948581,
0.0027758345451979,0.00282959836697759,0.00285600805808879,0.00290360819239027,
0.00297598425714359,0.00304640859529444),.UNSPECIFIED.);
#2267=B_SPLINE_CURVE_WITH_KNOTS('',3,(#93054,#93055,#93056,#93057,#93058,
#93059,#93060,#93061,#93062,#93063,#93064,#93065,#93066,#93067,#93068,#93069,
#93070,#93071,#93072,#93073,#93074,#93075,#93076,#93077,#93078,#93079,#93080,
#93081,#93082,#93083,#93084,#93085,#93086,#93087,#93088,#93089,#93090),
 .UNSPECIFIED.,.F.,.F.,(4,3,3,3,3,3,3,3,3,3,3,3,4),(1.83990108477198E-9,
0.000128387533529865,0.00025794985788125,0.000364723131813831,0.000364936417772228,
0.000547613913069482,0.000729446263627662,0.000730277175766961,0.000912528804080312,
0.00109439518681158,0.00127664385703345,0.00144798651104331,0.00145889252725532),
 .UNSPECIFIED.);
#2268=B_SPLINE_CURVE_WITH_KNOTS('',3,(#93109,#93110,#93111,#93112,#93113,
#93114,#93115),.UNSPECIFIED.,.F.,.F.,(4,3,4),(2.41016821063581E-15,0.00262158494557133,
0.00335832469594566),.UNSPECIFIED.);
#2269=B_SPLINE_CURVE_WITH_KNOTS('',3,(#93142,#93143,#93144,#93145,#93146,
#93147,#93148,#93149,#93150,#93151,#93152,#93153,#93154,#93155,#93156,#93157,
#93158,#93159,#93160,#93161,#93162,#93163,#93164,#93165,#93166,#93167,#93168,
#93169,#93170,#93171,#93172,#93173,#93174,#93175,#93176,#93177,#93178,#93179,
#93180,#93181),.UNSPECIFIED.,.F.,.F.,(4,3,3,3,3,3,3,3,3,3,3,3,3,4),(4.75463922286045E-13,
0.000114874771772721,0.000233668770413462,0.00035889395548095,0.000488266865941692,
0.000623835778388218,0.000646036121242161,0.000676434176771284,0.000814383672645379,
0.00095995065267877,0.000993298115721985,0.00115816801506027,0.00133156200529955,
0.00135286835354256),.UNSPECIFIED.);
#2270=B_SPLINE_CURVE_WITH_KNOTS('',3,(#93273,#93274,#93275,#93276,#93277,
#93278,#93279,#93280,#93281,#93282,#93283,#93284,#93285,#93286,#93287,#93288,
#93289,#93290,#93291,#93292,#93293,#93294,#93295,#93296,#93297,#93298,#93299,
#93300,#93301,#93302,#93303,#93304,#93305,#93306,#93307,#93308,#93309,#93310,
#93311,#93312,#93313,#93314,#93315,#93316,#93317,#93318,#93319,#93320,#93321,
#93322,#93323,#93324,#93325,#93326,#93327,#93328,#93329,#93330,#93331,#93332,
#93333,#93334,#93335,#93336,#93337,#93338,#93339,#93340,#93341,#93342,#93343,
#93344,#93345,#93346,#93347,#93348,#93349,#93350,#93351,#93352,#93353,#93354,
#93355,#93356,#93357),.UNSPECIFIED.,.F.,.F.,(4,3,3,3,3,3,3,3,3,3,3,3,3,
3,3,3,3,3,3,3,3,3,3,3,3,3,3,3,4),(1.04083408558608E-17,0.00306132087462231,
0.00458763228313725,0.00505755460700053,0.00737727473051059,0.00758657165052886,
0.0091752645662745,0.0101149087127913,0.0114690807078431,0.0137628968494117,
0.0151702835088379,0.0176976693841385,0.0183505291325489,0.0189612134424709,
0.0202246504480127,0.0206443452741175,0.0227077461535235,0.0229381614156862,
0.0252770618598094,0.0275257936988233,0.0278023764522136,0.0290648438726516,
0.0298196098403919,0.0303268301110632,0.0318006663681232,0.0321134259819605,
0.0348081739351341,0.0353740968812584,0.0367010582650977),.UNSPECIFIED.);
#2271=B_SPLINE_CURVE_WITH_KNOTS('',3,(#93396,#93397,#93398,#93399,#93400,
#93401,#93402,#93403,#93404,#93405,#93406,#93407,#93408,#93409,#93410,#93411,
#93412,#93413,#93414,#93415,#93416,#93417,#93418,#93419,#93420,#93421,#93422,
#93423,#93424,#93425,#93426),.UNSPECIFIED.,.F.,.F.,(4,3,3,3,3,3,3,3,3,3,
4),(1.38777878078145E-17,0.00369677025853092,0.00369698575261873,0.00739308614352542,
0.00739397150523745,0.00924116752762853,0.00924246438154679,0.0110896622905033,
0.0110909572578561,0.0145604524022874,0.0147879430104749),.UNSPECIFIED.);
#2272=B_SPLINE_CURVE_WITH_KNOTS('',3,(#93518,#93519,#93520,#93521,#93522,
#93523,#93524,#93525,#93526,#93527,#93528,#93529,#93530,#93531,#93532,#93533,
#93534,#93535,#93536,#93537,#93538,#93539,#93540,#93541,#93542,#93543,#93544,
#93545,#93546,#93547,#93548,#93549,#93550,#93551,#93552,#93553,#93554,#93555,
#93556,#93557,#93558,#93559,#93560,#93561,#93562,#93563,#93564,#93565,#93566,
#93567,#93568,#93569,#93570,#93571,#93572,#93573,#93574,#93575,#93576,#93577,
#93578,#93579,#93580,#93581,#93582,#93583,#93584,#93585,#93586,#93587,#93588,
#93589,#93590),.UNSPECIFIED.,.F.,.F.,(4,3,3,3,3,3,3,3,3,3,3,3,3,3,3,3,3,
3,3,3,3,3,3,3,4),(0.0483087273746794,0.0483353046476464,0.0499595272800289,
0.0502196409139219,0.0516103271853785,0.052103792003993,0.0549119269960775,
0.0558715388891371,0.0575187227537936,0.0577552750749259,0.0582135268067766,
0.0592308700721096,0.0596389008572866,0.0598643267121261,0.0615151266174756,
0.063406623077028,0.0671759109819169,0.0681183262388737,0.0690610075966447,
0.0697691261442232,0.0708751300026104,0.0709471315103791,0.0714199260495728,
0.0743329760918185,0.0747215258602685),.UNSPECIFIED.);
#2273=B_SPLINE_CURVE_WITH_KNOTS('',3,(#93752,#93753,#93754,#93755,#93756,
#93757,#93758,#93759,#93760,#93761,#93762,#93763,#93764,#93765,#93766,#93767,
#93768,#93769,#93770,#93771,#93772,#93773,#93774,#93775,#93776,#93777,#93778,
#93779,#93780,#93781,#93782,#93783,#93784,#93785,#93786,#93787,#93788,#93789,
#93790,#93791,#93792,#93793,#93794,#93795,#93796,#93797,#93798,#93799,#93800,
#93801,#93802,#93803,#93804,#93805,#93806,#93807,#93808,#93809,#93810,#93811,
#93812,#93813,#93814,#93815,#93816,#93817,#93818,#93819,#93820,#93821,#93822,
#93823,#93824,#93825,#93826,#93827,#93828,#93829,#93830,#93831,#93832,#93833,
#93834,#93835,#93836,#93837,#93838,#93839,#93840,#93841,#93842,#93843,#93844,
#93845,#93846,#93847,#93848,#93849,#93850,#93851,#93852,#93853,#93854,#93855,
#93856,#93857,#93858,#93859,#93860,#93861,#93862,#93863,#93864,#93865,#93866,
#93867,#93868,#93869,#93870,#93871,#93872,#93873,#93874,#93875,#93876,#93877,
#93878,#93879,#93880,#93881,#93882,#93883,#93884,#93885,#93886,#93887,#93888,
#93889,#93890,#93891,#93892,#93893,#93894,#93895,#93896,#93897,#93898,#93899,
#93900,#93901,#93902,#93903,#93904,#93905,#93906,#93907,#93908,#93909,#93910,
#93911,#93912,#93913,#93914,#93915,#93916,#93917,#93918,#93919,#93920,#93921,
#93922,#93923,#93924,#93925,#93926,#93927,#93928,#93929,#93930,#93931,#93932,
#93933,#93934,#93935,#93936,#93937,#93938,#93939,#93940,#93941,#93942,#93943,
#93944,#93945,#93946,#93947,#93948,#93949,#93950,#93951,#93952,#93953,#93954,
#93955,#93956,#93957,#93958,#93959,#93960,#93961,#93962,#93963,#93964,#93965),
 .UNSPECIFIED.,.F.,.F.,(4,3,3,3,3,3,3,3,3,3,3,3,3,3,3,3,3,3,3,3,3,3,3,3,
3,3,3,3,3,3,3,3,3,3,3,3,3,3,3,3,3,3,3,3,3,3,3,3,3,3,3,3,3,3,3,3,3,3,3,3,
3,3,3,3,3,3,3,3,3,3,3,4),(0.,0.0016184602718221,0.00319828590087957,0.004726552519676,
0.0062296665305914,0.00624571575272172,0.0077129297625436,0.00780714469090215,
0.00780777507546303,0.00880374169768939,0.00936857362908258,0.00939497775797128,
0.0110637108063712,0.0124914315054434,0.0125796213647023,0.014886037330468,
0.0172473351707312,0.0187371472581651,0.0189513025431913,0.0199039933520977,
0.0202985761963456,0.0213604955378055,0.021860005134526,0.0221313353710413,
0.023934479755877,0.0249828630108868,0.0253066784590323,0.0290723120433818,
0.0312285787636085,0.0316436340020624,0.0332250107158749,0.0343514366399693,
0.0348052706445514,0.0374742945163301,0.0379625216831405,0.0417199791548649,
0.0437200102690518,0.0442643097824748,0.0482414580560455,0.0499657260217734,
0.0505499917372572,0.0530885838981343,0.053687282245013,0.0562114417744951,
0.0568213808126068,0.0613502593264657,0.0624571575272168,0.0630810366667805,
0.0680308152815377,0.0687028732799386,0.0693306751795749,0.0735190343863351,
0.0749485890326603,0.0755720956952829,0.0811367906296009,0.0871241069005245,
0.0874400205381038,0.0880368539666603,0.0960156407501182,0.0999314520435472,
0.100484493326179,0.110352684692032,0.112422883548991,0.112920779842532,
0.124914315054434,0.125349598801627,0.142221446158236,0.149897178065321,
0.150194407331914,0.174880041076208,0.175030605012004,0.199862904087095),
 .UNSPECIFIED.);
#2274=B_SPLINE_CURVE_WITH_KNOTS('',3,(#93968,#93969,#93970,#93971,#93972,
#93973,#93974,#93975,#93976,#93977,#93978,#93979,#93980,#93981,#93982,#93983,
#93984,#93985,#93986,#93987,#93988,#93989,#93990,#93991,#93992,#93993,#93994,
#93995,#93996,#93997,#93998,#93999,#94000,#94001,#94002,#94003,#94004,#94005,
#94006,#94007,#94008,#94009,#94010,#94011,#94012,#94013,#94014,#94015,#94016,
#94017,#94018,#94019,#94020,#94021,#94022,#94023,#94024,#94025,#94026,#94027,
#94028,#94029,#94030,#94031,#94032,#94033,#94034,#94035,#94036,#94037,#94038,
#94039,#94040,#94041,#94042,#94043,#94044,#94045,#94046,#94047,#94048,#94049,
#94050,#94051,#94052,#94053,#94054,#94055,#94056,#94057,#94058,#94059,#94060,
#94061,#94062,#94063,#94064,#94065,#94066,#94067,#94068,#94069,#94070,#94071,
#94072,#94073,#94074,#94075,#94076,#94077,#94078,#94079,#94080,#94081,#94082,
#94083,#94084,#94085,#94086,#94087,#94088,#94089,#94090,#94091,#94092,#94093,
#94094,#94095,#94096,#94097,#94098,#94099,#94100,#94101,#94102,#94103,#94104,
#94105,#94106,#94107,#94108,#94109,#94110,#94111,#94112,#94113,#94114,#94115,
#94116,#94117,#94118,#94119,#94120,#94121,#94122,#94123,#94124,#94125,#94126,
#94127,#94128,#94129,#94130,#94131,#94132,#94133,#94134,#94135,#94136,#94137,
#94138,#94139,#94140,#94141,#94142),.UNSPECIFIED.,.F.,.F.,(4,3,3,3,3,3,
3,3,3,3,3,3,3,3,3,3,3,3,3,3,3,3,3,3,3,3,3,3,3,3,3,3,3,3,3,3,3,3,3,3,3,3,
3,3,3,3,3,3,3,3,3,3,3,3,3,3,3,3,4),(0.,0.0246446543849258,0.0246541408539193,
0.0492893087698515,0.0493082813931077,0.0739339631547773,0.0739624219187268,
0.0862562903472402,0.0862894922015488,0.0985786175397031,0.0986165624711814,
0.110900944732166,0.110943632741705,0.123223271924629,0.123270703016623,
0.12938443552086,0.129434238115484,0.135545599117092,0.135597773279537,
0.141706762713323,0.141761308417236,0.144787344511439,0.144843075947332,
0.147867926309555,0.147924844511973,0.15366260629182,0.154029089905786,
0.154088378680815,0.160190253502018,0.160251913829296,0.163270835300134,
0.163333681393769,0.164811126199191,0.164874564889871,0.166351417098249,
0.166415452062168,0.170160979779983,0.17251258069448,0.172578984095756,
0.175593162492596,0.175660751383538,0.177765246175035,0.178673744290712,
0.178742525402502,0.181788716644722,0.184834907886943,0.184906054338471,
0.187915489685058,0.187987822676343,0.189057434582198,0.189455780584116,
0.189527858303638,0.190809262316065,0.190996071483174,0.191062726298861,
0.192788975213052,0.194560412577886,0.196416249655382,0.197157235079405),
 .UNSPECIFIED.);
#2275=B_SPLINE_CURVE_WITH_KNOTS('',3,(#94188,#94189,#94190,#94191,#94192,
#94193,#94194,#94195,#94196,#94197,#94198,#94199,#94200,#94201,#94202,#94203,
#94204,#94205,#94206,#94207,#94208,#94209,#94210,#94211,#94212,#94213,#94214,
#94215,#94216,#94217,#94218,#94219,#94220,#94221,#94222,#94223,#94224,#94225,
#94226,#94227,#94228,#94229,#94230,#94231,#94232,#94233,#94234,#94235,#94236,
#94237,#94238,#94239,#94240,#94241,#94242,#94243,#94244,#94245,#94246,#94247,
#94248,#94249,#94250,#94251,#94252,#94253,#94254,#94255,#94256,#94257,#94258,
#94259,#94260,#94261,#94262,#94263,#94264,#94265,#94266),.UNSPECIFIED.,
 .F.,.F.,(4,3,3,3,3,3,3,3,3,3,3,3,3,3,3,3,3,3,3,3,3,3,3,3,3,3,4),(0.,0.000336250842231429,
0.000672501684462858,0.000787345219381404,0.000973846749200159,0.00114945806151638,
0.0013133825161952,0.00134500336892572,0.00148679920422429,0.00153267447151819,
0.00165410437577115,0.00168125421115719,0.00178334395389124,0.00187375941124646,
0.00197323383655314,0.00201750505338867,0.00209923935339125,0.00218097365339383,
0.00225620497656911,0.00232840090118059,0.00235375589562014,0.00242936444625713,
0.00244707680874984,0.00251502720952607,0.0025826808988154,0.00265019823541125,
0.00269000673785162),.UNSPECIFIED.);
#2276=B_SPLINE_CURVE_WITH_KNOTS('',3,(#94267,#94268,#94269,#94270,#94271,
#94272,#94273,#94274,#94275,#94276,#94277,#94278,#94279,#94280),
 .UNSPECIFIED.,.F.,.F.,(4,2,2,2,2,2,4),(0.,0.000499758886231802,0.000999517772463604,
0.00149927665869541,0.00199903554492721,0.00299855331739082,0.00399807108985443),
 .UNSPECIFIED.);
#2277=B_SPLINE_CURVE_WITH_KNOTS('',3,(#94317,#94318,#94319,#94320,#94321,
#94322,#94323,#94324,#94325,#94326,#94327,#94328,#94329,#94330,#94331,#94332,
#94333,#94334,#94335,#94336,#94337,#94338,#94339,#94340,#94341,#94342,#94343,
#94344),.UNSPECIFIED.,.F.,.F.,(4,3,3,3,3,3,3,3,3,4),(0.102333040030003,
0.113924927639759,0.114433131497043,0.126097619555127,0.126533222964083,
0.150443003704343,0.150733405898164,0.174788387734704,0.174933588832244,
0.199133771766325),.UNSPECIFIED.);
#2278=B_SPLINE_CURVE_WITH_KNOTS('',3,(#94345,#94346,#94347,#94348,#94349,
#94350,#94351,#94352,#94353,#94354,#94355,#94356),.UNSPECIFIED.,.F.,.F.,
(4,2,2,2,2,4),(6.16297582203915E-33,0.0239358211212684,0.0478716422425369,
0.0718074633638053,0.0837753739244396,0.0957432844850738),.UNSPECIFIED.);
#2279=B_SPLINE_CURVE_WITH_KNOTS('',3,(#94426,#94427,#94428,#94429,#94430,
#94431,#94432,#94433,#94434,#94435,#94436,#94437,#94438,#94439,#94440,#94441,
#94442,#94443,#94444,#94445,#94446,#94447,#94448,#94449,#94450,#94451,#94452,
#94453,#94454,#94455,#94456,#94457,#94458,#94459,#94460,#94461,#94462,#94463,
#94464,#94465,#94466,#94467,#94468,#94469,#94470,#94471,#94472,#94473,#94474,
#94475,#94476,#94477,#94478,#94479,#94480,#94481,#94482,#94483,#94484,#94485,
#94486,#94487,#94488,#94489,#94490,#94491,#94492,#94493,#94494,#94495,#94496,
#94497,#94498,#94499,#94500,#94501,#94502,#94503,#94504,#94505,#94506,#94507),
 .UNSPECIFIED.,.F.,.F.,(4,3,3,3,3,3,3,3,3,3,3,3,3,3,3,3,3,3,3,3,3,3,3,3,
3,3,3,4),(0.,0.000336813957898486,0.000673627915796972,0.000788294450931827,
0.000965405233874476,0.0011241828986832,0.00117000317678504,0.00133401990639404,
0.00134725583159394,0.00149483781156424,0.00153477011657144,0.00165318596336469,
0.00168406978949244,0.00178416166633809,0.00187612406911513,0.00197204161846305,
0.00202088374739094,0.00210969879246536,0.00218359020102549,0.00227031653218695,
0.00231573286521894,0.00235731345133549,0.0023805412898631,0.00245198186431492,
0.00252610468423863,0.00259198145108106,0.00265777781837003,0.00269451166318783),
 .UNSPECIFIED.);
#2280=B_SPLINE_CURVE_WITH_KNOTS('',3,(#94510,#94511,#94512,#94513,#94514,
#94515,#94516,#94517,#94518,#94519,#94520,#94521,#94522,#94523,#94524,#94525,
#94526,#94527,#94528,#94529,#94530,#94531,#94532,#94533,#94534,#94535,#94536,
#94537,#94538,#94539,#94540,#94541,#94542,#94543,#94544,#94545,#94546,#94547,
#94548,#94549,#94550,#94551,#94552,#94553,#94554,#94555,#94556,#94557,#94558,
#94559,#94560,#94561,#94562,#94563,#94564,#94565,#94566,#94567,#94568,#94569,
#94570),.UNSPECIFIED.,.F.,.F.,(4,3,3,3,3,3,3,3,3,3,3,3,3,3,3,3,3,3,3,3,
4),(0.,0.000740904719734282,0.000992426177924283,0.000994381157584888,0.00134969342662063,
0.00148863926688639,0.00149340155200891,0.00198485235584851,0.00199238270471871,
0.00229592938464614,0.00249083959038169,0.00275696980167887,0.00297727853377274,
0.00298709774675677,0.00319310808437571,0.00338978198634247,0.00347349162273481,
0.00348023433971105,0.00372496952570397,0.00395655830428439,0.00396970471169688),
 .UNSPECIFIED.);
#2281=B_SPLINE_CURVE_WITH_KNOTS('',3,(#94670,#94671,#94672,#94673,#94674,
#94675,#94676,#94677,#94678,#94679,#94680,#94681,#94682,#94683,#94684,#94685,
#94686,#94687,#94688,#94689,#94690,#94691,#94692,#94693,#94694,#94695,#94696,
#94697,#94698,#94699,#94700,#94701,#94702,#94703,#94704,#94705,#94706,#94707,
#94708,#94709,#94710,#94711,#94712,#94713,#94714,#94715),.UNSPECIFIED.,
 .F.,.F.,(4,3,3,3,3,3,3,3,3,3,3,3,3,3,3,4),(0.,0.0056591289497744,0.00848869342466156,
0.0113182578995487,0.0226365157990974,0.033954773698646,0.0396139026484203,
0.0452730315981947,0.0565912894977434,0.0679095473972921,0.0905460631963896,
0.101864321095938,0.113182578995487,0.135819094794585,0.158455610593682,
0.18109212639278),.UNSPECIFIED.);
#2282=B_SPLINE_CURVE_WITH_KNOTS('',3,(#94716,#94717,#94718,#94719,#94720,
#94721,#94722,#94723,#94724,#94725,#94726,#94727,#94728,#94729,#94730,#94731,
#94732,#94733,#94734,#94735,#94736,#94737,#94738,#94739,#94740,#94741,#94742,
#94743,#94744,#94745),.UNSPECIFIED.,.F.,.F.,(4,2,2,2,2,2,2,2,2,2,2,2,2,
2,4),(0.,0.0225170076686272,0.0450340153372545,0.0675510230058817,0.0788095268401953,
0.0900680306745089,0.112585038343136,0.12384354217745,0.135102046011763,
0.146360549846077,0.15761905368039,0.168877557514704,0.171692183473282,
0.174506809431861,0.180136061349017),.UNSPECIFIED.);
#2283=B_SPLINE_CURVE_WITH_KNOTS('',3,(#94793,#94794,#94795,#94796,#94797,
#94798,#94799,#94800,#94801,#94802,#94803,#94804,#94805,#94806,#94807,#94808,
#94809,#94810,#94811,#94812,#94813,#94814,#94815,#94816,#94817,#94818,#94819,
#94820),.UNSPECIFIED.,.F.,.F.,(4,3,3,3,3,3,3,3,3,4),(0.152124875880697,
0.156978231818529,0.158991212459818,0.164515562446826,0.165857549038938,
0.170542889642604,0.172052891500496,0.172723885618059,0.177134015604045,
0.17959022219718),.UNSPECIFIED.);
#2284=B_SPLINE_CURVE_WITH_KNOTS('',3,(#94821,#94822,#94823,#94824,#94825,
#94826,#94827,#94828,#94829,#94830),.UNSPECIFIED.,.F.,.F.,(4,2,2,2,4),(6.20633538311818E-17,
0.00753427253238126,0.0150685450647625,0.0226028175971437,0.0301370901295249),
 .UNSPECIFIED.);
#2285=B_SPLINE_CURVE_WITH_KNOTS('',3,(#94834,#94835,#94836,#94837,#94838,
#94839,#94840,#94841,#94842,#94843,#94844,#94845,#94846,#94847,#94848,#94849,
#94850,#94851,#94852,#94853,#94854,#94855,#94856,#94857,#94858,#94859,#94860,
#94861,#94862,#94863,#94864),.UNSPECIFIED.,.F.,.F.,(4,3,3,3,3,3,3,3,3,3,
4),(0.,0.0270705423331218,0.0278297418200406,0.0541410846662436,0.0556594833976957,
0.0812116269993654,0.083489181931652,0.0930720176545818,0.0947468981659263,
0.0974041311753799,0.108282169332487),.UNSPECIFIED.);
#2286=B_SPLINE_CURVE_WITH_KNOTS('',3,(#95223,#95224,#95225,#95226,#95227,
#95228,#95229,#95230,#95231,#95232,#95233,#95234,#95235,#95236,#95237,#95238,
#95239,#95240,#95241,#95242,#95243,#95244,#95245,#95246,#95247,#95248,#95249,
#95250,#95251,#95252,#95253,#95254,#95255,#95256,#95257,#95258,#95259,#95260,
#95261,#95262,#95263,#95264,#95265,#95266,#95267,#95268,#95269,#95270,#95271,
#95272,#95273,#95274,#95275,#95276,#95277,#95278,#95279,#95280,#95281,#95282,
#95283,#95284,#95285,#95286,#95287,#95288,#95289,#95290,#95291,#95292,#95293,
#95294,#95295,#95296,#95297,#95298,#95299,#95300,#95301,#95302,#95303,#95304,
#95305,#95306,#95307,#95308,#95309,#95310,#95311,#95312,#95313,#95314,#95315,
#95316,#95317,#95318,#95319,#95320,#95321,#95322,#95323,#95324,#95325,#95326,
#95327,#95328,#95329,#95330,#95331,#95332,#95333,#95334,#95335,#95336,#95337,
#95338,#95339,#95340,#95341,#95342,#95343,#95344,#95345,#95346,#95347,#95348,
#95349,#95350,#95351,#95352,#95353,#95354,#95355,#95356,#95357,#95358,#95359,
#95360,#95361,#95362,#95363,#95364,#95365,#95366,#95367,#95368,#95369,#95370,
#95371,#95372,#95373,#95374,#95375,#95376,#95377,#95378,#95379,#95380,#95381,
#95382,#95383,#95384,#95385,#95386,#95387,#95388,#95389,#95390,#95391,#95392,
#95393,#95394,#95395,#95396,#95397,#95398,#95399,#95400,#95401,#95402,#95403,
#95404,#95405,#95406,#95407,#95408,#95409,#95410,#95411,#95412,#95413,#95414,
#95415,#95416,#95417,#95418,#95419,#95420,#95421,#95422,#95423,#95424,#95425,
#95426,#95427,#95428,#95429,#95430,#95431,#95432,#95433,#95434,#95435,#95436,
#95437,#95438,#95439,#95440,#95441,#95442,#95443,#95444,#95445,#95446,#95447,
#95448,#95449,#95450,#95451,#95452,#95453,#95454,#95455,#95456,#95457,#95458,
#95459,#95460,#95461,#95462,#95463,#95464,#95465,#95466,#95467,#95468,#95469,
#95470,#95471,#95472,#95473,#95474,#95475,#95476,#95477,#95478,#95479,#95480,
#95481,#95482,#95483,#95484,#95485,#95486,#95487,#95488,#95489,#95490,#95491,
#95492,#95493,#95494,#95495,#95496,#95497,#95498,#95499,#95500,#95501,#95502,
#95503,#95504,#95505,#95506,#95507,#95508,#95509,#95510,#95511,#95512,#95513,
#95514,#95515,#95516,#95517,#95518,#95519,#95520,#95521,#95522,#95523,#95524,
#95525,#95526,#95527,#95528,#95529,#95530,#95531,#95532,#95533,#95534,#95535,
#95536,#95537,#95538,#95539,#95540,#95541,#95542,#95543,#95544,#95545,#95546,
#95547,#95548,#95549,#95550,#95551,#95552,#95553,#95554,#95555,#95556,#95557,
#95558,#95559,#95560,#95561,#95562,#95563,#95564,#95565,#95566,#95567,#95568,
#95569,#95570,#95571,#95572,#95573,#95574,#95575,#95576,#95577,#95578,#95579,
#95580,#95581,#95582,#95583,#95584,#95585,#95586,#95587,#95588,#95589,#95590,
#95591,#95592,#95593,#95594,#95595,#95596,#95597,#95598,#95599,#95600,#95601),
 .UNSPECIFIED.,.F.,.F.,(4,3,3,3,3,3,3,3,3,3,3,3,3,3,3,3,3,3,3,3,3,3,3,3,
3,3,3,3,3,3,3,3,3,3,3,3,3,3,3,3,3,3,3,3,3,3,3,3,3,3,3,3,3,3,3,3,3,3,3,3,
3,3,3,3,3,3,3,3,3,3,3,3,3,3,3,3,3,3,3,3,3,3,3,3,3,3,3,3,3,3,3,3,3,3,3,3,
3,3,3,3,3,3,3,3,3,3,3,3,3,3,3,3,3,3,3,3,3,3,3,3,3,3,3,3,3,3,4),(0.,6.3863872932077E-5,
0.000127727745864154,0.000255455491728355,0.000510910983456715,0.00102182196691343,
0.00204364393382687,0.00395866138431376,0.00408728786765373,0.00729301756278118,
0.00817457573530746,0.0109725858555631,0.0137315028763566,0.0163491514706149,
0.0188948101717854,0.0214185435272282,0.0239103168830918,0.0245237272059223,
0.0268730591163259,0.0292008190500179,0.0314952438282925,0.0326983029412297,
0.0348110563874667,0.0369036365300053,0.0389623250662188,0.0408728786765371,
0.042768391397286,0.0446313687617704,0.0464752601039315,0.0482907238196907,
0.0490474544118446,0.0507095387659064,0.0523399285160803,0.0539528973554379,
0.055587463751295,0.057222030147152,0.0585122437009908,0.0597920455722731,
0.0610597218698551,0.0613093180148057,0.0631588971570508,0.0649809589485905,
0.0653966058824594,0.0672599831382585,0.0691003001841124,0.0694838937501131,
0.0704474234477631,0.0714030435344079,0.0723553074864157,0.0733045284193833,
0.0735711816177668,0.0751256651782625,0.0766739942267828,0.0776584694854205,
0.079205276027418,0.0807467960809093,0.0817457573530743,0.0833266384402915,
0.0837894012869011,0.0846318113552563,0.0854751143109977,0.0858330452207279,
0.087426131113557,0.0890419747830855,0.0899203330883816,0.0914954629283162,
0.0931453244021594,0.0947560270353013,0.0964254679294951,0.0980949088236888,
0.100273110033121,0.102182196691342,0.103761745158836,0.105357246450793,
0.106269484558996,0.108028728367388,0.109807518376732,0.111597064178548,
0.113402460236553,0.114444060294304,0.11648770422813,0.118525317988821,
0.12058098272364,0.122618636029611,0.124886611197948,0.12716589682006,0.129461943442204,
0.130793211764918,0.134072565285742,0.137393966194065,0.138967787500226,
0.141523871414855,0.144091743727972,0.146675795174257,0.147142363235533,
0.149988497106441,0.152848718747428,0.155730243243085,0.158623557998049,
0.16153491316658,0.163491514706148,0.16674704306941,0.170024638087439,0.173314174255391,
0.176623301543565,0.179840666176763,0.183487414628456,0.187155087402397,
0.190834713137538,0.19453197048957,0.196189817647378,0.200362893445446,
0.204549745330657,0.208750511135911,0.212965303417563,0.217201799274002,
0.221450368174175,0.225717874822285,0.228888120588607,0.233645051531473,
0.238413896994045,0.243200551547939,0.245237272059222,0.250355598656634,
0.255485848524186,0.260633046954424,0.261586423529837),.UNSPECIFIED.);
#2287=B_SPLINE_CURVE_WITH_KNOTS('',3,(#95602,#95603,#95604,#95605,#95606,
#95607,#95608,#95609,#95610,#95611,#95612,#95613,#95614,#95615,#95616,#95617,
#95618,#95619,#95620,#95621,#95622,#95623,#95624,#95625,#95626,#95627,#95628,
#95629,#95630,#95631,#95632,#95633,#95634,#95635,#95636,#95637,#95638,#95639,
#95640,#95641,#95642,#95643,#95644,#95645,#95646,#95647,#95648,#95649,#95650,
#95651,#95652,#95653,#95654,#95655,#95656,#95657,#95658,#95659,#95660,#95661,
#95662,#95663,#95664,#95665,#95666,#95667,#95668,#95669,#95670,#95671,#95672,
#95673,#95674,#95675,#95676,#95677,#95678,#95679,#95680,#95681,#95682,#95683,
#95684,#95685,#95686,#95687,#95688,#95689,#95690,#95691,#95692,#95693,#95694,
#95695,#95696,#95697,#95698,#95699,#95700,#95701,#95702,#95703,#95704,#95705,
#95706,#95707,#95708,#95709,#95710,#95711,#95712,#95713,#95714,#95715,#95716,
#95717,#95718,#95719,#95720,#95721,#95722,#95723,#95724,#95725,#95726,#95727,
#95728,#95729,#95730,#95731,#95732,#95733,#95734,#95735,#95736,#95737,#95738,
#95739,#95740,#95741,#95742,#95743,#95744,#95745,#95746,#95747,#95748,#95749,
#95750,#95751,#95752,#95753,#95754,#95755,#95756,#95757,#95758,#95759,#95760,
#95761,#95762,#95763,#95764,#95765,#95766,#95767,#95768,#95769,#95770,#95771,
#95772,#95773,#95774,#95775,#95776,#95777,#95778,#95779,#95780,#95781,#95782,
#95783,#95784,#95785,#95786,#95787,#95788,#95789,#95790,#95791,#95792,#95793,
#95794,#95795,#95796,#95797,#95798,#95799,#95800,#95801,#95802,#95803,#95804,
#95805,#95806,#95807,#95808,#95809,#95810,#95811,#95812,#95813,#95814,#95815,
#95816,#95817,#95818,#95819,#95820,#95821,#95822,#95823,#95824,#95825,#95826,
#95827,#95828,#95829,#95830,#95831,#95832,#95833,#95834,#95835,#95836,#95837,
#95838,#95839,#95840,#95841,#95842,#95843,#95844,#95845,#95846,#95847,#95848,
#95849,#95850,#95851,#95852,#95853,#95854,#95855,#95856,#95857,#95858,#95859,
#95860,#95861,#95862,#95863,#95864,#95865,#95866,#95867,#95868,#95869,#95870,
#95871,#95872,#95873,#95874,#95875,#95876,#95877,#95878,#95879,#95880,#95881,
#95882,#95883,#95884,#95885,#95886,#95887,#95888,#95889,#95890,#95891,#95892,
#95893,#95894,#95895,#95896),.UNSPECIFIED.,.F.,.F.,(4,3,3,3,3,3,3,3,3,3,
3,3,3,3,3,3,3,3,3,3,3,3,3,3,3,3,3,3,3,3,3,3,3,3,3,3,3,3,3,3,3,3,3,3,3,3,
3,3,3,3,3,3,3,3,3,3,3,3,3,3,3,3,3,3,3,3,3,3,3,3,3,3,3,3,3,3,3,3,3,3,3,3,
3,3,3,3,3,3,3,3,3,3,3,3,3,3,3,3,4),(0.1827680134667,0.1837097763468,0.183788376881043,
0.1848114574746,0.185834538068157,0.186450425254853,0.187665846450934,0.187847001796835,
0.189183047116277,0.189834967005636,0.190132837043007,0.191684431947844,
0.193343346752475,0.193763845867017,0.195709116538605,0.197497660619314,
0.197664069537048,0.199428846362787,0.201037120742463,0.201573334879782,
0.203004814586262,0.204361491262147,0.20486248419562,0.205540372303086,
0.206882660228423,0.208197711507143,0.208544895983774,0.209619358449715,
0.211014679742743,0.212227307771927,0.213385155422244,0.213865693507827,
0.214928865854929,0.215909719560081,0.217074197422792,0.218129218846608,
0.218238675285504,0.219212653160603,0.219592131348234,0.220477427707672,
0.221340257489479,0.222173866721717,0.222523667053981,0.223274543136388,
0.224537890016825,0.225767044721813,0.226557950821135,0.226956954924541,
0.227791691781628,0.228649200114669,0.228798160818618,0.229998539586015,
0.230362152850368,0.230639366712694,0.231774149191568,0.232961266775828,
0.234037876499932,0.234321778500848,0.235846026650995,0.236162984394925,
0.236957113549215,0.237648448805943,0.238004190289001,0.238546786721677,
0.23892479323604,0.239291967104069,0.239471814281867,0.239740665904253,
0.239845396183078,0.240033003014875,0.240209425489808,0.240305697656597,
0.240424316420931,0.240595157775524,0.240755298158673,0.240765999130116,
0.240868186286462,0.240934658995761,0.241007569397729,0.241076617911449,
0.241145342671251,0.241214156232952,0.241226300603636,0.241227953670809,
0.241269769601594,0.241310756863425,0.241351708284969,0.241393277997084,
0.241408856129991,0.24144045251339,0.241456451340395,0.241496529999511,
0.241528523246559,0.241561898975136,0.241571526708775,0.241603871867202,
0.241636532552263,0.241670569204549,0.241686602077155),.UNSPECIFIED.);
#2288=B_SPLINE_CURVE_WITH_KNOTS('',3,(#96180,#96181,#96182,#96183,#96184,
#96185,#96186,#96187,#96188,#96189,#96190,#96191,#96192,#96193,#96194,#96195,
#96196,#96197,#96198,#96199,#96200,#96201,#96202,#96203,#96204,#96205,#96206,
#96207,#96208,#96209,#96210,#96211,#96212,#96213,#96214,#96215,#96216,#96217,
#96218,#96219,#96220,#96221,#96222,#96223,#96224,#96225,#96226,#96227,#96228,
#96229,#96230,#96231,#96232,#96233,#96234,#96235,#96236,#96237),
 .UNSPECIFIED.,.F.,.F.,(4,2,2,2,2,2,2,2,2,2,2,2,2,2,2,2,2,2,2,2,2,2,2,2,
2,2,2,2,4),(0.152635115845842,0.155960973078063,0.159286830310285,0.165938544774729,
0.172590259239172,0.175916116471394,0.179241973703615,0.185893688168059,
0.18755661678417,0.189219545400281,0.192545402632502,0.199197117096946,
0.202522974329168,0.20584883156139,0.212500546025834,0.219152260490277,
0.225803974954721,0.232455689419165,0.239107403883608,0.245759118348052,
0.252410832812496,0.255736690044718,0.257399618660829,0.258231082968884,
0.258646815122912,0.258854681199926,0.258958614238433,0.259010580757686,
0.25906254727694),.UNSPECIFIED.);
#2289=B_SPLINE_CURVE_WITH_KNOTS('',3,(#96238,#96239,#96240,#96241,#96242,
#96243,#96244,#96245,#96246,#96247,#96248,#96249,#96250,#96251,#96252,#96253,
#96254,#96255,#96256,#96257,#96258,#96259,#96260,#96261,#96262,#96263),
 .UNSPECIFIED.,.F.,.F.,(4,2,2,2,2,2,2,2,2,2,2,2,4),(0.155674698583529,0.158344544285759,
0.161014389987988,0.166354081392447,0.171693772796906,0.174363618499135,
0.177033464201365,0.182373155605823,0.185043001308053,0.186377924159168,
0.187712847010282,0.193052538414741,0.1983922298192),.UNSPECIFIED.);
#2290=B_SPLINE_CURVE_WITH_KNOTS('',3,(#96265,#96266,#96267,#96268,#96269,
#96270,#96271,#96272,#96273,#96274,#96275,#96276,#96277,#96278,#96279,#96280,
#96281,#96282,#96283,#96284,#96285,#96286,#96287,#96288,#96289,#96290,#96291,
#96292,#96293,#96294,#96295,#96296,#96297,#96298,#96299,#96300,#96301,#96302,
#96303,#96304,#96305,#96306,#96307,#96308,#96309,#96310,#96311,#96312,#96313,
#96314,#96315,#96316,#96317,#96318,#96319,#96320,#96321,#96322,#96323,#96324,
#96325,#96326,#96327,#96328,#96329,#96330,#96331,#96332,#96333,#96334,#96335,
#96336,#96337,#96338,#96339,#96340,#96341,#96342,#96343,#96344,#96345,#96346,
#96347,#96348,#96349,#96350,#96351,#96352,#96353,#96354,#96355,#96356,#96357,
#96358,#96359,#96360,#96361,#96362,#96363,#96364,#96365,#96366,#96367,#96368,
#96369,#96370,#96371,#96372,#96373,#96374,#96375,#96376,#96377,#96378,#96379,
#96380,#96381,#96382,#96383,#96384,#96385,#96386,#96387,#96388,#96389,#96390,
#96391,#96392,#96393,#96394,#96395,#96396,#96397,#96398,#96399,#96400,#96401,
#96402,#96403,#96404,#96405,#96406,#96407,#96408,#96409,#96410,#96411,#96412,
#96413,#96414,#96415,#96416,#96417,#96418,#96419,#96420,#96421,#96422,#96423,
#96424,#96425,#96426,#96427,#96428,#96429,#96430,#96431,#96432,#96433,#96434,
#96435,#96436,#96437,#96438,#96439,#96440,#96441,#96442,#96443,#96444,#96445,
#96446,#96447,#96448,#96449,#96450,#96451,#96452,#96453,#96454,#96455,#96456,
#96457,#96458,#96459,#96460,#96461,#96462,#96463,#96464,#96465,#96466,#96467,
#96468,#96469,#96470,#96471,#96472,#96473,#96474,#96475,#96476,#96477,#96478,
#96479,#96480,#96481,#96482,#96483,#96484,#96485,#96486,#96487,#96488,#96489,
#96490,#96491,#96492,#96493,#96494,#96495,#96496,#96497,#96498,#96499,#96500,
#96501,#96502,#96503,#96504,#96505,#96506,#96507,#96508,#96509,#96510,#96511,
#96512,#96513,#96514,#96515,#96516,#96517,#96518,#96519,#96520,#96521,#96522,
#96523,#96524,#96525,#96526,#96527,#96528,#96529,#96530,#96531,#96532,#96533,
#96534,#96535,#96536,#96537,#96538,#96539,#96540,#96541,#96542,#96543,#96544),
 .UNSPECIFIED.,.F.,.F.,(4,3,3,3,3,3,3,3,3,3,3,3,3,3,3,3,3,3,3,3,3,3,3,3,
3,3,3,3,3,3,3,3,3,3,3,3,3,3,3,3,3,3,3,3,3,3,3,3,3,3,3,3,3,3,3,3,3,3,3,3,
3,3,3,3,3,3,3,3,3,3,3,3,3,3,3,3,3,3,3,3,3,3,3,3,3,3,3,3,3,3,3,3,3,4),(-5.99999997357394E-8,
4.38639073236214E-5,9.45970100728408E-5,0.000143126291908774,0.000186981185804612,
0.000191655573744707,0.000238520430505583,0.000270886863781888,0.000302536470316016,
0.000334074906589417,0.000343491009070944,0.000385878567015112,0.000429046783158217,
0.000477100861010902,0.00053209145428618,0.000565495260578844,0.000644015141512509,
0.000724439418075443,0.000806876778552401,0.00089462570938181,0.000937236773082297,
0.000954261722021523,0.00108689662222606,0.00122328225306106,0.00136816856359854,
0.00143142258303214,0.00159703908410309,0.00182842102722904,0.00190858344404277,
0.00248987825450814,0.00283814937392281,0.002862905166064,0.0032727783285689,
0.00369274471980585,0.00381722688808523,0.00453462896213004,0.0052489820951574,
0.00572587033212766,0.00670618958050466,0.00763451377617009,0.00765380603805355,
0.00886989494599809,0.0100859838539426,0.0112427315510617,0.0114518006642549,
0.012508327049095,0.0135431991630298,0.01455216354716,0.0150992258566461,
0.0152690875523398,0.0165866437037344,0.0177273665533294,0.0189215940108622,
0.0190863744404246,0.0201406885427821,0.0204648227868727,0.0213971958834355,
0.0223802573823971,0.0229036613285095,0.0233008123087915,0.0243620918098927,
0.0255722010062106,0.0261934427647077,0.0267209482165943,0.0279206208184966,
0.0290918341054633,0.0303053741212861,0.0305382351046792,0.0319468973072417,
0.0336437380028234,0.034355521992764,0.0357530268846585,0.0371798114132647,
0.0374722459149548,0.0381728088808489,0.0396630234973826,0.0412451663134016,
0.0428139984561576,0.0446963350828273,0.0458073826570186,0.0478860358725533,
0.0480757277027665,0.0499768000329801,0.0516885463137229,0.0533471197081705,
0.0534419564331883,0.0548581550144974,0.0560142987512958,0.0572592433212732,
0.058412277998669,0.058721495098687,0.0597401974867129,0.0607272993377569,
0.0610765302093581),.UNSPECIFIED.);
#2291=B_SPLINE_CURVE_WITH_KNOTS('',3,(#96666,#96667,#96668,#96669,#96670,
#96671,#96672,#96673,#96674,#96675,#96676,#96677,#96678,#96679,#96680,#96681,
#96682,#96683,#96684,#96685,#96686,#96687,#96688,#96689,#96690,#96691,#96692,
#96693,#96694,#96695,#96696,#96697,#96698,#96699,#96700,#96701,#96702,#96703,
#96704,#96705,#96706,#96707,#96708,#96709,#96710,#96711,#96712,#96713,#96714,
#96715,#96716,#96717,#96718,#96719,#96720,#96721,#96722,#96723,#96724,#96725,
#96726,#96727,#96728,#96729,#96730,#96731,#96732,#96733,#96734,#96735,#96736,
#96737,#96738,#96739,#96740,#96741,#96742,#96743,#96744,#96745,#96746,#96747),
 .UNSPECIFIED.,.F.,.F.,(4,3,3,3,3,3,3,3,3,3,3,3,3,3,3,3,3,3,3,3,3,3,3,3,
3,3,3,4),(0.,0.00184488703262337,0.00351661220106541,0.00518833736950746,
0.00531158003263634,0.00840640040076616,0.0103766747390149,0.0106295342414134,
0.0119592317531148,0.0129708434237686,0.0132884192546281,0.0148093646562269,
0.0155650121085223,0.0159474718369938,0.0207533494780297,0.0212654877795165,
0.0225952604584355,0.0233475181627834,0.0239242929808601,0.0254892764424578,
0.025941686847537,0.0265833716869893,0.0311300242170443,0.0319013210682786,
0.0363183615865516,0.0372192739307114,0.041056774429001,0.0415066989560588),
 .UNSPECIFIED.);
#2292=B_SPLINE_CURVE_WITH_KNOTS('',3,(#96787,#96788,#96789,#96790,#96791,
#96792,#96793,#96794,#96795,#96796,#96797,#96798),.UNSPECIFIED.,.F.,.F.,
(4,2,2,2,2,4),(0.0690311453325833,0.082781586176973,0.0965320270213627,
0.124032908710142,0.151533790398921,0.179034672087701),.UNSPECIFIED.);
#2293=B_SPLINE_CURVE_WITH_KNOTS('',3,(#96843,#96844,#96845,#96846,#96847,
#96848,#96849,#96850,#96851,#96852,#96853,#96854,#96855,#96856,#96857,#96858,
#96859,#96860,#96861,#96862,#96863,#96864,#96865,#96866,#96867,#96868,#96869,
#96870,#96871,#96872,#96873,#96874,#96875,#96876,#96877,#96878,#96879,#96880,
#96881,#96882,#96883,#96884,#96885,#96886,#96887,#96888,#96889,#96890,#96891,
#96892,#96893,#96894,#96895,#96896,#96897,#96898,#96899,#96900),
 .UNSPECIFIED.,.F.,.F.,(4,3,3,3,3,3,3,3,3,3,3,3,3,3,3,3,3,3,3,4),(6.16297582203915E-33,
0.0119699703913031,0.022367524718284,0.0239399407826063,0.0240424455537452,
0.0334984644888833,0.0423205469418825,0.0479759496178658,0.0480848911074903,
0.055447210326906,0.0600524042179919,0.0667007954868039,0.0721273366612355,
0.0721894789266184,0.0776788850245133,0.0829468346892967,0.0844114653878106,
0.0892194993938014,0.0938779179888398,0.0961697822083357),.UNSPECIFIED.);
#2910=ORIENTED_CLOSED_SHELL('',*,#45453,.F.);
#2911=ORIENTED_CLOSED_SHELL('',*,#45454,.F.);
#2919=BREP_WITH_VOIDS('Body1',#45455,(#2910,#2911));
#2923=SHAPE_REPRESENTATION_RELATIONSHIP('SRR','None',#130945,#2931);
#2931=ADVANCED_BREP_SHAPE_REPRESENTATION('',(#2919),#130905);
#2939=STYLED_ITEM('',(#130991),#2919);
#3575=PLANE('',#48166);
#3576=PLANE('',#48170);
#3577=PLANE('',#48171);
#3578=PLANE('',#48172);
#3579=PLANE('',#48173);
#3580=PLANE('',#48176);
#3581=PLANE('',#48179);
#3582=PLANE('',#48182);
#3583=PLANE('',#48275);
#3584=PLANE('',#48284);
#3585=PLANE('',#48285);
#3586=PLANE('',#48286);
#3587=PLANE('',#48365);
#3588=PLANE('',#48366);
#3589=PLANE('',#48369);
#3590=PLANE('',#48370);
#3591=PLANE('',#48371);
#3592=PLANE('',#48400);
#3593=PLANE('',#48401);
#3594=PLANE('',#48403);
#3595=PLANE('',#48404);
#3596=PLANE('',#48405);
#3597=PLANE('',#48434);
#3598=PLANE('',#48435);
#3599=PLANE('',#48437);
#3600=PLANE('',#48438);
#3601=PLANE('',#48439);
#3602=PLANE('',#48468);
#3603=PLANE('',#48469);
#3604=PLANE('',#48471);
#3605=PLANE('',#48472);
#3606=PLANE('',#48473);
#3607=PLANE('',#48474);
#3608=PLANE('',#48475);
#3609=PLANE('',#48476);
#3610=PLANE('',#48544);
#3611=PLANE('',#48557);
#3612=PLANE('',#48563);
#3613=PLANE('',#48564);
#3614=PLANE('',#48565);
#3615=PLANE('',#48567);
#3616=PLANE('',#48568);
#3617=PLANE('',#48573);
#5022=LINE('',#85910,#6796);
#5023=LINE('',#85914,#6797);
#5024=LINE('',#85919,#6798);
#5025=LINE('',#85920,#6799);
#5026=LINE('',#85921,#6800);
#5027=LINE('',#85925,#6801);
#5028=LINE('',#85929,#6802);
#5029=LINE('',#85930,#6803);
#5030=LINE('',#85938,#6804);
#5031=LINE('',#85941,#6805);
#5032=LINE('',#85944,#6806);
#5033=LINE('',#85946,#6807);
#5034=LINE('',#85947,#6808);
#5035=LINE('',#85951,#6809);
#5036=LINE('',#85954,#6810);
#5037=LINE('',#85955,#6811);
#5038=LINE('',#86018,#6812);
#5039=LINE('',#86081,#6813);
#5040=LINE('',#86085,#6814);
#5041=LINE('',#86145,#6815);
#5042=LINE('',#86187,#6816);
#5043=LINE('',#86387,#6817);
#5044=LINE('',#86412,#6818);
#5045=LINE('',#86418,#6819);
#5046=LINE('',#86443,#6820);
#5047=LINE('',#86449,#6821);
#5048=LINE('',#86474,#6822);
#5049=LINE('',#86480,#6823);
#5050=LINE('',#86484,#6824);
#5051=LINE('',#86597,#6825);
#5052=LINE('',#86605,#6826);
#5053=LINE('',#86608,#6827);
#5054=LINE('',#86723,#6828);
#5055=LINE('',#86727,#6829);
#5056=LINE('',#86840,#6830);
#5057=LINE('',#86848,#6831);
#5058=LINE('',#86851,#6832);
#5059=LINE('',#86966,#6833);
#5060=LINE('',#86970,#6834);
#5061=LINE('',#87083,#6835);
#5062=LINE('',#87091,#6836);
#5063=LINE('',#87094,#6837);
#5064=LINE('',#87208,#6838);
#5065=LINE('',#87212,#6839);
#5066=LINE('',#87331,#6840);
#5067=LINE('',#87605,#6841);
#5068=LINE('',#87607,#6842);
#5069=LINE('',#87608,#6843);
#5070=LINE('',#87612,#6844);
#5071=LINE('',#87616,#6845);
#5072=LINE('',#87628,#6846);
#5073=LINE('',#88057,#6847);
#5074=LINE('',#88061,#6848);
#5075=LINE('',#88499,#6849);
#5076=LINE('',#88501,#6850);
#5077=LINE('',#88503,#6851);
#5078=LINE('',#88504,#6852);
#5079=LINE('',#88507,#6853);
#5080=LINE('',#88509,#6854);
#5081=LINE('',#88510,#6855);
#5082=LINE('',#88514,#6856);
#5083=LINE('',#88515,#6857);
#5084=LINE('',#88516,#6858);
#5085=LINE('',#89284,#6859);
#5086=LINE('',#89287,#6860);
#5087=LINE('',#89319,#6861);
#5088=LINE('',#89711,#6862);
#5089=LINE('',#89712,#6863);
#5090=LINE('',#89717,#6864);
#5091=LINE('',#89718,#6865);
#5092=LINE('',#89726,#6866);
#5093=LINE('',#89906,#6867);
#5094=LINE('',#89907,#6868);
#5095=LINE('',#89916,#6869);
#5096=LINE('',#89917,#6870);
#5097=LINE('',#90113,#6871);
#5098=LINE('',#90114,#6872);
#5099=LINE('',#90116,#6873);
#5100=LINE('',#90118,#6874);
#5101=LINE('',#90119,#6875);
#5102=LINE('',#90123,#6876);
#5103=LINE('',#90124,#6877);
#5104=LINE('',#90126,#6878);
#5105=LINE('',#90127,#6879);
#5106=LINE('',#90135,#6880);
#5107=LINE('',#90136,#6881);
#5108=LINE('',#90144,#6882);
#5109=LINE('',#90145,#6883);
#5110=LINE('',#90302,#6884);
#5111=LINE('',#90307,#6885);
#5112=LINE('',#90308,#6886);
#5113=LINE('',#90313,#6887);
#5114=LINE('',#90314,#6888);
#5115=LINE('',#90318,#6889);
#5116=LINE('',#90482,#6890);
#5117=LINE('',#90483,#6891);
#5118=LINE('',#90485,#6892);
#5119=LINE('',#90486,#6893);
#5120=LINE('',#90490,#6894);
#5121=LINE('',#90491,#6895);
#5122=LINE('',#90499,#6896);
#5123=LINE('',#90500,#6897);
#5124=LINE('',#90508,#6898);
#5125=LINE('',#90509,#6899);
#5126=LINE('',#90666,#6900);
#5127=LINE('',#90671,#6901);
#5128=LINE('',#90672,#6902);
#5129=LINE('',#90677,#6903);
#5130=LINE('',#90678,#6904);
#5131=LINE('',#90682,#6905);
#5132=LINE('',#90846,#6906);
#5133=LINE('',#90847,#6907);
#5134=LINE('',#90849,#6908);
#5135=LINE('',#90850,#6909);
#5136=LINE('',#90854,#6910);
#5137=LINE('',#90855,#6911);
#5138=LINE('',#90863,#6912);
#5139=LINE('',#90864,#6913);
#5140=LINE('',#90872,#6914);
#5141=LINE('',#90873,#6915);
#5142=LINE('',#91030,#6916);
#5143=LINE('',#91035,#6917);
#5144=LINE('',#91036,#6918);
#5145=LINE('',#91041,#6919);
#5146=LINE('',#91042,#6920);
#5147=LINE('',#91046,#6921);
#5148=LINE('',#91210,#6922);
#5149=LINE('',#91211,#6923);
#5150=LINE('',#91213,#6924);
#5151=LINE('',#91214,#6925);
#5152=LINE('',#91218,#6926);
#5153=LINE('',#91219,#6927);
#5154=LINE('',#91224,#6928);
#5155=LINE('',#91226,#6929);
#5156=LINE('',#91228,#6930);
#5157=LINE('',#91234,#6931);
#5158=LINE('',#91398,#6932);
#5159=LINE('',#91473,#6933);
#5160=LINE('',#91961,#6934);
#5161=LINE('',#91963,#6935);
#5162=LINE('',#92536,#6936);
#5163=LINE('',#92875,#6937);
#5164=LINE('',#92881,#6938);
#5165=LINE('',#92882,#6939);
#5166=LINE('',#93005,#6940);
#5167=LINE('',#93094,#6941);
#5168=LINE('',#94832,#6942);
#5169=LINE('',#94833,#6943);
#5170=LINE('',#94865,#6944);
#5171=LINE('',#94866,#6945);
#5172=LINE('',#94869,#6946);
#5173=LINE('',#94871,#6947);
#5174=LINE('',#96547,#6948);
#5175=LINE('',#96548,#6949);
#5176=LINE('',#96557,#6950);
#5177=LINE('',#96568,#6951);
#5178=LINE('',#96570,#6952);
#5179=LINE('',#96587,#6953);
#5180=LINE('',#96749,#6954);
#5181=LINE('',#96750,#6955);
#5182=LINE('',#96918,#6956);
#5183=LINE('',#96920,#6957);
#5184=LINE('',#96922,#6958);
#5185=LINE('',#96924,#6959);
#6796=VECTOR('',#57541,1000.);
#6797=VECTOR('',#57544,1000.);
#6798=VECTOR('',#57549,1000.);
#6799=VECTOR('',#57550,1000.);
#6800=VECTOR('',#57551,1000.);
#6801=VECTOR('',#57554,1000.);
#6802=VECTOR('',#57561,1000.);
#6803=VECTOR('',#57562,1000.);
#6804=VECTOR('',#57571,1000.);
#6805=VECTOR('',#57574,1000.);
#6806=VECTOR('',#57577,1000.);
#6807=VECTOR('',#57578,1000.);
#6808=VECTOR('',#57579,1000.);
#6809=VECTOR('',#57584,1000.);
#6810=VECTOR('',#57587,1000.);
#6811=VECTOR('',#57588,1000.);
#6812=VECTOR('',#57597,1000.);
#6813=VECTOR('',#57600,1000.);
#6814=VECTOR('',#57603,1000.);
#6815=VECTOR('',#57606,1000.);
#6816=VECTOR('',#57609,28.5226030790361);
#6817=VECTOR('',#57624,1000.);
#6818=VECTOR('',#57627,1000.);
#6819=VECTOR('',#57632,1000.);
#6820=VECTOR('',#57635,1000.);
#6821=VECTOR('',#57640,1000.);
#6822=VECTOR('',#57643,1000.);
#6823=VECTOR('',#57648,16.);
#6824=VECTOR('',#57651,1000.);
#6825=VECTOR('',#57654,1000.);
#6826=VECTOR('',#57663,1000.);
#6827=VECTOR('',#57666,1000.);
#6828=VECTOR('',#57697,16.);
#6829=VECTOR('',#57700,1000.);
#6830=VECTOR('',#57703,1000.);
#6831=VECTOR('',#57712,1000.);
#6832=VECTOR('',#57715,1000.);
#6833=VECTOR('',#57746,16.);
#6834=VECTOR('',#57749,1000.);
#6835=VECTOR('',#57752,1000.);
#6836=VECTOR('',#57761,1000.);
#6837=VECTOR('',#57764,1000.);
#6838=VECTOR('',#57795,26.0226030790361);
#6839=VECTOR('',#57798,1000.);
#6840=VECTOR('',#57801,1000.);
#6841=VECTOR('',#57814,1000.);
#6842=VECTOR('',#57815,1000.);
#6843=VECTOR('',#57816,1000.);
#6844=VECTOR('',#57819,1000.);
#6845=VECTOR('',#57822,1000.);
#6846=VECTOR('',#57825,1000.);
#6847=VECTOR('',#57828,1000.);
#6848=VECTOR('',#57831,1000.);
#6849=VECTOR('',#57836,1000.);
#6850=VECTOR('',#57837,1000.);
#6851=VECTOR('',#57838,1000.);
#6852=VECTOR('',#57839,1000.);
#6853=VECTOR('',#57842,1000.);
#6854=VECTOR('',#57843,1000.);
#6855=VECTOR('',#57844,1000.);
#6856=VECTOR('',#57847,1000.);
#6857=VECTOR('',#57848,1000.);
#6858=VECTOR('',#57849,1000.);
#6859=VECTOR('',#57872,1000.);
#6860=VECTOR('',#57875,1000.);
#6861=VECTOR('',#57884,1000.);
#6862=VECTOR('',#57947,1000.);
#6863=VECTOR('',#57948,1000.);
#6864=VECTOR('',#57953,1000.);
#6865=VECTOR('',#57954,1000.);
#6866=VECTOR('',#57965,1000.);
#6867=VECTOR('',#57976,1000.);
#6868=VECTOR('',#57977,1000.);
#6869=VECTOR('',#57988,1000.);
#6870=VECTOR('',#57989,1000.);
#6871=VECTOR('',#58014,1000.);
#6872=VECTOR('',#58015,1000.);
#6873=VECTOR('',#58018,1000.);
#6874=VECTOR('',#58021,1000.);
#6875=VECTOR('',#58022,1000.);
#6876=VECTOR('',#58029,1000.);
#6877=VECTOR('',#58030,1000.);
#6878=VECTOR('',#58033,1000.);
#6879=VECTOR('',#58034,1000.);
#6880=VECTOR('',#58045,1000.);
#6881=VECTOR('',#58046,1000.);
#6882=VECTOR('',#58057,1000.);
#6883=VECTOR('',#58058,1000.);
#6884=VECTOR('',#58075,1000.);
#6885=VECTOR('',#58080,1000.);
#6886=VECTOR('',#58081,1000.);
#6887=VECTOR('',#58086,1000.);
#6888=VECTOR('',#58087,1000.);
#6889=VECTOR('',#58092,1000.);
#6890=VECTOR('',#58105,1000.);
#6891=VECTOR('',#58106,1000.);
#6892=VECTOR('',#58109,1000.);
#6893=VECTOR('',#58110,1000.);
#6894=VECTOR('',#58117,1000.);
#6895=VECTOR('',#58118,1000.);
#6896=VECTOR('',#58129,1000.);
#6897=VECTOR('',#58130,1000.);
#6898=VECTOR('',#58141,1000.);
#6899=VECTOR('',#58142,1000.);
#6900=VECTOR('',#58159,1000.);
#6901=VECTOR('',#58164,1000.);
#6902=VECTOR('',#58165,1000.);
#6903=VECTOR('',#58170,1000.);
#6904=VECTOR('',#58171,1000.);
#6905=VECTOR('',#58176,1000.);
#6906=VECTOR('',#58189,1000.);
#6907=VECTOR('',#58190,1000.);
#6908=VECTOR('',#58193,1000.);
#6909=VECTOR('',#58194,1000.);
#6910=VECTOR('',#58201,1000.);
#6911=VECTOR('',#58202,1000.);
#6912=VECTOR('',#58213,1000.);
#6913=VECTOR('',#58214,1000.);
#6914=VECTOR('',#58225,1000.);
#6915=VECTOR('',#58226,1000.);
#6916=VECTOR('',#58243,1000.);
#6917=VECTOR('',#58248,1000.);
#6918=VECTOR('',#58249,1000.);
#6919=VECTOR('',#58254,1000.);
#6920=VECTOR('',#58255,1000.);
#6921=VECTOR('',#58260,1000.);
#6922=VECTOR('',#58273,1000.);
#6923=VECTOR('',#58274,1000.);
#6924=VECTOR('',#58277,1000.);
#6925=VECTOR('',#58278,1000.);
#6926=VECTOR('',#58285,1000.);
#6927=VECTOR('',#58286,1000.);
#6928=VECTOR('',#58295,1000.);
#6929=VECTOR('',#58298,1000.);
#6930=VECTOR('',#58301,1000.);
#6931=VECTOR('',#58308,1000.);
#6932=VECTOR('',#58325,1000.);
#6933=VECTOR('',#58338,1000.);
#6934=VECTOR('',#58351,1000.);
#6935=VECTOR('',#58352,1000.);
#6936=VECTOR('',#58377,1000.);
#6937=VECTOR('',#58394,1000.);
#6938=VECTOR('',#58403,1000.);
#6939=VECTOR('',#58404,1000.);
#6940=VECTOR('',#58423,1000.);
#6941=VECTOR('',#58436,1000.);
#6942=VECTOR('',#58475,1000.);
#6943=VECTOR('',#58476,1000.);
#6944=VECTOR('',#58477,1000.);
#6945=VECTOR('',#58478,1000.);
#6946=VECTOR('',#58481,1000.);
#6947=VECTOR('',#58482,1000.);
#6948=VECTOR('',#58491,1000.);
#6949=VECTOR('',#58492,1000.);
#6950=VECTOR('',#58493,1000.);
#6951=VECTOR('',#58498,1000.);
#6952=VECTOR('',#58501,1000.);
#6953=VECTOR('',#58502,1000.);
#6954=VECTOR('',#58505,1000.);
#6955=VECTOR('',#58506,1000.);
#6956=VECTOR('',#58513,1000.);
#6957=VECTOR('',#58516,1000.);
#6958=VECTOR('',#58519,1000.);
#6959=VECTOR('',#58522,1000.);
#8541=CYLINDRICAL_SURFACE('',#48163,0.500000000000028);
#8542=CYLINDRICAL_SURFACE('',#48167,0.499999999999973);
#8543=CYLINDRICAL_SURFACE('',#48177,0.499999999999973);
#8544=CYLINDRICAL_SURFACE('',#48180,0.500000000000028);
#8545=CYLINDRICAL_SURFACE('',#48183,28.5226030790361);
#8546=CYLINDRICAL_SURFACE('',#48193,16.5);
#8547=CYLINDRICAL_SURFACE('',#48196,16.5);
#8548=CYLINDRICAL_SURFACE('',#48199,16.5);
#8549=CYLINDRICAL_SURFACE('',#48202,16.);
#8550=CYLINDRICAL_SURFACE('',#48208,3.96802221877415);
#8551=CYLINDRICAL_SURFACE('',#48224,16.);
#8552=CYLINDRICAL_SURFACE('',#48230,3.96802221877416);
#8553=CYLINDRICAL_SURFACE('',#48246,16.);
#8554=CYLINDRICAL_SURFACE('',#48252,3.96802221877416);
#8555=CYLINDRICAL_SURFACE('',#48268,26.0226030790361);
#8556=CYLINDRICAL_SURFACE('',#48278,30.);
#8557=CYLINDRICAL_SURFACE('',#48281,30.);
#8558=CYLINDRICAL_SURFACE('',#48296,0.5);
#8559=CYLINDRICAL_SURFACE('',#48298,0.5);
#8560=CYLINDRICAL_SURFACE('',#48300,0.5);
#8561=CYLINDRICAL_SURFACE('',#48307,0.5);
#8562=CYLINDRICAL_SURFACE('',#48309,0.5);
#8563=CYLINDRICAL_SURFACE('',#48311,0.5);
#8564=CYLINDRICAL_SURFACE('',#48318,0.5);
#8565=CYLINDRICAL_SURFACE('',#48320,0.5);
#8566=CYLINDRICAL_SURFACE('',#48332,0.700000000000006);
#8567=CYLINDRICAL_SURFACE('',#48334,0.700000000000006);
#8568=CYLINDRICAL_SURFACE('',#48339,0.700000000000006);
#8569=CYLINDRICAL_SURFACE('',#48344,0.700000000000006);
#8570=CYLINDRICAL_SURFACE('',#48349,0.700000000000006);
#8571=CYLINDRICAL_SURFACE('',#48362,0.700000000000006);
#8572=CYLINDRICAL_SURFACE('',#48363,0.700000000000006);
#8573=CYLINDRICAL_SURFACE('',#48364,0.700000000000006);
#8574=CYLINDRICAL_SURFACE('',#48367,4.75563473233925);
#8575=CYLINDRICAL_SURFACE('',#48368,4.75563473233925);
#8576=CYLINDRICAL_SURFACE('',#48372,0.499999999999998);
#8577=CYLINDRICAL_SURFACE('',#48378,0.499999999999998);
#8578=CYLINDRICAL_SURFACE('',#48385,0.5);
#8579=CYLINDRICAL_SURFACE('',#48387,0.499999999999998);
#8580=CYLINDRICAL_SURFACE('',#48389,0.499999999999998);
#8581=CYLINDRICAL_SURFACE('',#48391,0.5);
#8582=CYLINDRICAL_SURFACE('',#48398,0.499999999999998);
#8583=CYLINDRICAL_SURFACE('',#48399,0.499999999999998);
#8584=CYLINDRICAL_SURFACE('',#48402,3.96802221877416);
#8585=CYLINDRICAL_SURFACE('',#48406,0.499999999999998);
#8586=CYLINDRICAL_SURFACE('',#48412,0.499999999999998);
#8587=CYLINDRICAL_SURFACE('',#48419,0.5);
#8588=CYLINDRICAL_SURFACE('',#48421,0.499999999999998);
#8589=CYLINDRICAL_SURFACE('',#48423,0.499999999999998);
#8590=CYLINDRICAL_SURFACE('',#48425,0.5);
#8591=CYLINDRICAL_SURFACE('',#48432,0.5);
#8592=CYLINDRICAL_SURFACE('',#48433,0.499999999999998);
#8593=CYLINDRICAL_SURFACE('',#48436,3.96802221877416);
#8594=CYLINDRICAL_SURFACE('',#48440,0.500000000000003);
#8595=CYLINDRICAL_SURFACE('',#48446,0.500000000000003);
#8596=CYLINDRICAL_SURFACE('',#48453,0.5);
#8597=CYLINDRICAL_SURFACE('',#48455,0.500000000000003);
#8598=CYLINDRICAL_SURFACE('',#48457,0.500000000000003);
#8599=CYLINDRICAL_SURFACE('',#48459,0.5);
#8600=CYLINDRICAL_SURFACE('',#48466,0.500000000000003);
#8601=CYLINDRICAL_SURFACE('',#48467,0.500000000000003);
#8602=CYLINDRICAL_SURFACE('',#48470,3.96802221877415);
#8603=CYLINDRICAL_SURFACE('',#48477,0.5);
#8604=CYLINDRICAL_SURFACE('',#48486,0.5);
#8605=CYLINDRICAL_SURFACE('',#48492,0.5);
#8606=CYLINDRICAL_SURFACE('',#48499,1.);
#8607=CYLINDRICAL_SURFACE('',#48510,1.);
#8608=CYLINDRICAL_SURFACE('',#48518,1.);
#8609=CYLINDRICAL_SURFACE('',#48523,1.);
#8610=CYLINDRICAL_SURFACE('',#48531,1.);
#8611=CYLINDRICAL_SURFACE('',#48537,1.);
#8612=CYLINDRICAL_SURFACE('',#48558,30.);
#8613=CYLINDRICAL_SURFACE('',#48562,30.);
#8614=CYLINDRICAL_SURFACE('',#48566,1.);
#8615=CYLINDRICAL_SURFACE('',#48569,1.);
#8616=CYLINDRICAL_SURFACE('',#48570,1.);
#8617=CYLINDRICAL_SURFACE('',#48571,1.);
#8618=CYLINDRICAL_SURFACE('',#48572,1.);
#10896=FACE_OUTER_BOUND('',#14931,.T.);
#10897=FACE_OUTER_BOUND('',#14932,.T.);
#10898=FACE_OUTER_BOUND('',#14933,.T.);
#10899=FACE_OUTER_BOUND('',#14934,.T.);
#10900=FACE_OUTER_BOUND('',#14935,.T.);
#10901=FACE_OUTER_BOUND('',#14936,.T.);
#10902=FACE_OUTER_BOUND('',#14937,.T.);
#10903=FACE_OUTER_BOUND('',#14938,.T.);
#10904=FACE_OUTER_BOUND('',#14939,.T.);
#10905=FACE_OUTER_BOUND('',#14940,.T.);
#10906=FACE_OUTER_BOUND('',#14941,.T.);
#10907=FACE_OUTER_BOUND('',#14942,.T.);
#10908=FACE_OUTER_BOUND('',#14943,.T.);
#10909=FACE_OUTER_BOUND('',#14944,.T.);
#10910=FACE_OUTER_BOUND('',#14945,.T.);
#10911=FACE_OUTER_BOUND('',#14946,.T.);
#10912=FACE_OUTER_BOUND('',#14947,.T.);
#10913=FACE_OUTER_BOUND('',#14948,.T.);
#10914=FACE_OUTER_BOUND('',#14949,.T.);
#10915=FACE_OUTER_BOUND('',#14950,.T.);
#10916=FACE_OUTER_BOUND('',#14951,.T.);
#10917=FACE_OUTER_BOUND('',#14952,.T.);
#10918=FACE_OUTER_BOUND('',#14953,.T.);
#10919=FACE_OUTER_BOUND('',#14954,.T.);
#10920=FACE_OUTER_BOUND('',#14955,.T.);
#10921=FACE_OUTER_BOUND('',#14956,.T.);
#10922=FACE_OUTER_BOUND('',#14957,.T.);
#10923=FACE_OUTER_BOUND('',#14958,.T.);
#10924=FACE_OUTER_BOUND('',#14959,.T.);
#10925=FACE_OUTER_BOUND('',#14960,.T.);
#10926=FACE_OUTER_BOUND('',#14961,.T.);
#10927=FACE_OUTER_BOUND('',#14962,.T.);
#10928=FACE_OUTER_BOUND('',#14963,.T.);
#10929=FACE_OUTER_BOUND('',#14964,.T.);
#10930=FACE_OUTER_BOUND('',#14965,.T.);
#10931=FACE_OUTER_BOUND('',#14966,.T.);
#10932=FACE_OUTER_BOUND('',#14967,.T.);
#10933=FACE_OUTER_BOUND('',#14968,.T.);
#10934=FACE_OUTER_BOUND('',#14969,.T.);
#10935=FACE_OUTER_BOUND('',#14970,.T.);
#10936=FACE_OUTER_BOUND('',#14971,.T.);
#10937=FACE_OUTER_BOUND('',#14972,.T.);
#10938=FACE_OUTER_BOUND('',#14973,.T.);
#10939=FACE_OUTER_BOUND('',#14974,.T.);
#10940=FACE_OUTER_BOUND('',#14975,.T.);
#10941=FACE_OUTER_BOUND('',#14976,.T.);
#10942=FACE_OUTER_BOUND('',#14977,.T.);
#10943=FACE_OUTER_BOUND('',#14978,.T.);
#10944=FACE_OUTER_BOUND('',#14979,.T.);
#10945=FACE_OUTER_BOUND('',#14980,.T.);
#10946=FACE_OUTER_BOUND('',#14981,.T.);
#10947=FACE_OUTER_BOUND('',#14982,.T.);
#10948=FACE_OUTER_BOUND('',#14983,.T.);
#10949=FACE_OUTER_BOUND('',#14984,.T.);
#10950=FACE_OUTER_BOUND('',#14985,.T.);
#10951=FACE_OUTER_BOUND('',#14986,.T.);
#10952=FACE_OUTER_BOUND('',#14987,.T.);
#10953=FACE_OUTER_BOUND('',#14988,.T.);
#10954=FACE_OUTER_BOUND('',#14989,.T.);
#10955=FACE_OUTER_BOUND('',#14990,.T.);
#10956=FACE_OUTER_BOUND('',#14991,.T.);
#10957=FACE_OUTER_BOUND('',#14992,.T.);
#10958=FACE_OUTER_BOUND('',#14993,.T.);
#10959=FACE_OUTER_BOUND('',#14994,.T.);
#10960=FACE_OUTER_BOUND('',#14995,.T.);
#10961=FACE_OUTER_BOUND('',#14996,.T.);
#10962=FACE_OUTER_BOUND('',#14997,.T.);
#10963=FACE_OUTER_BOUND('',#14998,.T.);
#10964=FACE_OUTER_BOUND('',#14999,.T.);
#10965=FACE_OUTER_BOUND('',#15000,.T.);
#10966=FACE_OUTER_BOUND('',#15001,.T.);
#10967=FACE_OUTER_BOUND('',#15002,.T.);
#10968=FACE_OUTER_BOUND('',#15003,.T.);
#10969=FACE_OUTER_BOUND('',#15004,.T.);
#10970=FACE_OUTER_BOUND('',#15005,.T.);
#10971=FACE_OUTER_BOUND('',#15006,.T.);
#10972=FACE_OUTER_BOUND('',#15007,.T.);
#10973=FACE_OUTER_BOUND('',#15008,.T.);
#10974=FACE_OUTER_BOUND('',#15009,.T.);
#10975=FACE_OUTER_BOUND('',#15010,.T.);
#10976=FACE_OUTER_BOUND('',#15011,.T.);
#10977=FACE_OUTER_BOUND('',#15012,.T.);
#10978=FACE_OUTER_BOUND('',#15013,.T.);
#10979=FACE_OUTER_BOUND('',#15014,.T.);
#10980=FACE_OUTER_BOUND('',#15015,.T.);
#10981=FACE_OUTER_BOUND('',#15016,.T.);
#10982=FACE_OUTER_BOUND('',#15017,.T.);
#10983=FACE_OUTER_BOUND('',#15018,.T.);
#10984=FACE_OUTER_BOUND('',#15019,.T.);
#10985=FACE_OUTER_BOUND('',#15020,.T.);
#10986=FACE_OUTER_BOUND('',#15021,.T.);
#10987=FACE_OUTER_BOUND('',#15022,.T.);
#10988=FACE_OUTER_BOUND('',#15023,.T.);
#10989=FACE_OUTER_BOUND('',#15024,.T.);
#10990=FACE_OUTER_BOUND('',#15025,.T.);
#10991=FACE_OUTER_BOUND('',#15026,.T.);
#10992=FACE_OUTER_BOUND('',#15027,.T.);
#10993=FACE_OUTER_BOUND('',#15028,.T.);
#10994=FACE_OUTER_BOUND('',#15029,.T.);
#10995=FACE_OUTER_BOUND('',#15030,.T.);
#10996=FACE_OUTER_BOUND('',#15031,.T.);
#10997=FACE_OUTER_BOUND('',#15032,.T.);
#10998=FACE_OUTER_BOUND('',#15033,.T.);
#10999=FACE_OUTER_BOUND('',#15034,.T.);
#11000=FACE_OUTER_BOUND('',#15035,.T.);
#11001=FACE_OUTER_BOUND('',#15036,.T.);
#11002=FACE_OUTER_BOUND('',#15037,.T.);
#11003=FACE_OUTER_BOUND('',#15038,.T.);
#11004=FACE_OUTER_BOUND('',#15039,.T.);
#11005=FACE_OUTER_BOUND('',#15040,.T.);
#11006=FACE_OUTER_BOUND('',#15041,.T.);
#11007=FACE_OUTER_BOUND('',#15042,.T.);
#11008=FACE_OUTER_BOUND('',#15043,.T.);
#11009=FACE_OUTER_BOUND('',#15044,.T.);
#11010=FACE_OUTER_BOUND('',#15045,.T.);
#11011=FACE_OUTER_BOUND('',#15046,.T.);
#11012=FACE_OUTER_BOUND('',#15047,.T.);
#11013=FACE_OUTER_BOUND('',#15048,.T.);
#11014=FACE_OUTER_BOUND('',#15049,.T.);
#11015=FACE_OUTER_BOUND('',#15050,.T.);
#11016=FACE_OUTER_BOUND('',#15051,.T.);
#11017=FACE_OUTER_BOUND('',#15052,.T.);
#11018=FACE_OUTER_BOUND('',#15053,.T.);
#11019=FACE_OUTER_BOUND('',#15054,.T.);
#11020=FACE_OUTER_BOUND('',#15055,.T.);
#11021=FACE_OUTER_BOUND('',#15056,.T.);
#11022=FACE_OUTER_BOUND('',#15057,.T.);
#11023=FACE_OUTER_BOUND('',#15058,.T.);
#11024=FACE_OUTER_BOUND('',#15059,.T.);
#11025=FACE_OUTER_BOUND('',#15060,.T.);
#11026=FACE_OUTER_BOUND('',#15061,.T.);
#11027=FACE_OUTER_BOUND('',#15062,.T.);
#11028=FACE_OUTER_BOUND('',#15063,.T.);
#11029=FACE_OUTER_BOUND('',#15064,.T.);
#11030=FACE_OUTER_BOUND('',#15065,.T.);
#11031=FACE_OUTER_BOUND('',#15066,.T.);
#11032=FACE_OUTER_BOUND('',#15067,.T.);
#11033=FACE_OUTER_BOUND('',#15068,.T.);
#11034=FACE_OUTER_BOUND('',#15069,.T.);
#11035=FACE_OUTER_BOUND('',#15070,.T.);
#11036=FACE_OUTER_BOUND('',#15071,.T.);
#11037=FACE_OUTER_BOUND('',#15072,.T.);
#11038=FACE_OUTER_BOUND('',#15073,.T.);
#11039=FACE_OUTER_BOUND('',#15074,.T.);
#11040=FACE_OUTER_BOUND('',#15075,.T.);
#11041=FACE_OUTER_BOUND('',#15076,.T.);
#11042=FACE_OUTER_BOUND('',#15077,.T.);
#11043=FACE_OUTER_BOUND('',#15078,.T.);
#11044=FACE_OUTER_BOUND('',#15079,.T.);
#11045=FACE_OUTER_BOUND('',#15080,.T.);
#11046=FACE_OUTER_BOUND('',#15081,.T.);
#11047=FACE_OUTER_BOUND('',#15082,.T.);
#11048=FACE_OUTER_BOUND('',#15083,.T.);
#11049=FACE_OUTER_BOUND('',#15084,.T.);
#11050=FACE_OUTER_BOUND('',#15085,.T.);
#11051=FACE_OUTER_BOUND('',#15086,.T.);
#11052=FACE_OUTER_BOUND('',#15087,.T.);
#11053=FACE_OUTER_BOUND('',#15088,.T.);
#11054=FACE_OUTER_BOUND('',#15089,.T.);
#11055=FACE_OUTER_BOUND('',#15090,.T.);
#11056=FACE_OUTER_BOUND('',#15091,.T.);
#11057=FACE_OUTER_BOUND('',#15092,.T.);
#11058=FACE_OUTER_BOUND('',#15093,.T.);
#11059=FACE_OUTER_BOUND('',#15094,.T.);
#11060=FACE_OUTER_BOUND('',#15095,.T.);
#11061=FACE_OUTER_BOUND('',#15096,.T.);
#11062=FACE_OUTER_BOUND('',#15097,.T.);
#11063=FACE_OUTER_BOUND('',#15098,.T.);
#11064=FACE_OUTER_BOUND('',#15099,.T.);
#11065=FACE_OUTER_BOUND('',#15100,.T.);
#11066=FACE_OUTER_BOUND('',#15101,.T.);
#11067=FACE_OUTER_BOUND('',#15102,.T.);
#11068=FACE_OUTER_BOUND('',#15103,.T.);
#11069=FACE_OUTER_BOUND('',#15104,.T.);
#11070=FACE_OUTER_BOUND('',#15105,.T.);
#11071=FACE_OUTER_BOUND('',#15106,.T.);
#11072=FACE_OUTER_BOUND('',#15107,.T.);
#11073=FACE_OUTER_BOUND('',#15108,.T.);
#11074=FACE_OUTER_BOUND('',#15109,.T.);
#11075=FACE_OUTER_BOUND('',#15110,.T.);
#11076=FACE_OUTER_BOUND('',#15111,.T.);
#11077=FACE_OUTER_BOUND('',#15112,.T.);
#11078=FACE_OUTER_BOUND('',#15113,.T.);
#11079=FACE_OUTER_BOUND('',#15114,.T.);
#11080=FACE_OUTER_BOUND('',#15115,.T.);
#11081=FACE_OUTER_BOUND('',#15116,.T.);
#11082=FACE_OUTER_BOUND('',#15117,.T.);
#11083=FACE_OUTER_BOUND('',#15118,.T.);
#11084=FACE_OUTER_BOUND('',#15119,.T.);
#11085=FACE_OUTER_BOUND('',#15120,.T.);
#11086=FACE_OUTER_BOUND('',#15121,.T.);
#11087=FACE_OUTER_BOUND('',#15122,.T.);
#11088=FACE_OUTER_BOUND('',#15123,.T.);
#11089=FACE_OUTER_BOUND('',#15124,.T.);
#11090=FACE_OUTER_BOUND('',#15126,.T.);
#11091=FACE_OUTER_BOUND('',#15127,.T.);
#11092=FACE_OUTER_BOUND('',#15128,.T.);
#11093=FACE_OUTER_BOUND('',#15129,.T.);
#11094=FACE_OUTER_BOUND('',#15130,.T.);
#11095=FACE_OUTER_BOUND('',#15131,.T.);
#11096=FACE_OUTER_BOUND('',#15132,.T.);
#11097=FACE_OUTER_BOUND('',#15133,.T.);
#11098=FACE_OUTER_BOUND('',#15134,.T.);
#11099=FACE_OUTER_BOUND('',#15138,.T.);
#11100=FACE_OUTER_BOUND('',#15139,.T.);
#11101=FACE_OUTER_BOUND('',#15140,.T.);
#11102=FACE_OUTER_BOUND('',#15141,.T.);
#11103=FACE_OUTER_BOUND('',#15142,.T.);
#11104=FACE_OUTER_BOUND('',#15143,.T.);
#11105=FACE_OUTER_BOUND('',#15144,.T.);
#11106=FACE_OUTER_BOUND('',#15145,.T.);
#11107=FACE_OUTER_BOUND('',#15146,.T.);
#11108=FACE_OUTER_BOUND('',#15147,.T.);
#11109=FACE_OUTER_BOUND('',#15148,.T.);
#11110=FACE_OUTER_BOUND('',#15149,.T.);
#11111=FACE_OUTER_BOUND('',#15150,.T.);
#11112=FACE_OUTER_BOUND('',#15151,.T.);
#11113=FACE_OUTER_BOUND('',#15152,.T.);
#11114=FACE_OUTER_BOUND('',#15153,.T.);
#11115=FACE_OUTER_BOUND('',#15154,.T.);
#11116=FACE_OUTER_BOUND('',#15155,.T.);
#11117=FACE_OUTER_BOUND('',#15156,.T.);
#11118=FACE_OUTER_BOUND('',#15157,.T.);
#11119=FACE_OUTER_BOUND('',#15158,.T.);
#11120=FACE_OUTER_BOUND('',#15159,.T.);
#11121=FACE_OUTER_BOUND('',#15160,.T.);
#11122=FACE_OUTER_BOUND('',#15161,.T.);
#14931=EDGE_LOOP('',(#35046,#35047,#35048,#35049));
#14932=EDGE_LOOP('',(#35050,#35051,#35052,#35053));
#14933=EDGE_LOOP('',(#35054,#35055,#35056,#35057));
#14934=EDGE_LOOP('',(#35058,#35059,#35060,#35061));
#14935=EDGE_LOOP('',(#35062,#35063,#35064,#35065));
#14936=EDGE_LOOP('',(#35066,#35067,#35068,#35069));
#14937=EDGE_LOOP('',(#35070,#35071,#35072,#35073));
#14938=EDGE_LOOP('',(#35074,#35075,#35076,#35077));
#14939=EDGE_LOOP('',(#35078,#35079,#35080,#35081));
#14940=EDGE_LOOP('',(#35082,#35083,#35084,#35085));
#14941=EDGE_LOOP('',(#35086,#35087,#35088,#35089));
#14942=EDGE_LOOP('',(#35090,#35091,#35092,#35093));
#14943=EDGE_LOOP('',(#35094,#35095,#35096,#35097,#35098,#35099,#35100,#35101,
#35102,#35103,#35104,#35105,#35106,#35107,#35108,#35109,#35110,#35111,#35112,
#35113,#35114));
#14944=EDGE_LOOP('',(#35115,#35116,#35117,#35118));
#14945=EDGE_LOOP('',(#35119,#35120,#35121,#35122,#35123,#35124));
#14946=EDGE_LOOP('',(#35125,#35126,#35127,#35128,#35129,#35130));
#14947=EDGE_LOOP('',(#35131,#35132,#35133,#35134,#35135,#35136));
#14948=EDGE_LOOP('',(#35137,#35138,#35139,#35140,#35141,#35142,#35143,#35144,
#35145,#35146,#35147));
#14949=EDGE_LOOP('',(#35148,#35149,#35150,#35151));
#14950=EDGE_LOOP('',(#35152,#35153,#35154,#35155));
#14951=EDGE_LOOP('',(#35156,#35157,#35158,#35159,#35160));
#14952=EDGE_LOOP('',(#35161,#35162,#35163,#35164));
#14953=EDGE_LOOP('',(#35165,#35166,#35167,#35168,#35169));
#14954=EDGE_LOOP('',(#35170,#35171,#35172,#35173,#35174,#35175,#35176,#35177,
#35178,#35179,#35180));
#14955=EDGE_LOOP('',(#35181,#35182,#35183,#35184));
#14956=EDGE_LOOP('',(#35185,#35186,#35187,#35188));
#14957=EDGE_LOOP('',(#35189,#35190,#35191,#35192,#35193));
#14958=EDGE_LOOP('',(#35194,#35195,#35196,#35197));
#14959=EDGE_LOOP('',(#35198,#35199,#35200,#35201,#35202));
#14960=EDGE_LOOP('',(#35203,#35204,#35205,#35206,#35207,#35208,#35209,#35210,
#35211,#35212,#35213));
#14961=EDGE_LOOP('',(#35214,#35215,#35216,#35217));
#14962=EDGE_LOOP('',(#35218,#35219,#35220,#35221));
#14963=EDGE_LOOP('',(#35222,#35223,#35224,#35225,#35226));
#14964=EDGE_LOOP('',(#35227,#35228,#35229,#35230));
#14965=EDGE_LOOP('',(#35231,#35232,#35233,#35234,#35235));
#14966=EDGE_LOOP('',(#35236,#35237,#35238,#35239,#35240,#35241,#35242,#35243,
#35244,#35245));
#14967=EDGE_LOOP('',(#35246,#35247,#35248,#35249,#35250));
#14968=EDGE_LOOP('',(#35251,#35252,#35253,#35254,#35255,#35256,#35257));
#14969=EDGE_LOOP('',(#35258,#35259,#35260,#35261));
#14970=EDGE_LOOP('',(#35262,#35263,#35264,#35265));
#14971=EDGE_LOOP('',(#35266,#35267,#35268,#35269));
#14972=EDGE_LOOP('',(#35270,#35271,#35272,#35273));
#14973=EDGE_LOOP('',(#35274,#35275,#35276,#35277));
#14974=EDGE_LOOP('',(#35278,#35279,#35280,#35281));
#14975=EDGE_LOOP('',(#35282,#35283,#35284,#35285));
#14976=EDGE_LOOP('',(#35286,#35287,#35288,#35289,#35290,#35291,#35292,#35293));
#14977=EDGE_LOOP('',(#35294,#35295,#35296,#35297));
#14978=EDGE_LOOP('',(#35298,#35299,#35300,#35301));
#14979=EDGE_LOOP('',(#35302,#35303,#35304,#35305));
#14980=EDGE_LOOP('',(#35306,#35307,#35308,#35309,#35310));
#14981=EDGE_LOOP('',(#35311,#35312,#35313,#35314,#35315));
#14982=EDGE_LOOP('',(#35316,#35317,#35318,#35319,#35320,#35321));
#14983=EDGE_LOOP('',(#35322,#35323,#35324,#35325));
#14984=EDGE_LOOP('',(#35326,#35327,#35328,#35329));
#14985=EDGE_LOOP('',(#35330,#35331,#35332,#35333));
#14986=EDGE_LOOP('',(#35334,#35335,#35336,#35337));
#14987=EDGE_LOOP('',(#35338,#35339,#35340,#35341));
#14988=EDGE_LOOP('',(#35342,#35343,#35344));
#14989=EDGE_LOOP('',(#35345,#35346,#35347));
#14990=EDGE_LOOP('',(#35348,#35349,#35350,#35351));
#14991=EDGE_LOOP('',(#35352,#35353,#35354,#35355));
#14992=EDGE_LOOP('',(#35356,#35357,#35358,#35359));
#14993=EDGE_LOOP('',(#35360,#35361,#35362,#35363));
#14994=EDGE_LOOP('',(#35364,#35365,#35366,#35367));
#14995=EDGE_LOOP('',(#35368,#35369,#35370,#35371));
#14996=EDGE_LOOP('',(#35372,#35373,#35374,#35375));
#14997=EDGE_LOOP('',(#35376,#35377,#35378,#35379));
#14998=EDGE_LOOP('',(#35380,#35381,#35382,#35383));
#14999=EDGE_LOOP('',(#35384,#35385,#35386,#35387));
#15000=EDGE_LOOP('',(#35388,#35389,#35390,#35391));
#15001=EDGE_LOOP('',(#35392,#35393,#35394,#35395));
#15002=EDGE_LOOP('',(#35396,#35397,#35398,#35399));
#15003=EDGE_LOOP('',(#35400,#35401,#35402,#35403));
#15004=EDGE_LOOP('',(#35404,#35405,#35406,#35407));
#15005=EDGE_LOOP('',(#35408,#35409,#35410,#35411));
#15006=EDGE_LOOP('',(#35412,#35413,#35414,#35415));
#15007=EDGE_LOOP('',(#35416,#35417,#35418,#35419));
#15008=EDGE_LOOP('',(#35420,#35421,#35422,#35423));
#15009=EDGE_LOOP('',(#35424,#35425,#35426,#35427));
#15010=EDGE_LOOP('',(#35428,#35429,#35430,#35431));
#15011=EDGE_LOOP('',(#35432,#35433,#35434,#35435));
#15012=EDGE_LOOP('',(#35436,#35437,#35438,#35439));
#15013=EDGE_LOOP('',(#35440,#35441,#35442,#35443));
#15014=EDGE_LOOP('',(#35444,#35445,#35446,#35447));
#15015=EDGE_LOOP('',(#35448,#35449,#35450,#35451));
#15016=EDGE_LOOP('',(#35452,#35453,#35454,#35455));
#15017=EDGE_LOOP('',(#35456,#35457,#35458,#35459,#35460,#35461,#35462));
#15018=EDGE_LOOP('',(#35463,#35464,#35465,#35466,#35467,#35468,#35469));
#15019=EDGE_LOOP('',(#35470,#35471,#35472,#35473));
#15020=EDGE_LOOP('',(#35474,#35475,#35476,#35477));
#15021=EDGE_LOOP('',(#35478,#35479,#35480,#35481));
#15022=EDGE_LOOP('',(#35482,#35483,#35484,#35485));
#15023=EDGE_LOOP('',(#35486,#35487,#35488,#35489));
#15024=EDGE_LOOP('',(#35490,#35491,#35492,#35493));
#15025=EDGE_LOOP('',(#35494,#35495,#35496,#35497));
#15026=EDGE_LOOP('',(#35498,#35499,#35500,#35501));
#15027=EDGE_LOOP('',(#35502,#35503,#35504,#35505));
#15028=EDGE_LOOP('',(#35506,#35507,#35508,#35509));
#15029=EDGE_LOOP('',(#35510,#35511,#35512,#35513));
#15030=EDGE_LOOP('',(#35514,#35515,#35516,#35517));
#15031=EDGE_LOOP('',(#35518,#35519,#35520,#35521));
#15032=EDGE_LOOP('',(#35522,#35523,#35524,#35525));
#15033=EDGE_LOOP('',(#35526,#35527,#35528,#35529));
#15034=EDGE_LOOP('',(#35530,#35531,#35532,#35533));
#15035=EDGE_LOOP('',(#35534,#35535,#35536,#35537));
#15036=EDGE_LOOP('',(#35538,#35539,#35540,#35541));
#15037=EDGE_LOOP('',(#35542,#35543,#35544,#35545));
#15038=EDGE_LOOP('',(#35546,#35547,#35548,#35549,#35550,#35551,#35552));
#15039=EDGE_LOOP('',(#35553,#35554,#35555,#35556,#35557,#35558,#35559));
#15040=EDGE_LOOP('',(#35560,#35561,#35562,#35563));
#15041=EDGE_LOOP('',(#35564,#35565,#35566,#35567));
#15042=EDGE_LOOP('',(#35568,#35569,#35570,#35571));
#15043=EDGE_LOOP('',(#35572,#35573,#35574,#35575));
#15044=EDGE_LOOP('',(#35576,#35577,#35578,#35579));
#15045=EDGE_LOOP('',(#35580,#35581,#35582,#35583));
#15046=EDGE_LOOP('',(#35584,#35585,#35586,#35587));
#15047=EDGE_LOOP('',(#35588,#35589,#35590,#35591));
#15048=EDGE_LOOP('',(#35592,#35593,#35594,#35595));
#15049=EDGE_LOOP('',(#35596,#35597,#35598,#35599));
#15050=EDGE_LOOP('',(#35600,#35601,#35602,#35603));
#15051=EDGE_LOOP('',(#35604,#35605,#35606,#35607));
#15052=EDGE_LOOP('',(#35608,#35609,#35610,#35611));
#15053=EDGE_LOOP('',(#35612,#35613,#35614,#35615));
#15054=EDGE_LOOP('',(#35616,#35617,#35618,#35619));
#15055=EDGE_LOOP('',(#35620,#35621,#35622,#35623));
#15056=EDGE_LOOP('',(#35624,#35625,#35626,#35627));
#15057=EDGE_LOOP('',(#35628,#35629,#35630,#35631));
#15058=EDGE_LOOP('',(#35632,#35633,#35634,#35635));
#15059=EDGE_LOOP('',(#35636,#35637,#35638,#35639,#35640,#35641,#35642));
#15060=EDGE_LOOP('',(#35643,#35644,#35645,#35646,#35647,#35648,#35649));
#15061=EDGE_LOOP('',(#35650,#35651,#35652,#35653));
#15062=EDGE_LOOP('',(#35654,#35655,#35656,#35657));
#15063=EDGE_LOOP('',(#35658,#35659,#35660,#35661));
#15064=EDGE_LOOP('',(#35662,#35663,#35664,#35665));
#15065=EDGE_LOOP('',(#35666,#35667,#35668,#35669));
#15066=EDGE_LOOP('',(#35670,#35671,#35672,#35673));
#15067=EDGE_LOOP('',(#35674,#35675,#35676,#35677));
#15068=EDGE_LOOP('',(#35678,#35679,#35680,#35681));
#15069=EDGE_LOOP('',(#35682,#35683,#35684,#35685));
#15070=EDGE_LOOP('',(#35686,#35687,#35688,#35689));
#15071=EDGE_LOOP('',(#35690,#35691,#35692,#35693));
#15072=EDGE_LOOP('',(#35694,#35695,#35696,#35697));
#15073=EDGE_LOOP('',(#35698,#35699,#35700,#35701));
#15074=EDGE_LOOP('',(#35702,#35703,#35704,#35705));
#15075=EDGE_LOOP('',(#35706,#35707,#35708,#35709));
#15076=EDGE_LOOP('',(#35710,#35711,#35712,#35713));
#15077=EDGE_LOOP('',(#35714,#35715,#35716,#35717));
#15078=EDGE_LOOP('',(#35718,#35719,#35720,#35721));
#15079=EDGE_LOOP('',(#35722,#35723,#35724,#35725));
#15080=EDGE_LOOP('',(#35726,#35727,#35728,#35729,#35730,#35731,#35732));
#15081=EDGE_LOOP('',(#35733,#35734,#35735,#35736,#35737,#35738,#35739));
#15082=EDGE_LOOP('',(#35740,#35741,#35742,#35743));
#15083=EDGE_LOOP('',(#35744,#35745));
#15084=EDGE_LOOP('',(#35746,#35747));
#15085=EDGE_LOOP('',(#35748,#35749));
#15086=EDGE_LOOP('',(#35750,#35751,#35752,#35753));
#15087=EDGE_LOOP('',(#35754,#35755,#35756,#35757));
#15088=EDGE_LOOP('',(#35758,#35759,#35760,#35761,#35762,#35763));
#15089=EDGE_LOOP('',(#35764,#35765,#35766,#35767));
#15090=EDGE_LOOP('',(#35768,#35769,#35770,#35771));
#15091=EDGE_LOOP('',(#35772,#35773,#35774,#35775));
#15092=EDGE_LOOP('',(#35776,#35777,#35778,#35779,#35780,#35781));
#15093=EDGE_LOOP('',(#35782,#35783,#35784,#35785));
#15094=EDGE_LOOP('',(#35786,#35787,#35788,#35789));
#15095=EDGE_LOOP('',(#35790,#35791,#35792,#35793));
#15096=EDGE_LOOP('',(#35794,#35795,#35796,#35797));
#15097=EDGE_LOOP('',(#35798,#35799,#35800,#35801));
#15098=EDGE_LOOP('',(#35802,#35803,#35804,#35805));
#15099=EDGE_LOOP('',(#35806,#35807,#35808,#35809));
#15100=EDGE_LOOP('',(#35810,#35811,#35812,#35813));
#15101=EDGE_LOOP('',(#35814,#35815,#35816,#35817));
#15102=EDGE_LOOP('',(#35818,#35819,#35820,#35821));
#15103=EDGE_LOOP('',(#35822,#35823,#35824,#35825));
#15104=EDGE_LOOP('',(#35826,#35827,#35828,#35829));
#15105=EDGE_LOOP('',(#35830,#35831,#35832,#35833));
#15106=EDGE_LOOP('',(#35834,#35835,#35836,#35837));
#15107=EDGE_LOOP('',(#35838,#35839,#35840,#35841));
#15108=EDGE_LOOP('',(#35842,#35843,#35844,#35845));
#15109=EDGE_LOOP('',(#35846,#35847,#35848,#35849));
#15110=EDGE_LOOP('',(#35850,#35851,#35852,#35853));
#15111=EDGE_LOOP('',(#35854,#35855,#35856,#35857));
#15112=EDGE_LOOP('',(#35858,#35859,#35860));
#15113=EDGE_LOOP('',(#35861,#35862,#35863,#35864));
#15114=EDGE_LOOP('',(#35865,#35866,#35867,#35868));
#15115=EDGE_LOOP('',(#35869,#35870,#35871));
#15116=EDGE_LOOP('',(#35872,#35873,#35874,#35875,#35876));
#15117=EDGE_LOOP('',(#35877,#35878,#35879,#35880));
#15118=EDGE_LOOP('',(#35881,#35882,#35883,#35884));
#15119=EDGE_LOOP('',(#35885,#35886,#35887,#35888));
#15120=EDGE_LOOP('',(#35889,#35890,#35891,#35892,#35893));
#15121=EDGE_LOOP('',(#35894,#35895,#35896,#35897,#35898));
#15122=EDGE_LOOP('',(#35899,#35900,#35901,#35902));
#15123=EDGE_LOOP('',(#35903,#35904,#35905,#35906,#35907));
#15124=EDGE_LOOP('',(#35908));
#15125=EDGE_LOOP('',(#35909));
#15126=EDGE_LOOP('',(#35910,#35911,#35912,#35913));
#15127=EDGE_LOOP('',(#35914,#35915,#35916,#35917));
#15128=EDGE_LOOP('',(#35918,#35919,#35920,#35921));
#15129=EDGE_LOOP('',(#35922,#35923,#35924,#35925));
#15130=EDGE_LOOP('',(#35926,#35927,#35928,#35929));
#15131=EDGE_LOOP('',(#35930,#35931,#35932,#35933));
#15132=EDGE_LOOP('',(#35934,#35935,#35936,#35937));
#15133=EDGE_LOOP('',(#35938,#35939,#35940,#35941));
#15134=EDGE_LOOP('',(#35942,#35943,#35944,#35945,#35946,#35947,#35948,#35949,
#35950,#35951,#35952));
#15135=EDGE_LOOP('',(#35953));
#15136=EDGE_LOOP('',(#35954));
#15137=EDGE_LOOP('',(#35955));
#15138=EDGE_LOOP('',(#35956,#35957,#35958,#35959));
#15139=EDGE_LOOP('',(#35960,#35961,#35962,#35963,#35964,#35965,#35966));
#15140=EDGE_LOOP('',(#35967,#35968,#35969,#35970,#35971,#35972,#35973));
#15141=EDGE_LOOP('',(#35974,#35975,#35976,#35977));
#15142=EDGE_LOOP('',(#35978,#35979,#35980,#35981));
#15143=EDGE_LOOP('',(#35982,#35983,#35984,#35985));
#15144=EDGE_LOOP('',(#35986,#35987,#35988,#35989,#35990,#35991,#35992,#35993,
#35994));
#15145=EDGE_LOOP('',(#35995,#35996,#35997,#35998));
#15146=EDGE_LOOP('',(#35999,#36000,#36001,#36002));
#15147=EDGE_LOOP('',(#36003,#36004,#36005,#36006,#36007));
#15148=EDGE_LOOP('',(#36008,#36009,#36010,#36011,#36012));
#15149=EDGE_LOOP('',(#36013,#36014,#36015,#36016));
#15150=EDGE_LOOP('',(#36017,#36018,#36019,#36020));
#15151=EDGE_LOOP('',(#36021,#36022,#36023,#36024));
#15152=EDGE_LOOP('',(#36025,#36026,#36027,#36028));
#15153=EDGE_LOOP('',(#36029,#36030,#36031));
#15154=EDGE_LOOP('',(#36032,#36033,#36034,#36035));
#15155=EDGE_LOOP('',(#36036,#36037,#36038,#36039));
#15156=EDGE_LOOP('',(#36040,#36041,#36042,#36043));
#15157=EDGE_LOOP('',(#36044,#36045,#36046,#36047));
#15158=EDGE_LOOP('',(#36048,#36049,#36050,#36051));
#15159=EDGE_LOOP('',(#36052,#36053,#36054,#36055));
#15160=EDGE_LOOP('',(#36056,#36057,#36058,#36059));
#15161=EDGE_LOOP('',(#36060,#36061,#36062,#36063,#36064,#36065,#36066,#36067,
#36068,#36069,#36070,#36071,#36072,#36073,#36074,#36075));
#18972=CIRCLE('',#48164,0.500000000000028);
#18973=CIRCLE('',#48165,0.500000000000028);
#18974=CIRCLE('',#48168,0.499999999999973);
#18975=CIRCLE('',#48169,0.499999999999973);
#18976=CIRCLE('',#48174,0.500000000000028);
#18977=CIRCLE('',#48175,0.499999999999973);
#18978=CIRCLE('',#48178,0.499999999999973);
#18979=CIRCLE('',#48181,0.500000000000028);
#18980=CIRCLE('',#48184,28.5226030790361);
#18981=CIRCLE('',#48185,28.5226030790361);
#18982=CIRCLE('',#48186,28.5226030790361);
#18983=CIRCLE('',#48187,27.5913762017691);
#18984=CIRCLE('',#48188,28.5226030790361);
#18985=CIRCLE('',#48189,1.86064640637173);
#18986=CIRCLE('',#48191,1.);
#18987=CIRCLE('',#48192,27.5226030790361);
#18988=CIRCLE('',#48194,16.5);
#18989=CIRCLE('',#48195,16.5);
#18990=CIRCLE('',#48197,16.5);
#18991=CIRCLE('',#48198,16.5);
#18992=CIRCLE('',#48200,16.5);
#18993=CIRCLE('',#48201,16.5);
#18994=CIRCLE('',#48203,16.);
#18995=CIRCLE('',#48204,16.);
#18996=CIRCLE('',#48205,16.);
#18997=CIRCLE('',#48206,16.);
#18998=CIRCLE('',#48207,16.);
#18999=CIRCLE('',#48209,3.96802221877415);
#19000=CIRCLE('',#48210,3.96802221877415);
#19001=CIRCLE('',#48212,0.5);
#19002=CIRCLE('',#48213,4.46802221877415);
#19003=CIRCLE('',#48214,0.5);
#19004=CIRCLE('',#48216,15.5);
#19005=CIRCLE('',#48218,0.5);
#19006=CIRCLE('',#48219,3.46802221877415);
#19007=CIRCLE('',#48220,0.5);
#19008=CIRCLE('',#48222,0.5);
#19009=CIRCLE('',#48223,15.5);
#19010=CIRCLE('',#48225,16.);
#19011=CIRCLE('',#48226,16.);
#19012=CIRCLE('',#48227,16.);
#19013=CIRCLE('',#48228,16.);
#19014=CIRCLE('',#48229,16.);
#19015=CIRCLE('',#48231,3.96802221877416);
#19016=CIRCLE('',#48232,3.96802221877416);
#19017=CIRCLE('',#48234,0.5);
#19018=CIRCLE('',#48235,4.46802221877416);
#19019=CIRCLE('',#48236,0.5);
#19020=CIRCLE('',#48238,15.5);
#19021=CIRCLE('',#48240,0.5);
#19022=CIRCLE('',#48241,3.46802221877416);
#19023=CIRCLE('',#48242,0.5);
#19024=CIRCLE('',#48244,0.5);
#19025=CIRCLE('',#48245,15.5);
#19026=CIRCLE('',#48247,16.);
#19027=CIRCLE('',#48248,16.);
#19028=CIRCLE('',#48249,16.);
#19029=CIRCLE('',#48250,16.);
#19030=CIRCLE('',#48251,16.);
#19031=CIRCLE('',#48253,3.96802221877416);
#19032=CIRCLE('',#48254,3.96802221877416);
#19033=CIRCLE('',#48256,0.5);
#19034=CIRCLE('',#48257,4.46802221877416);
#19035=CIRCLE('',#48258,0.5);
#19036=CIRCLE('',#48260,15.5);
#19037=CIRCLE('',#48262,0.5);
#19038=CIRCLE('',#48263,3.46802221877416);
#19039=CIRCLE('',#48264,0.5);
#19040=CIRCLE('',#48266,0.5);
#19041=CIRCLE('',#48267,15.5);
#19042=CIRCLE('',#48269,26.0226030790361);
#19043=CIRCLE('',#48270,26.0226030790361);
#19044=CIRCLE('',#48271,26.0226030790361);
#19045=CIRCLE('',#48272,26.0226030790361);
#19046=CIRCLE('',#48274,25.3226030790361);
#19047=CIRCLE('',#48276,29.5);
#19048=CIRCLE('',#48277,29.5);
#19049=CIRCLE('',#48279,30.);
#19050=CIRCLE('',#48280,30.);
#19051=CIRCLE('',#48282,30.);
#19052=CIRCLE('',#48283,30.);
#19053=CIRCLE('',#48287,0.500000000000003);
#19054=CIRCLE('',#48288,0.5);
#19055=CIRCLE('',#48289,0.500000000000003);
#19056=CIRCLE('',#48291,29.7179449471771);
#19057=CIRCLE('',#48292,0.5);
#19058=CIRCLE('',#48294,29.7179449471771);
#19059=CIRCLE('',#48295,0.5);
#19060=CIRCLE('',#48297,0.5);
#19061=CIRCLE('',#48299,0.5);
#19062=CIRCLE('',#48301,0.5);
#19063=CIRCLE('',#48302,0.5);
#19064=CIRCLE('',#48304,0.5);
#19065=CIRCLE('',#48306,0.5);
#19066=CIRCLE('',#48308,0.5);
#19067=CIRCLE('',#48310,0.5);
#19068=CIRCLE('',#48312,0.5);
#19069=CIRCLE('',#48313,0.5);
#19070=CIRCLE('',#48315,0.5);
#19071=CIRCLE('',#48317,0.5);
#19072=CIRCLE('',#48319,0.5);
#19073=CIRCLE('',#48321,0.5);
#19074=CIRCLE('',#48323,0.500000000000003);
#19075=CIRCLE('',#48325,0.500000000000003);
#19076=CIRCLE('',#48326,0.5);
#19077=CIRCLE('',#48328,0.700000000000006);
#19078=CIRCLE('',#48329,4.75563473233925);
#19079=CIRCLE('',#48330,0.700000000000006);
#19080=CIRCLE('',#48331,4.05563473233925);
#19081=CIRCLE('',#48333,0.700000000000006);
#19082=CIRCLE('',#48335,0.700000000000006);
#19083=CIRCLE('',#48337,4.75563473233925);
#19084=CIRCLE('',#48338,4.05563473233925);
#19085=CIRCLE('',#48340,0.700000000000006);
#19086=CIRCLE('',#48341,0.700000000000006);
#19087=CIRCLE('',#48342,0.699999999999998);
#19088=CIRCLE('',#48343,0.700000000000006);
#19089=CIRCLE('',#48345,0.700000000000006);
#19090=CIRCLE('',#48347,0.7);
#19091=CIRCLE('',#48348,26.7226030790361);
#19092=CIRCLE('',#48350,0.700000000000006);
#19093=CIRCLE('',#48352,0.700000000000006);
#19094=CIRCLE('',#48353,4.05563473233925);
#19095=CIRCLE('',#48354,4.75563473233925);
#19096=CIRCLE('',#48355,0.700000000000006);
#19097=CIRCLE('',#48356,0.700000000000006);
#19098=CIRCLE('',#48357,0.700000000000006);
#19099=CIRCLE('',#48359,0.700000000000006);
#19100=CIRCLE('',#48360,4.75563473233925);
#19101=CIRCLE('',#48361,5.45563473233926);
#19102=CIRCLE('',#48373,0.499999999999999);
#19103=CIRCLE('',#48375,0.5);
#19104=CIRCLE('',#48376,3.96802221877416);
#19105=CIRCLE('',#48377,3.46802221877416);
#19106=CIRCLE('',#48380,0.500000000000001);
#19107=CIRCLE('',#48381,0.5);
#19108=CIRCLE('',#48382,16.5);
#19109=CIRCLE('',#48383,0.5);
#19110=CIRCLE('',#48384,0.5);
#19111=CIRCLE('',#48386,0.5);
#19112=CIRCLE('',#48388,0.499999999999999);
#19113=CIRCLE('',#48390,0.5);
#19114=CIRCLE('',#48392,0.5);
#19115=CIRCLE('',#48393,0.499999999999999);
#19116=CIRCLE('',#48395,3.96802221877416);
#19117=CIRCLE('',#48396,3.46802221877416);
#19118=CIRCLE('',#48397,0.499999999999998);
#19119=CIRCLE('',#48407,0.500000000000001);
#19120=CIRCLE('',#48409,0.500000000000003);
#19121=CIRCLE('',#48410,3.96802221877416);
#19122=CIRCLE('',#48411,3.46802221877416);
#19123=CIRCLE('',#48414,0.499999999999999);
#19124=CIRCLE('',#48415,0.5);
#19125=CIRCLE('',#48416,16.5);
#19126=CIRCLE('',#48417,0.5);
#19127=CIRCLE('',#48418,0.5);
#19128=CIRCLE('',#48420,0.5);
#19129=CIRCLE('',#48422,0.500000000000002);
#19130=CIRCLE('',#48424,0.5);
#19131=CIRCLE('',#48426,0.5);
#19132=CIRCLE('',#48427,0.500000000000003);
#19133=CIRCLE('',#48429,3.96802221877416);
#19134=CIRCLE('',#48430,3.46802221877416);
#19135=CIRCLE('',#48431,0.5);
#19136=CIRCLE('',#48441,0.500000000000001);
#19137=CIRCLE('',#48443,0.500000000000003);
#19138=CIRCLE('',#48444,3.96802221877415);
#19139=CIRCLE('',#48445,3.46802221877417);
#19140=CIRCLE('',#48448,0.499999999999999);
#19141=CIRCLE('',#48449,0.5);
#19142=CIRCLE('',#48450,16.5);
#19143=CIRCLE('',#48451,0.5);
#19144=CIRCLE('',#48452,0.5);
#19145=CIRCLE('',#48454,0.5);
#19146=CIRCLE('',#48456,0.500000000000002);
#19147=CIRCLE('',#48458,0.5);
#19148=CIRCLE('',#48460,0.5);
#19149=CIRCLE('',#48461,0.499999999999997);
#19150=CIRCLE('',#48463,3.96802221877415);
#19151=CIRCLE('',#48464,3.46802221877417);
#19152=CIRCLE('',#48465,0.5);
#19153=CIRCLE('',#48478,0.5);
#19154=CIRCLE('',#48479,0.5);
#19155=CIRCLE('',#48481,0.500000000000003);
#19156=CIRCLE('',#48482,30.);
#19157=CIRCLE('',#48483,1.);
#19158=CIRCLE('',#48484,0.5);
#19159=CIRCLE('',#48485,0.499999999999988);
#19160=CIRCLE('',#48487,0.5);
#19161=CIRCLE('',#48488,0.500000000000011);
#19162=CIRCLE('',#48489,0.5);
#19163=CIRCLE('',#48490,1.);
#19164=CIRCLE('',#48491,0.499999999999989);
#19165=CIRCLE('',#48493,0.5);
#19166=CIRCLE('',#48494,0.499999999999993);
#19167=CIRCLE('',#48496,0.500000000000003);
#19168=CIRCLE('',#48497,30.);
#19169=CIRCLE('',#48498,0.5);
#19170=CIRCLE('',#48500,1.);
#19171=CIRCLE('',#48501,1.);
#19172=CIRCLE('',#48502,1.);
#19173=CIRCLE('',#48504,1.);
#19174=CIRCLE('',#48505,1.);
#19175=CIRCLE('',#48506,2.);
#19176=CIRCLE('',#48508,0.999999999999994);
#19177=CIRCLE('',#48509,27.5226030790361);
#19178=CIRCLE('',#48511,1.);
#19179=CIRCLE('',#48513,1.);
#19180=CIRCLE('',#48514,1.);
#19181=CIRCLE('',#48515,2.);
#19182=CIRCLE('',#48516,0.999999999999999);
#19183=CIRCLE('',#48517,1.);
#19184=CIRCLE('',#48519,1.);
#19185=CIRCLE('',#48521,1.);
#19186=CIRCLE('',#48522,29.5226030790361);
#19187=CIRCLE('',#48524,0.999999999999999);
#19188=CIRCLE('',#48526,1.);
#19189=CIRCLE('',#48527,1.);
#19190=CIRCLE('',#48529,1.);
#19191=CIRCLE('',#48530,29.5226030790361);
#19192=CIRCLE('',#48532,1.);
#19193=CIRCLE('',#48534,1.);
#19194=CIRCLE('',#48535,1.);
#19195=CIRCLE('',#48536,1.00000000000001);
#19196=CIRCLE('',#48538,1.);
#19197=CIRCLE('',#48539,1.00000000000001);
#19198=CIRCLE('',#48540,1.);
#19199=CIRCLE('',#48541,0.99999999999999);
#19200=CIRCLE('',#48542,1.00000000000001);
#19201=CIRCLE('',#48543,0.999999999999988);
#19202=CIRCLE('',#48545,1.);
#19203=CIRCLE('',#48546,1.);
#19204=CIRCLE('',#48547,1.00000000000001);
#19205=CIRCLE('',#48548,1.);
#19206=CIRCLE('',#48549,32.4650886384815);
#19207=CIRCLE('',#48550,33.3654637529391);
#19208=CIRCLE('',#48551,0.999999999999998);
#19209=CIRCLE('',#48552,1.);
#19210=CIRCLE('',#48553,1.);
#19211=CIRCLE('',#48554,1.);
#19212=CIRCLE('',#48555,33.3726238561351);
#19213=CIRCLE('',#48556,32.4650889393932);
#19214=CIRCLE('',#48559,30.);
#19215=CIRCLE('',#48560,30.);
#19216=CIRCLE('',#48561,30.);
#22215=VERTEX_POINT('',#85908);
#22216=VERTEX_POINT('',#85909);
#22217=VERTEX_POINT('',#85911);
#22218=VERTEX_POINT('',#85913);
#22219=VERTEX_POINT('',#85917);
#22220=VERTEX_POINT('',#85918);
#22221=VERTEX_POINT('',#85923);
#22222=VERTEX_POINT('',#85924);
#22223=VERTEX_POINT('',#85934);
#22224=VERTEX_POINT('',#85935);
#22225=VERTEX_POINT('',#85937);
#22226=VERTEX_POINT('',#85939);
#22227=VERTEX_POINT('',#85943);
#22228=VERTEX_POINT('',#85945);
#22229=VERTEX_POINT('',#85949);
#22230=VERTEX_POINT('',#85953);
#22231=VERTEX_POINT('',#85960);
#22232=VERTEX_POINT('',#85961);
#22233=VERTEX_POINT('',#86017);
#22234=VERTEX_POINT('',#86019);
#22235=VERTEX_POINT('',#86021);
#22236=VERTEX_POINT('',#86080);
#22237=VERTEX_POINT('',#86082);
#22238=VERTEX_POINT('',#86084);
#22239=VERTEX_POINT('',#86086);
#22240=VERTEX_POINT('',#86142);
#22241=VERTEX_POINT('',#86144);
#22242=VERTEX_POINT('',#86146);
#22243=VERTEX_POINT('',#86184);
#22244=VERTEX_POINT('',#86186);
#22245=VERTEX_POINT('',#86189);
#22246=VERTEX_POINT('',#86202);
#22247=VERTEX_POINT('',#86267);
#22248=VERTEX_POINT('',#86274);
#22249=VERTEX_POINT('',#86369);
#22250=VERTEX_POINT('',#86379);
#22251=VERTEX_POINT('',#86383);
#22252=VERTEX_POINT('',#86384);
#22253=VERTEX_POINT('',#86386);
#22254=VERTEX_POINT('',#86388);
#22255=VERTEX_POINT('',#86399);
#22256=VERTEX_POINT('',#86401);
#22257=VERTEX_POINT('',#86414);
#22258=VERTEX_POINT('',#86415);
#22259=VERTEX_POINT('',#86417);
#22260=VERTEX_POINT('',#86419);
#22261=VERTEX_POINT('',#86430);
#22262=VERTEX_POINT('',#86432);
#22263=VERTEX_POINT('',#86445);
#22264=VERTEX_POINT('',#86446);
#22265=VERTEX_POINT('',#86448);
#22266=VERTEX_POINT('',#86450);
#22267=VERTEX_POINT('',#86461);
#22268=VERTEX_POINT('',#86463);
#22269=VERTEX_POINT('',#86476);
#22270=VERTEX_POINT('',#86477);
#22271=VERTEX_POINT('',#86479);
#22272=VERTEX_POINT('',#86481);
#22273=VERTEX_POINT('',#86483);
#22274=VERTEX_POINT('',#86485);
#22275=VERTEX_POINT('',#86535);
#22276=VERTEX_POINT('',#86537);
#22277=VERTEX_POINT('',#86596);
#22278=VERTEX_POINT('',#86601);
#22279=VERTEX_POINT('',#86602);
#22280=VERTEX_POINT('',#86604);
#22281=VERTEX_POINT('',#86606);
#22282=VERTEX_POINT('',#86610);
#22283=VERTEX_POINT('',#86612);
#22284=VERTEX_POINT('',#86616);
#22285=VERTEX_POINT('',#86660);
#22286=VERTEX_POINT('',#86709);
#22287=VERTEX_POINT('',#86711);
#22288=VERTEX_POINT('',#86715);
#22289=VERTEX_POINT('',#86719);
#22290=VERTEX_POINT('',#86720);
#22291=VERTEX_POINT('',#86722);
#22292=VERTEX_POINT('',#86724);
#22293=VERTEX_POINT('',#86726);
#22294=VERTEX_POINT('',#86728);
#22295=VERTEX_POINT('',#86778);
#22296=VERTEX_POINT('',#86780);
#22297=VERTEX_POINT('',#86839);
#22298=VERTEX_POINT('',#86844);
#22299=VERTEX_POINT('',#86845);
#22300=VERTEX_POINT('',#86847);
#22301=VERTEX_POINT('',#86849);
#22302=VERTEX_POINT('',#86853);
#22303=VERTEX_POINT('',#86855);
#22304=VERTEX_POINT('',#86859);
#22305=VERTEX_POINT('',#86903);
#22306=VERTEX_POINT('',#86952);
#22307=VERTEX_POINT('',#86954);
#22308=VERTEX_POINT('',#86958);
#22309=VERTEX_POINT('',#86962);
#22310=VERTEX_POINT('',#86963);
#22311=VERTEX_POINT('',#86965);
#22312=VERTEX_POINT('',#86967);
#22313=VERTEX_POINT('',#86969);
#22314=VERTEX_POINT('',#86971);
#22315=VERTEX_POINT('',#87021);
#22316=VERTEX_POINT('',#87023);
#22317=VERTEX_POINT('',#87082);
#22318=VERTEX_POINT('',#87087);
#22319=VERTEX_POINT('',#87088);
#22320=VERTEX_POINT('',#87090);
#22321=VERTEX_POINT('',#87092);
#22322=VERTEX_POINT('',#87096);
#22323=VERTEX_POINT('',#87098);
#22324=VERTEX_POINT('',#87102);
#22325=VERTEX_POINT('',#87146);
#22326=VERTEX_POINT('',#87195);
#22327=VERTEX_POINT('',#87197);
#22328=VERTEX_POINT('',#87201);
#22329=VERTEX_POINT('',#87205);
#22330=VERTEX_POINT('',#87207);
#22331=VERTEX_POINT('',#87209);
#22332=VERTEX_POINT('',#87211);
#22333=VERTEX_POINT('',#87213);
#22334=VERTEX_POINT('',#87272);
#22335=VERTEX_POINT('',#87274);
#22336=VERTEX_POINT('',#87330);
#22337=VERTEX_POINT('',#87334);
#22338=VERTEX_POINT('',#87384);
#22339=VERTEX_POINT('',#87430);
#22340=VERTEX_POINT('',#87431);
#22341=VERTEX_POINT('',#87433);
#22342=VERTEX_POINT('',#87519);
#22343=VERTEX_POINT('',#87602);
#22344=VERTEX_POINT('',#87604);
#22345=VERTEX_POINT('',#87606);
#22346=VERTEX_POINT('',#87610);
#22347=VERTEX_POINT('',#87611);
#22348=VERTEX_POINT('',#87613);
#22349=VERTEX_POINT('',#87615);
#22350=VERTEX_POINT('',#87626);
#22351=VERTEX_POINT('',#87627);
#22352=VERTEX_POINT('',#88055);
#22353=VERTEX_POINT('',#88056);
#22354=VERTEX_POINT('',#88058);
#22355=VERTEX_POINT('',#88060);
#22356=VERTEX_POINT('',#88497);
#22357=VERTEX_POINT('',#88498);
#22358=VERTEX_POINT('',#88500);
#22359=VERTEX_POINT('',#88502);
#22360=VERTEX_POINT('',#88506);
#22361=VERTEX_POINT('',#88508);
#22362=VERTEX_POINT('',#88512);
#22363=VERTEX_POINT('',#88513);
#22364=VERTEX_POINT('',#88691);
#22365=VERTEX_POINT('',#88692);
#22366=VERTEX_POINT('',#88733);
#22367=VERTEX_POINT('',#88738);
#22368=VERTEX_POINT('',#88757);
#22369=VERTEX_POINT('',#88783);
#22370=VERTEX_POINT('',#88996);
#22371=VERTEX_POINT('',#89267);
#22372=VERTEX_POINT('',#89271);
#22373=VERTEX_POINT('',#89275);
#22374=VERTEX_POINT('',#89276);
#22375=VERTEX_POINT('',#89286);
#22376=VERTEX_POINT('',#89288);
#22377=VERTEX_POINT('',#89299);
#22378=VERTEX_POINT('',#89300);
#22379=VERTEX_POINT('',#89308);
#22380=VERTEX_POINT('',#89310);
#22381=VERTEX_POINT('',#89699);
#22382=VERTEX_POINT('',#89700);
#22383=VERTEX_POINT('',#89702);
#22384=VERTEX_POINT('',#89704);
#22385=VERTEX_POINT('',#89708);
#22386=VERTEX_POINT('',#89709);
#22387=VERTEX_POINT('',#89714);
#22388=VERTEX_POINT('',#89715);
#22389=VERTEX_POINT('',#89723);
#22390=VERTEX_POINT('',#89725);
#22391=VERTEX_POINT('',#89764);
#22392=VERTEX_POINT('',#89845);
#22393=VERTEX_POINT('',#89903);
#22394=VERTEX_POINT('',#89904);
#22395=VERTEX_POINT('',#89909);
#22396=VERTEX_POINT('',#89913);
#22397=VERTEX_POINT('',#89914);
#22398=VERTEX_POINT('',#89919);
#22399=VERTEX_POINT('',#89920);
#22400=VERTEX_POINT('',#89960);
#22401=VERTEX_POINT('',#90041);
#22402=VERTEX_POINT('',#90042);
#22403=VERTEX_POINT('',#90107);
#22404=VERTEX_POINT('',#90108);
#22405=VERTEX_POINT('',#90132);
#22406=VERTEX_POINT('',#90133);
#22407=VERTEX_POINT('',#90138);
#22408=VERTEX_POINT('',#90139);
#22409=VERTEX_POINT('',#90147);
#22410=VERTEX_POINT('',#90149);
#22411=VERTEX_POINT('',#90182);
#22412=VERTEX_POINT('',#90257);
#22413=VERTEX_POINT('',#90300);
#22414=VERTEX_POINT('',#90304);
#22415=VERTEX_POINT('',#90305);
#22416=VERTEX_POINT('',#90310);
#22417=VERTEX_POINT('',#90311);
#22418=VERTEX_POINT('',#90316);
#22419=VERTEX_POINT('',#90349);
#22420=VERTEX_POINT('',#90424);
#22421=VERTEX_POINT('',#90496);
#22422=VERTEX_POINT('',#90497);
#22423=VERTEX_POINT('',#90502);
#22424=VERTEX_POINT('',#90503);
#22425=VERTEX_POINT('',#90511);
#22426=VERTEX_POINT('',#90513);
#22427=VERTEX_POINT('',#90546);
#22428=VERTEX_POINT('',#90621);
#22429=VERTEX_POINT('',#90664);
#22430=VERTEX_POINT('',#90668);
#22431=VERTEX_POINT('',#90669);
#22432=VERTEX_POINT('',#90674);
#22433=VERTEX_POINT('',#90675);
#22434=VERTEX_POINT('',#90680);
#22435=VERTEX_POINT('',#90713);
#22436=VERTEX_POINT('',#90788);
#22437=VERTEX_POINT('',#90860);
#22438=VERTEX_POINT('',#90861);
#22439=VERTEX_POINT('',#90866);
#22440=VERTEX_POINT('',#90867);
#22441=VERTEX_POINT('',#90875);
#22442=VERTEX_POINT('',#90877);
#22443=VERTEX_POINT('',#90910);
#22444=VERTEX_POINT('',#90985);
#22445=VERTEX_POINT('',#91028);
#22446=VERTEX_POINT('',#91032);
#22447=VERTEX_POINT('',#91033);
#22448=VERTEX_POINT('',#91038);
#22449=VERTEX_POINT('',#91039);
#22450=VERTEX_POINT('',#91044);
#22451=VERTEX_POINT('',#91077);
#22452=VERTEX_POINT('',#91152);
#22453=VERTEX_POINT('',#91230);
#22454=VERTEX_POINT('',#91232);
#22455=VERTEX_POINT('',#91236);
#22456=VERTEX_POINT('',#91248);
#22457=VERTEX_POINT('',#91389);
#22458=VERTEX_POINT('',#91396);
#22459=VERTEX_POINT('',#91417);
#22460=VERTEX_POINT('',#91441);
#22461=VERTEX_POINT('',#91462);
#22462=VERTEX_POINT('',#91471);
#22463=VERTEX_POINT('',#91492);
#22464=VERTEX_POINT('',#91508);
#22465=VERTEX_POINT('',#91553);
#22466=VERTEX_POINT('',#91960);
#22467=VERTEX_POINT('',#91962);
#22468=VERTEX_POINT('',#92091);
#22469=VERTEX_POINT('',#92092);
#22470=VERTEX_POINT('',#92444);
#22471=VERTEX_POINT('',#92445);
#22472=VERTEX_POINT('',#92525);
#22473=VERTEX_POINT('',#92530);
#22474=VERTEX_POINT('',#92534);
#22475=VERTEX_POINT('',#92538);
#22476=VERTEX_POINT('',#92539);
#22477=VERTEX_POINT('',#92585);
#22478=VERTEX_POINT('',#92747);
#22479=VERTEX_POINT('',#92748);
#22480=VERTEX_POINT('',#92873);
#22481=VERTEX_POINT('',#92877);
#22482=VERTEX_POINT('',#92919);
#22483=VERTEX_POINT('',#92995);
#22484=VERTEX_POINT('',#92999);
#22485=VERTEX_POINT('',#93003);
#22486=VERTEX_POINT('',#93007);
#22487=VERTEX_POINT('',#93052);
#22488=VERTEX_POINT('',#93092);
#22489=VERTEX_POINT('',#93107);
#22490=VERTEX_POINT('',#93140);
#22491=VERTEX_POINT('',#93394);
#22492=VERTEX_POINT('',#93748);
#22493=VERTEX_POINT('',#93749);
#22494=VERTEX_POINT('',#93751);
#22495=VERTEX_POINT('',#93966);
#22496=VERTEX_POINT('',#94185);
#22497=VERTEX_POINT('',#94186);
#22498=VERTEX_POINT('',#94369);
#22499=VERTEX_POINT('',#94370);
#22500=VERTEX_POINT('',#94422);
#22501=VERTEX_POINT('',#94423);
#22502=VERTEX_POINT('',#94425);
#22503=VERTEX_POINT('',#94508);
#22504=VERTEX_POINT('',#94667);
#22505=VERTEX_POINT('',#94668);
#22506=VERTEX_POINT('',#94758);
#22507=VERTEX_POINT('',#94759);
#22508=VERTEX_POINT('',#94868);
#22509=VERTEX_POINT('',#94870);
#22510=VERTEX_POINT('',#95221);
#22511=VERTEX_POINT('',#96179);
#22512=VERTEX_POINT('',#96264);
#26867=EDGE_CURVE('',#22215,#22216,#5022,.T.);
#26868=EDGE_CURVE('',#22216,#22217,#18972,.T.);
#26869=EDGE_CURVE('',#22218,#22217,#5023,.T.);
#26870=EDGE_CURVE('',#22215,#22218,#18973,.T.);
#26871=EDGE_CURVE('',#22219,#22220,#5024,.T.);
#26872=EDGE_CURVE('',#22220,#22216,#5025,.T.);
#26873=EDGE_CURVE('',#22219,#22215,#5026,.T.);
#26874=EDGE_CURVE('',#22221,#22222,#5027,.T.);
#26875=EDGE_CURVE('',#22222,#22220,#18974,.T.);
#26876=EDGE_CURVE('',#22221,#22219,#18975,.T.);
#26877=EDGE_CURVE('',#22217,#22222,#5028,.T.);
#26878=EDGE_CURVE('',#22218,#22221,#5029,.T.);
#26879=EDGE_CURVE('',#22223,#22224,#18976,.T.);
#26880=EDGE_CURVE('',#22224,#22225,#5030,.T.);
#26881=EDGE_CURVE('',#22225,#22226,#18977,.T.);
#26882=EDGE_CURVE('',#22226,#22223,#5031,.T.);
#26883=EDGE_CURVE('',#22224,#22227,#5032,.T.);
#26884=EDGE_CURVE('',#22227,#22228,#5033,.T.);
#26885=EDGE_CURVE('',#22225,#22228,#5034,.T.);
#26886=EDGE_CURVE('',#22228,#22229,#18978,.T.);
#26887=EDGE_CURVE('',#22226,#22229,#5035,.T.);
#26888=EDGE_CURVE('',#22229,#22230,#5036,.T.);
#26889=EDGE_CURVE('',#22223,#22230,#5037,.T.);
#26890=EDGE_CURVE('',#22230,#22227,#18979,.T.);
#26891=EDGE_CURVE('',#22231,#22232,#2188,.T.);
#26892=EDGE_CURVE('',#22232,#22233,#5038,.T.);
#26893=EDGE_CURVE('',#22233,#22234,#18980,.T.);
#26894=EDGE_CURVE('',#22234,#22235,#2189,.T.);
#26895=EDGE_CURVE('',#22235,#22236,#5039,.T.);
#26896=EDGE_CURVE('',#22236,#22237,#18981,.T.);
#26897=EDGE_CURVE('',#22237,#22238,#5040,.T.);
#26898=EDGE_CURVE('',#22238,#22239,#2190,.T.);
#26899=EDGE_CURVE('',#22239,#22240,#18982,.T.);
#26900=EDGE_CURVE('',#22240,#22241,#5041,.T.);
#26901=EDGE_CURVE('',#22241,#22242,#2191,.T.);
#26902=EDGE_CURVE('',#22242,#22243,#18983,.T.);
#26903=EDGE_CURVE('',#22243,#22244,#5042,.T.);
#26904=EDGE_CURVE('',#22244,#22244,#18984,.T.);
#26905=EDGE_CURVE('',#22243,#22245,#2192,.T.);
#26906=EDGE_CURVE('',#22245,#22246,#2193,.T.);
#26907=EDGE_CURVE('',#22246,#22247,#2194,.T.);
#26908=EDGE_CURVE('',#22247,#22248,#2195,.T.);
#26909=EDGE_CURVE('',#22248,#22249,#2196,.T.);
#26910=EDGE_CURVE('',#22249,#22231,#18985,.T.);
#26911=EDGE_CURVE('',#22244,#22250,#18986,.T.);
#26912=EDGE_CURVE('',#22250,#22250,#18987,.T.);
#26913=EDGE_CURVE('',#22251,#22252,#18988,.T.);
#26914=EDGE_CURVE('',#22252,#22253,#5043,.T.);
#26915=EDGE_CURVE('',#22253,#22254,#2197,.T.);
#26916=EDGE_CURVE('',#22255,#22254,#18989,.T.);
#26917=EDGE_CURVE('',#22255,#22256,#2198,.T.);
#26918=EDGE_CURVE('',#22256,#22251,#5044,.T.);
#26919=EDGE_CURVE('',#22257,#22258,#18990,.T.);
#26920=EDGE_CURVE('',#22258,#22259,#5045,.T.);
#26921=EDGE_CURVE('',#22259,#22260,#2199,.T.);
#26922=EDGE_CURVE('',#22261,#22260,#18991,.T.);
#26923=EDGE_CURVE('',#22261,#22262,#2200,.T.);
#26924=EDGE_CURVE('',#22262,#22257,#5046,.T.);
#26925=EDGE_CURVE('',#22263,#22264,#18992,.T.);
#26926=EDGE_CURVE('',#22264,#22265,#5047,.T.);
#26927=EDGE_CURVE('',#22265,#22266,#2201,.T.);
#26928=EDGE_CURVE('',#22267,#22266,#18993,.T.);
#26929=EDGE_CURVE('',#22267,#22268,#2202,.T.);
#26930=EDGE_CURVE('',#22268,#22263,#5048,.T.);
#26931=EDGE_CURVE('',#22269,#22270,#18994,.T.);
#26932=EDGE_CURVE('',#22270,#22271,#5049,.T.);
#26933=EDGE_CURVE('',#22271,#22272,#18995,.T.);
#26934=EDGE_CURVE('',#22272,#22273,#5050,.T.);
#26935=EDGE_CURVE('',#22274,#22273,#2203,.T.);
#26936=EDGE_CURVE('',#22274,#22275,#18996,.T.);
#26937=EDGE_CURVE('',#22276,#22275,#2204,.T.);
#26938=EDGE_CURVE('',#22276,#22277,#5051,.T.);
#26939=EDGE_CURVE('',#22277,#22271,#18997,.T.);
#26940=EDGE_CURVE('',#22270,#22269,#18998,.T.);
#26941=EDGE_CURVE('',#22278,#22279,#18999,.T.);
#26942=EDGE_CURVE('',#22279,#22280,#5052,.T.);
#26943=EDGE_CURVE('',#22280,#22281,#19000,.T.);
#26944=EDGE_CURVE('',#22278,#22281,#5053,.T.);
#26945=EDGE_CURVE('',#22282,#22278,#19001,.T.);
#26946=EDGE_CURVE('',#22283,#22282,#19002,.T.);
#26947=EDGE_CURVE('',#22279,#22283,#19003,.T.);
#26948=EDGE_CURVE('',#22284,#22277,#2205,.T.);
#26949=EDGE_CURVE('',#22285,#22284,#19004,.T.);
#26950=EDGE_CURVE('',#22272,#22285,#2206,.T.);
#26951=EDGE_CURVE('',#22280,#22286,#19005,.T.);
#26952=EDGE_CURVE('',#22287,#22286,#19006,.T.);
#26953=EDGE_CURVE('',#22281,#22287,#19007,.T.);
#26954=EDGE_CURVE('',#22269,#22288,#19008,.T.);
#26955=EDGE_CURVE('',#22288,#22288,#19009,.T.);
#26956=EDGE_CURVE('',#22289,#22290,#19010,.T.);
#26957=EDGE_CURVE('',#22290,#22291,#5054,.T.);
#26958=EDGE_CURVE('',#22291,#22292,#19011,.T.);
#26959=EDGE_CURVE('',#22292,#22293,#5055,.T.);
#26960=EDGE_CURVE('',#22294,#22293,#2207,.T.);
#26961=EDGE_CURVE('',#22294,#22295,#19012,.T.);
#26962=EDGE_CURVE('',#22296,#22295,#2208,.T.);
#26963=EDGE_CURVE('',#22296,#22297,#5056,.T.);
#26964=EDGE_CURVE('',#22297,#22291,#19013,.T.);
#26965=EDGE_CURVE('',#22290,#22289,#19014,.T.);
#26966=EDGE_CURVE('',#22298,#22299,#19015,.T.);
#26967=EDGE_CURVE('',#22299,#22300,#5057,.T.);
#26968=EDGE_CURVE('',#22300,#22301,#19016,.T.);
#26969=EDGE_CURVE('',#22298,#22301,#5058,.T.);
#26970=EDGE_CURVE('',#22302,#22298,#19017,.T.);
#26971=EDGE_CURVE('',#22303,#22302,#19018,.T.);
#26972=EDGE_CURVE('',#22299,#22303,#19019,.T.);
#26973=EDGE_CURVE('',#22304,#22297,#2209,.T.);
#26974=EDGE_CURVE('',#22305,#22304,#19020,.T.);
#26975=EDGE_CURVE('',#22292,#22305,#2210,.T.);
#26976=EDGE_CURVE('',#22300,#22306,#19021,.T.);
#26977=EDGE_CURVE('',#22307,#22306,#19022,.T.);
#26978=EDGE_CURVE('',#22301,#22307,#19023,.T.);
#26979=EDGE_CURVE('',#22289,#22308,#19024,.T.);
#26980=EDGE_CURVE('',#22308,#22308,#19025,.T.);
#26981=EDGE_CURVE('',#22309,#22310,#19026,.T.);
#26982=EDGE_CURVE('',#22310,#22311,#5059,.T.);
#26983=EDGE_CURVE('',#22311,#22312,#19027,.T.);
#26984=EDGE_CURVE('',#22312,#22313,#5060,.T.);
#26985=EDGE_CURVE('',#22314,#22313,#2211,.T.);
#26986=EDGE_CURVE('',#22314,#22315,#19028,.T.);
#26987=EDGE_CURVE('',#22316,#22315,#2212,.T.);
#26988=EDGE_CURVE('',#22316,#22317,#5061,.T.);
#26989=EDGE_CURVE('',#22317,#22311,#19029,.T.);
#26990=EDGE_CURVE('',#22310,#22309,#19030,.T.);
#26991=EDGE_CURVE('',#22318,#22319,#19031,.T.);
#26992=EDGE_CURVE('',#22319,#22320,#5062,.T.);
#26993=EDGE_CURVE('',#22320,#22321,#19032,.T.);
#26994=EDGE_CURVE('',#22318,#22321,#5063,.T.);
#26995=EDGE_CURVE('',#22322,#22318,#19033,.T.);
#26996=EDGE_CURVE('',#22323,#22322,#19034,.T.);
#26997=EDGE_CURVE('',#22319,#22323,#19035,.T.);
#26998=EDGE_CURVE('',#22324,#22317,#2213,.T.);
#26999=EDGE_CURVE('',#22325,#22324,#19036,.T.);
#27000=EDGE_CURVE('',#22312,#22325,#2214,.T.);
#27001=EDGE_CURVE('',#22320,#22326,#19037,.T.);
#27002=EDGE_CURVE('',#22327,#22326,#19038,.T.);
#27003=EDGE_CURVE('',#22321,#22327,#19039,.T.);
#27004=EDGE_CURVE('',#22309,#22328,#19040,.T.);
#27005=EDGE_CURVE('',#22328,#22328,#19041,.T.);
#27006=EDGE_CURVE('',#22329,#22329,#19042,.T.);
#27007=EDGE_CURVE('',#22329,#22330,#5064,.T.);
#27008=EDGE_CURVE('',#22330,#22331,#19043,.T.);
#27009=EDGE_CURVE('',#22331,#22332,#5065,.T.);
#27010=EDGE_CURVE('',#22333,#22332,#2215,.T.);
#27011=EDGE_CURVE('',#22333,#22334,#19044,.T.);
#27012=EDGE_CURVE('',#22335,#22334,#2216,.T.);
#27013=EDGE_CURVE('',#22335,#22336,#5066,.T.);
#27014=EDGE_CURVE('',#22336,#22330,#19045,.T.);
#27015=EDGE_CURVE('',#22336,#22337,#2217,.T.);
#27016=EDGE_CURVE('',#22338,#22337,#19046,.T.);
#27017=EDGE_CURVE('',#22331,#22338,#2218,.T.);
#27018=EDGE_CURVE('',#22339,#22340,#19047,.T.);
#27019=EDGE_CURVE('',#22340,#22341,#2219,.T.);
#27020=EDGE_CURVE('',#22341,#22342,#2220,.T.);
#27021=EDGE_CURVE('',#22342,#22343,#19048,.T.);
#27022=EDGE_CURVE('',#22343,#22344,#5067,.T.);
#27023=EDGE_CURVE('',#22344,#22345,#5068,.T.);
#27024=EDGE_CURVE('',#22345,#22339,#5069,.T.);
#27025=EDGE_CURVE('',#22346,#22347,#5070,.T.);
#27026=EDGE_CURVE('',#22346,#22348,#19049,.T.);
#27027=EDGE_CURVE('',#22349,#22348,#5071,.T.);
#27028=EDGE_CURVE('',#22349,#22347,#19050,.T.);
#27029=EDGE_CURVE('',#22350,#22351,#5072,.T.);
#27030=EDGE_CURVE('',#22351,#22346,#2221,.T.);
#27031=EDGE_CURVE('',#22347,#22350,#2222,.T.);
#27032=EDGE_CURVE('',#22352,#22353,#5073,.T.);
#27033=EDGE_CURVE('',#22352,#22354,#19051,.T.);
#27034=EDGE_CURVE('',#22355,#22354,#5074,.T.);
#27035=EDGE_CURVE('',#22355,#22353,#19052,.T.);
#27036=EDGE_CURVE('',#22354,#22351,#2223,.T.);
#27037=EDGE_CURVE('',#22350,#22355,#2224,.T.);
#27038=EDGE_CURVE('',#22356,#22357,#5075,.T.);
#27039=EDGE_CURVE('',#22357,#22358,#5076,.T.);
#27040=EDGE_CURVE('',#22358,#22359,#5077,.T.);
#27041=EDGE_CURVE('',#22359,#22356,#5078,.T.);
#27042=EDGE_CURVE('',#22348,#22360,#5079,.T.);
#27043=EDGE_CURVE('',#22360,#22361,#5080,.T.);
#27044=EDGE_CURVE('',#22361,#22349,#5081,.T.);
#27045=EDGE_CURVE('',#22362,#22363,#5082,.T.);
#27046=EDGE_CURVE('',#22363,#22352,#5083,.T.);
#27047=EDGE_CURVE('',#22353,#22362,#5084,.T.);
#27048=EDGE_CURVE('',#22364,#22365,#2225,.T.);
#27049=EDGE_CURVE('',#22366,#22364,#2226,.T.);
#27050=EDGE_CURVE('',#22367,#22366,#2227,.T.);
#27051=EDGE_CURVE('',#22368,#22367,#2228,.T.);
#27052=EDGE_CURVE('',#22369,#22368,#2229,.T.);
#27053=EDGE_CURVE('',#22355,#22369,#19053,.T.);
#27054=EDGE_CURVE('',#22365,#22350,#19054,.T.);
#27055=EDGE_CURVE('',#22365,#22370,#2230,.T.);
#27056=EDGE_CURVE('',#22370,#22347,#19055,.T.);
#27057=EDGE_CURVE('',#22371,#22369,#19056,.T.);
#27058=EDGE_CURVE('',#22353,#22371,#19057,.T.);
#27059=EDGE_CURVE('',#22370,#22372,#19058,.T.);
#27060=EDGE_CURVE('',#22372,#22349,#19059,.T.);
#27061=EDGE_CURVE('',#22373,#22374,#2231,.T.);
#27062=EDGE_CURVE('',#22362,#22373,#19060,.T.);
#27063=EDGE_CURVE('',#22374,#22371,#5085,.T.);
#27064=EDGE_CURVE('',#22372,#22375,#5086,.T.);
#27065=EDGE_CURVE('',#22376,#22361,#19061,.T.);
#27066=EDGE_CURVE('',#22375,#22376,#2232,.T.);
#27067=EDGE_CURVE('',#22377,#22378,#2233,.T.);
#27068=EDGE_CURVE('',#22357,#22377,#19062,.T.);
#27069=EDGE_CURVE('',#22379,#22356,#19063,.T.);
#27070=EDGE_CURVE('',#22380,#22379,#2234,.T.);
#27071=EDGE_CURVE('',#22378,#22380,#5087,.T.);
#27072=EDGE_CURVE('',#22379,#22373,#2235,.T.);
#27073=EDGE_CURVE('',#22362,#22356,#19064,.T.);
#27074=EDGE_CURVE('',#22376,#22377,#2236,.T.);
#27075=EDGE_CURVE('',#22357,#22361,#19065,.T.);
#27076=EDGE_CURVE('',#22363,#22359,#19066,.T.);
#27077=EDGE_CURVE('',#22358,#22360,#19067,.T.);
#27078=EDGE_CURVE('',#22359,#22344,#19068,.T.);
#27079=EDGE_CURVE('',#22345,#22358,#19069,.T.);
#27080=EDGE_CURVE('',#22363,#22344,#19070,.T.);
#27081=EDGE_CURVE('',#22345,#22360,#19071,.T.);
#27082=EDGE_CURVE('',#22352,#22343,#19072,.T.);
#27083=EDGE_CURVE('',#22339,#22348,#19073,.T.);
#27084=EDGE_CURVE('',#22354,#22342,#19074,.T.);
#27085=EDGE_CURVE('',#22340,#22346,#19075,.T.);
#27086=EDGE_CURVE('',#22351,#22341,#19076,.T.);
#27087=EDGE_CURVE('',#22381,#22382,#19077,.T.);
#27088=EDGE_CURVE('',#22383,#22382,#19078,.T.);
#27089=EDGE_CURVE('',#22383,#22384,#19079,.T.);
#27090=EDGE_CURVE('',#22381,#22384,#19080,.T.);
#27091=EDGE_CURVE('',#22385,#22386,#19081,.T.);
#27092=EDGE_CURVE('',#22384,#22386,#5088,.T.);
#27093=EDGE_CURVE('',#22385,#22383,#5089,.T.);
#27094=EDGE_CURVE('',#22387,#22388,#19082,.T.);
#27095=EDGE_CURVE('',#22382,#22388,#5090,.T.);
#27096=EDGE_CURVE('',#22387,#22381,#5091,.T.);
#27097=EDGE_CURVE('',#22388,#22385,#19083,.T.);
#27098=EDGE_CURVE('',#22386,#22387,#19084,.T.);
#27099=EDGE_CURVE('',#22331,#22389,#19085,.T.);
#27100=EDGE_CURVE('',#22390,#22389,#5092,.T.);
#27101=EDGE_CURVE('',#22390,#22332,#19086,.T.);
#27102=EDGE_CURVE('',#22391,#22333,#19087,.T.);
#27103=EDGE_CURVE('',#22390,#22391,#2237,.T.);
#27104=EDGE_CURVE('',#22338,#22392,#19088,.T.);
#27105=EDGE_CURVE('',#22392,#22389,#2238,.T.);
#27106=EDGE_CURVE('',#22393,#22394,#19089,.T.);
#27107=EDGE_CURVE('',#22391,#22394,#5093,.T.);
#27108=EDGE_CURVE('',#22393,#22390,#5094,.T.);
#27109=EDGE_CURVE('',#22395,#22334,#19090,.T.);
#27110=EDGE_CURVE('',#22395,#22391,#19091,.T.);
#27111=EDGE_CURVE('',#22396,#22397,#19092,.T.);
#27112=EDGE_CURVE('',#22392,#22397,#5095,.T.);
#27113=EDGE_CURVE('',#22396,#22338,#5096,.T.);
#27114=EDGE_CURVE('',#22398,#22399,#19093,.T.);
#27115=EDGE_CURVE('',#22394,#22399,#19094,.T.);
#27116=EDGE_CURVE('',#22398,#22393,#19095,.T.);
#27117=EDGE_CURVE('',#22400,#22335,#19096,.T.);
#27118=EDGE_CURVE('',#22395,#22400,#2239,.T.);
#27119=EDGE_CURVE('',#22401,#22402,#2240,.T.);
#27120=EDGE_CURVE('',#22402,#22337,#19097,.T.);
#27121=EDGE_CURVE('',#22336,#22401,#19098,.T.);
#27122=EDGE_CURVE('',#22403,#22404,#19099,.T.);
#27123=EDGE_CURVE('',#22397,#22404,#19100,.T.);
#27124=EDGE_CURVE('',#22403,#22396,#19101,.T.);
#27125=EDGE_CURVE('',#22400,#22398,#5097,.T.);
#27126=EDGE_CURVE('',#22399,#22395,#5098,.T.);
#27127=EDGE_CURVE('',#22401,#22400,#5099,.T.);
#27128=EDGE_CURVE('',#22404,#22402,#5100,.T.);
#27129=EDGE_CURVE('',#22337,#22403,#5101,.T.);
#27130=EDGE_CURVE('',#22393,#22388,#5102,.T.);
#27131=EDGE_CURVE('',#22398,#22385,#5103,.T.);
#27132=EDGE_CURVE('',#22404,#22383,#5104,.T.);
#27133=EDGE_CURVE('',#22397,#22382,#5105,.T.);
#27134=EDGE_CURVE('',#22405,#22406,#19102,.T.);
#27135=EDGE_CURVE('',#22321,#22406,#5106,.T.);
#27136=EDGE_CURVE('',#22405,#22327,#5107,.T.);
#27137=EDGE_CURVE('',#22407,#22408,#19103,.T.);
#27138=EDGE_CURVE('',#22406,#22408,#19104,.T.);
#27139=EDGE_CURVE('',#22407,#22405,#19105,.T.);
#27140=EDGE_CURVE('',#22408,#22320,#5108,.T.);
#27141=EDGE_CURVE('',#22326,#22407,#5109,.T.);
#27142=EDGE_CURVE('',#22409,#22315,#19106,.T.);
#27143=EDGE_CURVE('',#22314,#22410,#19107,.T.);
#27144=EDGE_CURVE('',#22409,#22410,#19108,.T.);
#27145=EDGE_CURVE('',#22313,#22411,#19109,.T.);
#27146=EDGE_CURVE('',#22411,#22410,#2241,.T.);
#27147=EDGE_CURVE('',#22412,#22316,#19110,.T.);
#27148=EDGE_CURVE('',#22409,#22412,#2242,.T.);
#27149=EDGE_CURVE('',#22312,#22413,#19111,.T.);
#27150=EDGE_CURVE('',#22411,#22413,#5110,.T.);
#27151=EDGE_CURVE('',#22414,#22415,#19112,.T.);
#27152=EDGE_CURVE('',#22410,#22415,#5111,.T.);
#27153=EDGE_CURVE('',#22414,#22411,#5112,.T.);
#27154=EDGE_CURVE('',#22416,#22417,#19113,.T.);
#27155=EDGE_CURVE('',#22412,#22417,#5113,.T.);
#27156=EDGE_CURVE('',#22416,#22409,#5114,.T.);
#27157=EDGE_CURVE('',#22418,#22317,#19114,.T.);
#27158=EDGE_CURVE('',#22418,#22412,#5115,.T.);
#27159=EDGE_CURVE('',#22325,#22419,#19115,.T.);
#27160=EDGE_CURVE('',#22419,#22413,#2243,.T.);
#27161=EDGE_CURVE('',#22417,#22414,#19116,.T.);
#27162=EDGE_CURVE('',#22415,#22416,#19117,.T.);
#27163=EDGE_CURVE('',#22420,#22324,#19118,.T.);
#27164=EDGE_CURVE('',#22418,#22420,#2244,.T.);
#27165=EDGE_CURVE('',#22419,#22318,#5116,.T.);
#27166=EDGE_CURVE('',#22322,#22325,#5117,.T.);
#27167=EDGE_CURVE('',#22324,#22323,#5118,.T.);
#27168=EDGE_CURVE('',#22319,#22420,#5119,.T.);
#27169=EDGE_CURVE('',#22417,#22408,#5120,.T.);
#27170=EDGE_CURVE('',#22414,#22406,#5121,.T.);
#27171=EDGE_CURVE('',#22421,#22422,#19119,.T.);
#27172=EDGE_CURVE('',#22301,#22422,#5122,.T.);
#27173=EDGE_CURVE('',#22421,#22307,#5123,.T.);
#27174=EDGE_CURVE('',#22423,#22424,#19120,.T.);
#27175=EDGE_CURVE('',#22422,#22424,#19121,.T.);
#27176=EDGE_CURVE('',#22423,#22421,#19122,.T.);
#27177=EDGE_CURVE('',#22424,#22300,#5124,.T.);
#27178=EDGE_CURVE('',#22306,#22423,#5125,.T.);
#27179=EDGE_CURVE('',#22425,#22295,#19123,.T.);
#27180=EDGE_CURVE('',#22294,#22426,#19124,.T.);
#27181=EDGE_CURVE('',#22425,#22426,#19125,.T.);
#27182=EDGE_CURVE('',#22293,#22427,#19126,.T.);
#27183=EDGE_CURVE('',#22427,#22426,#2245,.T.);
#27184=EDGE_CURVE('',#22428,#22296,#19127,.T.);
#27185=EDGE_CURVE('',#22425,#22428,#2246,.T.);
#27186=EDGE_CURVE('',#22292,#22429,#19128,.T.);
#27187=EDGE_CURVE('',#22427,#22429,#5126,.T.);
#27188=EDGE_CURVE('',#22430,#22431,#19129,.T.);
#27189=EDGE_CURVE('',#22426,#22431,#5127,.T.);
#27190=EDGE_CURVE('',#22430,#22427,#5128,.T.);
#27191=EDGE_CURVE('',#22432,#22433,#19130,.T.);
#27192=EDGE_CURVE('',#22428,#22433,#5129,.T.);
#27193=EDGE_CURVE('',#22432,#22425,#5130,.T.);
#27194=EDGE_CURVE('',#22434,#22297,#19131,.T.);
#27195=EDGE_CURVE('',#22434,#22428,#5131,.T.);
#27196=EDGE_CURVE('',#22305,#22435,#19132,.T.);
#27197=EDGE_CURVE('',#22435,#22429,#2247,.T.);
#27198=EDGE_CURVE('',#22433,#22430,#19133,.T.);
#27199=EDGE_CURVE('',#22431,#22432,#19134,.T.);
#27200=EDGE_CURVE('',#22436,#22304,#19135,.T.);
#27201=EDGE_CURVE('',#22434,#22436,#2248,.T.);
#27202=EDGE_CURVE('',#22435,#22298,#5132,.T.);
#27203=EDGE_CURVE('',#22302,#22305,#5133,.T.);
#27204=EDGE_CURVE('',#22304,#22303,#5134,.T.);
#27205=EDGE_CURVE('',#22299,#22436,#5135,.T.);
#27206=EDGE_CURVE('',#22433,#22424,#5136,.T.);
#27207=EDGE_CURVE('',#22430,#22422,#5137,.T.);
#27208=EDGE_CURVE('',#22437,#22438,#19136,.T.);
#27209=EDGE_CURVE('',#22281,#22438,#5138,.T.);
#27210=EDGE_CURVE('',#22437,#22287,#5139,.T.);
#27211=EDGE_CURVE('',#22439,#22440,#19137,.T.);
#27212=EDGE_CURVE('',#22438,#22440,#19138,.T.);
#27213=EDGE_CURVE('',#22439,#22437,#19139,.T.);
#27214=EDGE_CURVE('',#22440,#22280,#5140,.T.);
#27215=EDGE_CURVE('',#22286,#22439,#5141,.T.);
#27216=EDGE_CURVE('',#22441,#22275,#19140,.T.);
#27217=EDGE_CURVE('',#22274,#22442,#19141,.T.);
#27218=EDGE_CURVE('',#22441,#22442,#19142,.T.);
#27219=EDGE_CURVE('',#22273,#22443,#19143,.T.);
#27220=EDGE_CURVE('',#22443,#22442,#2249,.T.);
#27221=EDGE_CURVE('',#22444,#22276,#19144,.T.);
#27222=EDGE_CURVE('',#22441,#22444,#2250,.T.);
#27223=EDGE_CURVE('',#22272,#22445,#19145,.T.);
#27224=EDGE_CURVE('',#22443,#22445,#5142,.T.);
#27225=EDGE_CURVE('',#22446,#22447,#19146,.T.);
#27226=EDGE_CURVE('',#22442,#22447,#5143,.T.);
#27227=EDGE_CURVE('',#22446,#22443,#5144,.T.);
#27228=EDGE_CURVE('',#22448,#22449,#19147,.T.);
#27229=EDGE_CURVE('',#22444,#22449,#5145,.T.);
#27230=EDGE_CURVE('',#22448,#22441,#5146,.T.);
#27231=EDGE_CURVE('',#22450,#22277,#19148,.T.);
#27232=EDGE_CURVE('',#22450,#22444,#5147,.T.);
#27233=EDGE_CURVE('',#22285,#22451,#19149,.T.);
#27234=EDGE_CURVE('',#22451,#22445,#2251,.T.);
#27235=EDGE_CURVE('',#22449,#22446,#19150,.T.);
#27236=EDGE_CURVE('',#22447,#22448,#19151,.T.);
#27237=EDGE_CURVE('',#22452,#22284,#19152,.T.);
#27238=EDGE_CURVE('',#22450,#22452,#2252,.T.);
#27239=EDGE_CURVE('',#22451,#22278,#5148,.T.);
#27240=EDGE_CURVE('',#22282,#22285,#5149,.T.);
#27241=EDGE_CURVE('',#22284,#22283,#5150,.T.);
#27242=EDGE_CURVE('',#22279,#22452,#5151,.T.);
#27243=EDGE_CURVE('',#22449,#22440,#5152,.T.);
#27244=EDGE_CURVE('',#22446,#22438,#5153,.T.);
#27245=EDGE_CURVE('',#22264,#22263,#5154,.T.);
#27246=EDGE_CURVE('',#22258,#22257,#5155,.T.);
#27247=EDGE_CURVE('',#22252,#22251,#5156,.T.);
#27248=EDGE_CURVE('',#22453,#22374,#19153,.T.);
#27249=EDGE_CURVE('',#22371,#22454,#19154,.T.);
#27250=EDGE_CURVE('',#22453,#22454,#5157,.T.);
#27251=EDGE_CURVE('',#22369,#22455,#19155,.T.);
#27252=EDGE_CURVE('',#22454,#22455,#19156,.T.);
#27253=EDGE_CURVE('',#22456,#22453,#19157,.T.);
#27254=EDGE_CURVE('',#22456,#22380,#19158,.T.);
#27255=EDGE_CURVE('',#22368,#22457,#19159,.T.);
#27256=EDGE_CURVE('',#22455,#22457,#2253,.T.);
#27257=EDGE_CURVE('',#22458,#22378,#19160,.T.);
#27258=EDGE_CURVE('',#22458,#22456,#5158,.T.);
#27259=EDGE_CURVE('',#22367,#22459,#19161,.T.);
#27260=EDGE_CURVE('',#22457,#22459,#2254,.T.);
#27261=EDGE_CURVE('',#22460,#22375,#19162,.T.);
#27262=EDGE_CURVE('',#22460,#22458,#19163,.T.);
#27263=EDGE_CURVE('',#22366,#22461,#19164,.T.);
#27264=EDGE_CURVE('',#22459,#22461,#2255,.T.);
#27265=EDGE_CURVE('',#22462,#22372,#19165,.T.);
#27266=EDGE_CURVE('',#22462,#22460,#5159,.T.);
#27267=EDGE_CURVE('',#22364,#22463,#19166,.T.);
#27268=EDGE_CURVE('',#22461,#22463,#2256,.T.);
#27269=EDGE_CURVE('',#22464,#22370,#19167,.T.);
#27270=EDGE_CURVE('',#22464,#22462,#19168,.T.);
#27271=EDGE_CURVE('',#22365,#22465,#19169,.T.);
#27272=EDGE_CURVE('',#22463,#22465,#2257,.T.);
#27273=EDGE_CURVE('',#22465,#22464,#2258,.T.);
#27274=EDGE_CURVE('',#22460,#22466,#5160,.T.);
#27275=EDGE_CURVE('',#22467,#22458,#5161,.T.);
#27276=EDGE_CURVE('',#22467,#22466,#19170,.T.);
#27277=EDGE_CURVE('',#22468,#22469,#19171,.T.);
#27278=EDGE_CURVE('',#22466,#22469,#2259,.T.);
#27279=EDGE_CURVE('',#22468,#22467,#2260,.T.);
#27280=EDGE_CURVE('',#22470,#22471,#19172,.T.);
#27281=EDGE_CURVE('',#22469,#22471,#2261,.T.);
#27282=EDGE_CURVE('',#22470,#22468,#2262,.T.);
#27283=EDGE_CURVE('',#22472,#22236,#19173,.T.);
#27284=EDGE_CURVE('',#22236,#22471,#19174,.T.);
#27285=EDGE_CURVE('',#22470,#22472,#19175,.T.);
#27286=EDGE_CURVE('',#22473,#22237,#19176,.T.);
#27287=EDGE_CURVE('',#22473,#22472,#19177,.T.);
#27288=EDGE_CURVE('',#22235,#22474,#19178,.T.);
#27289=EDGE_CURVE('',#22471,#22474,#5162,.T.);
#27290=EDGE_CURVE('',#22475,#22476,#19179,.T.);
#27291=EDGE_CURVE('',#22476,#22237,#19180,.T.);
#27292=EDGE_CURVE('',#22473,#22475,#19181,.T.);
#27293=EDGE_CURVE('',#22234,#22477,#19182,.T.);
#27294=EDGE_CURVE('',#22474,#22477,#2263,.T.);
#27295=EDGE_CURVE('',#22478,#22479,#19183,.T.);
#27296=EDGE_CURVE('',#22476,#22479,#2264,.T.);
#27297=EDGE_CURVE('',#22478,#22475,#2265,.T.);
#27298=EDGE_CURVE('',#22480,#22238,#19184,.T.);
#27299=EDGE_CURVE('',#22480,#22476,#5163,.T.);
#27300=EDGE_CURVE('',#22233,#22481,#19185,.T.);
#27301=EDGE_CURVE('',#22477,#22481,#19186,.T.);
#27302=EDGE_CURVE('',#22456,#22478,#5164,.T.);
#27303=EDGE_CURVE('',#22479,#22453,#5165,.T.);
#27304=EDGE_CURVE('',#22482,#22239,#19187,.T.);
#27305=EDGE_CURVE('',#22482,#22480,#2266,.T.);
#27306=EDGE_CURVE('',#22233,#22483,#19188,.T.);
#27307=EDGE_CURVE('',#22481,#22483,#19189,.T.);
#27308=EDGE_CURVE('',#22484,#22240,#19190,.T.);
#27309=EDGE_CURVE('',#22484,#22482,#19191,.T.);
#27310=EDGE_CURVE('',#22232,#22485,#19192,.T.);
#27311=EDGE_CURVE('',#22483,#22485,#5166,.T.);
#27312=EDGE_CURVE('',#22486,#22484,#19193,.T.);
#27313=EDGE_CURVE('',#22486,#22240,#19194,.T.);
#27314=EDGE_CURVE('',#22249,#22487,#19195,.T.);
#27315=EDGE_CURVE('',#22485,#22487,#2267,.T.);
#27316=EDGE_CURVE('',#22488,#22241,#19196,.T.);
#27317=EDGE_CURVE('',#22488,#22486,#5167,.T.);
#27318=EDGE_CURVE('',#22248,#22489,#19197,.T.);
#27319=EDGE_CURVE('',#22487,#22489,#2268,.T.);
#27320=EDGE_CURVE('',#22490,#22242,#19198,.T.);
#27321=EDGE_CURVE('',#22490,#22488,#2269,.T.);
#27322=EDGE_CURVE('',#22247,#22461,#19199,.T.);
#27323=EDGE_CURVE('',#22489,#22463,#2270,.T.);
#27324=EDGE_CURVE('',#22491,#22245,#19200,.T.);
#27325=EDGE_CURVE('',#22491,#22490,#2271,.T.);
#27326=EDGE_CURVE('',#22246,#22459,#19201,.T.);
#27327=EDGE_CURVE('',#22457,#22491,#2272,.T.);
#27328=EDGE_CURVE('',#22492,#22493,#19202,.T.);
#27329=EDGE_CURVE('',#22494,#22493,#2273,.T.);
#27330=EDGE_CURVE('',#22494,#22495,#19203,.T.);
#27331=EDGE_CURVE('',#22492,#22495,#2274,.T.);
#27332=EDGE_CURVE('',#22496,#22497,#19204,.T.);
#27333=EDGE_CURVE('',#22497,#22495,#2275,.T.);
#27334=EDGE_CURVE('',#22494,#22496,#2276,.T.);
#27335=EDGE_CURVE('',#22485,#22492,#2277,.T.);
#27336=EDGE_CURVE('',#22493,#22487,#2278,.T.);
#27337=EDGE_CURVE('',#22498,#22499,#19205,.T.);
#27338=EDGE_CURVE('',#22497,#22499,#19206,.T.);
#27339=EDGE_CURVE('',#22498,#22496,#19207,.T.);
#27340=EDGE_CURVE('',#22500,#22501,#19208,.T.);
#27341=EDGE_CURVE('',#22502,#22500,#2279,.T.);
#27342=EDGE_CURVE('',#22502,#22503,#19209,.T.);
#27343=EDGE_CURVE('',#22503,#22501,#2280,.T.);
#27344=EDGE_CURVE('',#22504,#22505,#19210,.T.);
#27345=EDGE_CURVE('',#22499,#22505,#2281,.T.);
#27346=EDGE_CURVE('',#22504,#22498,#2282,.T.);
#27347=EDGE_CURVE('',#22506,#22507,#19211,.T.);
#27348=EDGE_CURVE('',#22503,#22507,#19212,.T.);
#27349=EDGE_CURVE('',#22506,#22502,#19213,.T.);
#27350=EDGE_CURVE('',#22482,#22506,#2283,.T.);
#27351=EDGE_CURVE('',#22507,#22480,#2284,.T.);
#27352=EDGE_CURVE('',#22254,#22267,#5168,.T.);
#27353=EDGE_CURVE('',#22266,#22497,#5169,.T.);
#27354=EDGE_CURVE('',#22505,#22477,#2285,.T.);
#27355=EDGE_CURVE('',#22481,#22261,#5170,.T.);
#27356=EDGE_CURVE('',#22260,#22255,#5171,.T.);
#27357=EDGE_CURVE('',#22464,#22508,#5172,.T.);
#27358=EDGE_CURVE('',#22509,#22462,#5173,.T.);
#27359=EDGE_CURVE('',#22509,#22508,#19214,.T.);
#27360=EDGE_CURVE('',#22493,#22510,#19215,.T.);
#27361=EDGE_CURVE('',#22508,#22510,#2286,.T.);
#27362=EDGE_CURVE('',#22498,#22509,#2287,.T.);
#27363=EDGE_CURVE('',#22491,#22511,#2288,.T.);
#27364=EDGE_CURVE('',#22490,#22501,#2289,.T.);
#27365=EDGE_CURVE('',#22512,#22507,#2290,.T.);
#27366=EDGE_CURVE('',#22512,#22511,#19216,.T.);
#27367=EDGE_CURVE('',#22454,#22512,#5174,.T.);
#27368=EDGE_CURVE('',#22511,#22455,#5175,.T.);
#27369=EDGE_CURVE('',#22510,#22465,#5176,.T.);
#27370=EDGE_CURVE('',#22509,#22466,#5177,.T.);
#27371=EDGE_CURVE('',#22512,#22479,#5178,.T.);
#27372=EDGE_CURVE('',#22504,#22469,#5179,.T.);
#27373=EDGE_CURVE('',#22500,#22488,#2291,.T.);
#27374=EDGE_CURVE('',#22486,#22500,#5180,.T.);
#27375=EDGE_CURVE('',#22502,#22484,#5181,.T.);
#27376=EDGE_CURVE('',#22474,#22504,#2292,.T.);
#27377=EDGE_CURVE('',#22510,#22489,#2293,.T.);
#27378=EDGE_CURVE('',#22256,#22259,#5182,.T.);
#27379=EDGE_CURVE('',#22262,#22483,#5183,.T.);
#27380=EDGE_CURVE('',#22495,#22265,#5184,.T.);
#27381=EDGE_CURVE('',#22268,#22253,#5185,.T.);
#35046=ORIENTED_EDGE('',*,*,#26867,.T.);
#35047=ORIENTED_EDGE('',*,*,#26868,.T.);
#35048=ORIENTED_EDGE('',*,*,#26869,.F.);
#35049=ORIENTED_EDGE('',*,*,#26870,.F.);
#35050=ORIENTED_EDGE('',*,*,#26871,.T.);
#35051=ORIENTED_EDGE('',*,*,#26872,.T.);
#35052=ORIENTED_EDGE('',*,*,#26867,.F.);
#35053=ORIENTED_EDGE('',*,*,#26873,.F.);
#35054=ORIENTED_EDGE('',*,*,#26874,.T.);
#35055=ORIENTED_EDGE('',*,*,#26875,.T.);
#35056=ORIENTED_EDGE('',*,*,#26871,.F.);
#35057=ORIENTED_EDGE('',*,*,#26876,.F.);
#35058=ORIENTED_EDGE('',*,*,#26869,.T.);
#35059=ORIENTED_EDGE('',*,*,#26877,.T.);
#35060=ORIENTED_EDGE('',*,*,#26874,.F.);
#35061=ORIENTED_EDGE('',*,*,#26878,.F.);
#35062=ORIENTED_EDGE('',*,*,#26870,.T.);
#35063=ORIENTED_EDGE('',*,*,#26878,.T.);
#35064=ORIENTED_EDGE('',*,*,#26876,.T.);
#35065=ORIENTED_EDGE('',*,*,#26873,.T.);
#35066=ORIENTED_EDGE('',*,*,#26868,.F.);
#35067=ORIENTED_EDGE('',*,*,#26872,.F.);
#35068=ORIENTED_EDGE('',*,*,#26875,.F.);
#35069=ORIENTED_EDGE('',*,*,#26877,.F.);
#35070=ORIENTED_EDGE('',*,*,#26879,.T.);
#35071=ORIENTED_EDGE('',*,*,#26880,.T.);
#35072=ORIENTED_EDGE('',*,*,#26881,.T.);
#35073=ORIENTED_EDGE('',*,*,#26882,.T.);
#35074=ORIENTED_EDGE('',*,*,#26883,.T.);
#35075=ORIENTED_EDGE('',*,*,#26884,.T.);
#35076=ORIENTED_EDGE('',*,*,#26885,.F.);
#35077=ORIENTED_EDGE('',*,*,#26880,.F.);
#35078=ORIENTED_EDGE('',*,*,#26885,.T.);
#35079=ORIENTED_EDGE('',*,*,#26886,.T.);
#35080=ORIENTED_EDGE('',*,*,#26887,.F.);
#35081=ORIENTED_EDGE('',*,*,#26881,.F.);
#35082=ORIENTED_EDGE('',*,*,#26887,.T.);
#35083=ORIENTED_EDGE('',*,*,#26888,.T.);
#35084=ORIENTED_EDGE('',*,*,#26889,.F.);
#35085=ORIENTED_EDGE('',*,*,#26882,.F.);
#35086=ORIENTED_EDGE('',*,*,#26889,.T.);
#35087=ORIENTED_EDGE('',*,*,#26890,.T.);
#35088=ORIENTED_EDGE('',*,*,#26883,.F.);
#35089=ORIENTED_EDGE('',*,*,#26879,.F.);
#35090=ORIENTED_EDGE('',*,*,#26890,.F.);
#35091=ORIENTED_EDGE('',*,*,#26888,.F.);
#35092=ORIENTED_EDGE('',*,*,#26886,.F.);
#35093=ORIENTED_EDGE('',*,*,#26884,.F.);
#35094=ORIENTED_EDGE('',*,*,#26891,.T.);
#35095=ORIENTED_EDGE('',*,*,#26892,.T.);
#35096=ORIENTED_EDGE('',*,*,#26893,.T.);
#35097=ORIENTED_EDGE('',*,*,#26894,.T.);
#35098=ORIENTED_EDGE('',*,*,#26895,.T.);
#35099=ORIENTED_EDGE('',*,*,#26896,.T.);
#35100=ORIENTED_EDGE('',*,*,#26897,.T.);
#35101=ORIENTED_EDGE('',*,*,#26898,.T.);
#35102=ORIENTED_EDGE('',*,*,#26899,.T.);
#35103=ORIENTED_EDGE('',*,*,#26900,.T.);
#35104=ORIENTED_EDGE('',*,*,#26901,.T.);
#35105=ORIENTED_EDGE('',*,*,#26902,.T.);
#35106=ORIENTED_EDGE('',*,*,#26903,.T.);
#35107=ORIENTED_EDGE('',*,*,#26904,.T.);
#35108=ORIENTED_EDGE('',*,*,#26903,.F.);
#35109=ORIENTED_EDGE('',*,*,#26905,.T.);
#35110=ORIENTED_EDGE('',*,*,#26906,.T.);
#35111=ORIENTED_EDGE('',*,*,#26907,.T.);
#35112=ORIENTED_EDGE('',*,*,#26908,.T.);
#35113=ORIENTED_EDGE('',*,*,#26909,.T.);
#35114=ORIENTED_EDGE('',*,*,#26910,.T.);
#35115=ORIENTED_EDGE('',*,*,#26904,.F.);
#35116=ORIENTED_EDGE('',*,*,#26911,.T.);
#35117=ORIENTED_EDGE('',*,*,#26912,.F.);
#35118=ORIENTED_EDGE('',*,*,#26911,.F.);
#35119=ORIENTED_EDGE('',*,*,#26913,.T.);
#35120=ORIENTED_EDGE('',*,*,#26914,.T.);
#35121=ORIENTED_EDGE('',*,*,#26915,.T.);
#35122=ORIENTED_EDGE('',*,*,#26916,.F.);
#35123=ORIENTED_EDGE('',*,*,#26917,.T.);
#35124=ORIENTED_EDGE('',*,*,#26918,.T.);
#35125=ORIENTED_EDGE('',*,*,#26919,.T.);
#35126=ORIENTED_EDGE('',*,*,#26920,.T.);
#35127=ORIENTED_EDGE('',*,*,#26921,.T.);
#35128=ORIENTED_EDGE('',*,*,#26922,.F.);
#35129=ORIENTED_EDGE('',*,*,#26923,.T.);
#35130=ORIENTED_EDGE('',*,*,#26924,.T.);
#35131=ORIENTED_EDGE('',*,*,#26925,.T.);
#35132=ORIENTED_EDGE('',*,*,#26926,.T.);
#35133=ORIENTED_EDGE('',*,*,#26927,.T.);
#35134=ORIENTED_EDGE('',*,*,#26928,.F.);
#35135=ORIENTED_EDGE('',*,*,#26929,.T.);
#35136=ORIENTED_EDGE('',*,*,#26930,.T.);
#35137=ORIENTED_EDGE('',*,*,#26931,.T.);
#35138=ORIENTED_EDGE('',*,*,#26932,.T.);
#35139=ORIENTED_EDGE('',*,*,#26933,.T.);
#35140=ORIENTED_EDGE('',*,*,#26934,.T.);
#35141=ORIENTED_EDGE('',*,*,#26935,.F.);
#35142=ORIENTED_EDGE('',*,*,#26936,.T.);
#35143=ORIENTED_EDGE('',*,*,#26937,.F.);
#35144=ORIENTED_EDGE('',*,*,#26938,.T.);
#35145=ORIENTED_EDGE('',*,*,#26939,.T.);
#35146=ORIENTED_EDGE('',*,*,#26932,.F.);
#35147=ORIENTED_EDGE('',*,*,#26940,.T.);
#35148=ORIENTED_EDGE('',*,*,#26941,.T.);
#35149=ORIENTED_EDGE('',*,*,#26942,.T.);
#35150=ORIENTED_EDGE('',*,*,#26943,.T.);
#35151=ORIENTED_EDGE('',*,*,#26944,.F.);
#35152=ORIENTED_EDGE('',*,*,#26941,.F.);
#35153=ORIENTED_EDGE('',*,*,#26945,.F.);
#35154=ORIENTED_EDGE('',*,*,#26946,.F.);
#35155=ORIENTED_EDGE('',*,*,#26947,.F.);
#35156=ORIENTED_EDGE('',*,*,#26939,.F.);
#35157=ORIENTED_EDGE('',*,*,#26948,.F.);
#35158=ORIENTED_EDGE('',*,*,#26949,.F.);
#35159=ORIENTED_EDGE('',*,*,#26950,.F.);
#35160=ORIENTED_EDGE('',*,*,#26933,.F.);
#35161=ORIENTED_EDGE('',*,*,#26943,.F.);
#35162=ORIENTED_EDGE('',*,*,#26951,.T.);
#35163=ORIENTED_EDGE('',*,*,#26952,.F.);
#35164=ORIENTED_EDGE('',*,*,#26953,.F.);
#35165=ORIENTED_EDGE('',*,*,#26931,.F.);
#35166=ORIENTED_EDGE('',*,*,#26954,.T.);
#35167=ORIENTED_EDGE('',*,*,#26955,.T.);
#35168=ORIENTED_EDGE('',*,*,#26954,.F.);
#35169=ORIENTED_EDGE('',*,*,#26940,.F.);
#35170=ORIENTED_EDGE('',*,*,#26956,.T.);
#35171=ORIENTED_EDGE('',*,*,#26957,.T.);
#35172=ORIENTED_EDGE('',*,*,#26958,.T.);
#35173=ORIENTED_EDGE('',*,*,#26959,.T.);
#35174=ORIENTED_EDGE('',*,*,#26960,.F.);
#35175=ORIENTED_EDGE('',*,*,#26961,.T.);
#35176=ORIENTED_EDGE('',*,*,#26962,.F.);
#35177=ORIENTED_EDGE('',*,*,#26963,.T.);
#35178=ORIENTED_EDGE('',*,*,#26964,.T.);
#35179=ORIENTED_EDGE('',*,*,#26957,.F.);
#35180=ORIENTED_EDGE('',*,*,#26965,.T.);
#35181=ORIENTED_EDGE('',*,*,#26966,.T.);
#35182=ORIENTED_EDGE('',*,*,#26967,.T.);
#35183=ORIENTED_EDGE('',*,*,#26968,.T.);
#35184=ORIENTED_EDGE('',*,*,#26969,.F.);
#35185=ORIENTED_EDGE('',*,*,#26966,.F.);
#35186=ORIENTED_EDGE('',*,*,#26970,.F.);
#35187=ORIENTED_EDGE('',*,*,#26971,.F.);
#35188=ORIENTED_EDGE('',*,*,#26972,.F.);
#35189=ORIENTED_EDGE('',*,*,#26964,.F.);
#35190=ORIENTED_EDGE('',*,*,#26973,.F.);
#35191=ORIENTED_EDGE('',*,*,#26974,.F.);
#35192=ORIENTED_EDGE('',*,*,#26975,.F.);
#35193=ORIENTED_EDGE('',*,*,#26958,.F.);
#35194=ORIENTED_EDGE('',*,*,#26968,.F.);
#35195=ORIENTED_EDGE('',*,*,#26976,.T.);
#35196=ORIENTED_EDGE('',*,*,#26977,.F.);
#35197=ORIENTED_EDGE('',*,*,#26978,.F.);
#35198=ORIENTED_EDGE('',*,*,#26956,.F.);
#35199=ORIENTED_EDGE('',*,*,#26979,.T.);
#35200=ORIENTED_EDGE('',*,*,#26980,.T.);
#35201=ORIENTED_EDGE('',*,*,#26979,.F.);
#35202=ORIENTED_EDGE('',*,*,#26965,.F.);
#35203=ORIENTED_EDGE('',*,*,#26981,.T.);
#35204=ORIENTED_EDGE('',*,*,#26982,.T.);
#35205=ORIENTED_EDGE('',*,*,#26983,.T.);
#35206=ORIENTED_EDGE('',*,*,#26984,.T.);
#35207=ORIENTED_EDGE('',*,*,#26985,.F.);
#35208=ORIENTED_EDGE('',*,*,#26986,.T.);
#35209=ORIENTED_EDGE('',*,*,#26987,.F.);
#35210=ORIENTED_EDGE('',*,*,#26988,.T.);
#35211=ORIENTED_EDGE('',*,*,#26989,.T.);
#35212=ORIENTED_EDGE('',*,*,#26982,.F.);
#35213=ORIENTED_EDGE('',*,*,#26990,.T.);
#35214=ORIENTED_EDGE('',*,*,#26991,.T.);
#35215=ORIENTED_EDGE('',*,*,#26992,.T.);
#35216=ORIENTED_EDGE('',*,*,#26993,.T.);
#35217=ORIENTED_EDGE('',*,*,#26994,.F.);
#35218=ORIENTED_EDGE('',*,*,#26991,.F.);
#35219=ORIENTED_EDGE('',*,*,#26995,.F.);
#35220=ORIENTED_EDGE('',*,*,#26996,.F.);
#35221=ORIENTED_EDGE('',*,*,#26997,.F.);
#35222=ORIENTED_EDGE('',*,*,#26989,.F.);
#35223=ORIENTED_EDGE('',*,*,#26998,.F.);
#35224=ORIENTED_EDGE('',*,*,#26999,.F.);
#35225=ORIENTED_EDGE('',*,*,#27000,.F.);
#35226=ORIENTED_EDGE('',*,*,#26983,.F.);
#35227=ORIENTED_EDGE('',*,*,#26993,.F.);
#35228=ORIENTED_EDGE('',*,*,#27001,.T.);
#35229=ORIENTED_EDGE('',*,*,#27002,.F.);
#35230=ORIENTED_EDGE('',*,*,#27003,.F.);
#35231=ORIENTED_EDGE('',*,*,#26981,.F.);
#35232=ORIENTED_EDGE('',*,*,#27004,.T.);
#35233=ORIENTED_EDGE('',*,*,#27005,.T.);
#35234=ORIENTED_EDGE('',*,*,#27004,.F.);
#35235=ORIENTED_EDGE('',*,*,#26990,.F.);
#35236=ORIENTED_EDGE('',*,*,#27006,.T.);
#35237=ORIENTED_EDGE('',*,*,#27007,.T.);
#35238=ORIENTED_EDGE('',*,*,#27008,.T.);
#35239=ORIENTED_EDGE('',*,*,#27009,.T.);
#35240=ORIENTED_EDGE('',*,*,#27010,.F.);
#35241=ORIENTED_EDGE('',*,*,#27011,.T.);
#35242=ORIENTED_EDGE('',*,*,#27012,.F.);
#35243=ORIENTED_EDGE('',*,*,#27013,.T.);
#35244=ORIENTED_EDGE('',*,*,#27014,.T.);
#35245=ORIENTED_EDGE('',*,*,#27007,.F.);
#35246=ORIENTED_EDGE('',*,*,#27014,.F.);
#35247=ORIENTED_EDGE('',*,*,#27015,.T.);
#35248=ORIENTED_EDGE('',*,*,#27016,.F.);
#35249=ORIENTED_EDGE('',*,*,#27017,.F.);
#35250=ORIENTED_EDGE('',*,*,#27008,.F.);
#35251=ORIENTED_EDGE('',*,*,#27018,.T.);
#35252=ORIENTED_EDGE('',*,*,#27019,.T.);
#35253=ORIENTED_EDGE('',*,*,#27020,.T.);
#35254=ORIENTED_EDGE('',*,*,#27021,.T.);
#35255=ORIENTED_EDGE('',*,*,#27022,.T.);
#35256=ORIENTED_EDGE('',*,*,#27023,.T.);
#35257=ORIENTED_EDGE('',*,*,#27024,.T.);
#35258=ORIENTED_EDGE('',*,*,#27025,.F.);
#35259=ORIENTED_EDGE('',*,*,#27026,.T.);
#35260=ORIENTED_EDGE('',*,*,#27027,.F.);
#35261=ORIENTED_EDGE('',*,*,#27028,.T.);
#35262=ORIENTED_EDGE('',*,*,#27029,.T.);
#35263=ORIENTED_EDGE('',*,*,#27030,.T.);
#35264=ORIENTED_EDGE('',*,*,#27025,.T.);
#35265=ORIENTED_EDGE('',*,*,#27031,.T.);
#35266=ORIENTED_EDGE('',*,*,#27032,.F.);
#35267=ORIENTED_EDGE('',*,*,#27033,.T.);
#35268=ORIENTED_EDGE('',*,*,#27034,.F.);
#35269=ORIENTED_EDGE('',*,*,#27035,.T.);
#35270=ORIENTED_EDGE('',*,*,#27034,.T.);
#35271=ORIENTED_EDGE('',*,*,#27036,.T.);
#35272=ORIENTED_EDGE('',*,*,#27029,.F.);
#35273=ORIENTED_EDGE('',*,*,#27037,.T.);
#35274=ORIENTED_EDGE('',*,*,#27038,.T.);
#35275=ORIENTED_EDGE('',*,*,#27039,.T.);
#35276=ORIENTED_EDGE('',*,*,#27040,.T.);
#35277=ORIENTED_EDGE('',*,*,#27041,.T.);
#35278=ORIENTED_EDGE('',*,*,#27027,.T.);
#35279=ORIENTED_EDGE('',*,*,#27042,.T.);
#35280=ORIENTED_EDGE('',*,*,#27043,.T.);
#35281=ORIENTED_EDGE('',*,*,#27044,.T.);
#35282=ORIENTED_EDGE('',*,*,#27045,.T.);
#35283=ORIENTED_EDGE('',*,*,#27046,.T.);
#35284=ORIENTED_EDGE('',*,*,#27032,.T.);
#35285=ORIENTED_EDGE('',*,*,#27047,.T.);
#35286=ORIENTED_EDGE('',*,*,#27048,.F.);
#35287=ORIENTED_EDGE('',*,*,#27049,.F.);
#35288=ORIENTED_EDGE('',*,*,#27050,.F.);
#35289=ORIENTED_EDGE('',*,*,#27051,.F.);
#35290=ORIENTED_EDGE('',*,*,#27052,.F.);
#35291=ORIENTED_EDGE('',*,*,#27053,.F.);
#35292=ORIENTED_EDGE('',*,*,#27037,.F.);
#35293=ORIENTED_EDGE('',*,*,#27054,.F.);
#35294=ORIENTED_EDGE('',*,*,#27055,.F.);
#35295=ORIENTED_EDGE('',*,*,#27054,.T.);
#35296=ORIENTED_EDGE('',*,*,#27031,.F.);
#35297=ORIENTED_EDGE('',*,*,#27056,.F.);
#35298=ORIENTED_EDGE('',*,*,#27057,.F.);
#35299=ORIENTED_EDGE('',*,*,#27058,.F.);
#35300=ORIENTED_EDGE('',*,*,#27035,.F.);
#35301=ORIENTED_EDGE('',*,*,#27053,.T.);
#35302=ORIENTED_EDGE('',*,*,#27059,.F.);
#35303=ORIENTED_EDGE('',*,*,#27056,.T.);
#35304=ORIENTED_EDGE('',*,*,#27028,.F.);
#35305=ORIENTED_EDGE('',*,*,#27060,.F.);
#35306=ORIENTED_EDGE('',*,*,#27061,.F.);
#35307=ORIENTED_EDGE('',*,*,#27062,.F.);
#35308=ORIENTED_EDGE('',*,*,#27047,.F.);
#35309=ORIENTED_EDGE('',*,*,#27058,.T.);
#35310=ORIENTED_EDGE('',*,*,#27063,.F.);
#35311=ORIENTED_EDGE('',*,*,#27064,.F.);
#35312=ORIENTED_EDGE('',*,*,#27060,.T.);
#35313=ORIENTED_EDGE('',*,*,#27044,.F.);
#35314=ORIENTED_EDGE('',*,*,#27065,.F.);
#35315=ORIENTED_EDGE('',*,*,#27066,.F.);
#35316=ORIENTED_EDGE('',*,*,#27067,.F.);
#35317=ORIENTED_EDGE('',*,*,#27068,.F.);
#35318=ORIENTED_EDGE('',*,*,#27038,.F.);
#35319=ORIENTED_EDGE('',*,*,#27069,.F.);
#35320=ORIENTED_EDGE('',*,*,#27070,.F.);
#35321=ORIENTED_EDGE('',*,*,#27071,.F.);
#35322=ORIENTED_EDGE('',*,*,#27072,.F.);
#35323=ORIENTED_EDGE('',*,*,#27069,.T.);
#35324=ORIENTED_EDGE('',*,*,#27073,.F.);
#35325=ORIENTED_EDGE('',*,*,#27062,.T.);
#35326=ORIENTED_EDGE('',*,*,#27074,.F.);
#35327=ORIENTED_EDGE('',*,*,#27065,.T.);
#35328=ORIENTED_EDGE('',*,*,#27075,.F.);
#35329=ORIENTED_EDGE('',*,*,#27068,.T.);
#35330=ORIENTED_EDGE('',*,*,#27073,.T.);
#35331=ORIENTED_EDGE('',*,*,#27041,.F.);
#35332=ORIENTED_EDGE('',*,*,#27076,.F.);
#35333=ORIENTED_EDGE('',*,*,#27045,.F.);
#35334=ORIENTED_EDGE('',*,*,#27075,.T.);
#35335=ORIENTED_EDGE('',*,*,#27043,.F.);
#35336=ORIENTED_EDGE('',*,*,#27077,.F.);
#35337=ORIENTED_EDGE('',*,*,#27039,.F.);
#35338=ORIENTED_EDGE('',*,*,#27078,.F.);
#35339=ORIENTED_EDGE('',*,*,#27040,.F.);
#35340=ORIENTED_EDGE('',*,*,#27079,.F.);
#35341=ORIENTED_EDGE('',*,*,#27023,.F.);
#35342=ORIENTED_EDGE('',*,*,#27076,.T.);
#35343=ORIENTED_EDGE('',*,*,#27078,.T.);
#35344=ORIENTED_EDGE('',*,*,#27080,.F.);
#35345=ORIENTED_EDGE('',*,*,#27079,.T.);
#35346=ORIENTED_EDGE('',*,*,#27077,.T.);
#35347=ORIENTED_EDGE('',*,*,#27081,.F.);
#35348=ORIENTED_EDGE('',*,*,#27080,.T.);
#35349=ORIENTED_EDGE('',*,*,#27022,.F.);
#35350=ORIENTED_EDGE('',*,*,#27082,.F.);
#35351=ORIENTED_EDGE('',*,*,#27046,.F.);
#35352=ORIENTED_EDGE('',*,*,#27081,.T.);
#35353=ORIENTED_EDGE('',*,*,#27042,.F.);
#35354=ORIENTED_EDGE('',*,*,#27083,.F.);
#35355=ORIENTED_EDGE('',*,*,#27024,.F.);
#35356=ORIENTED_EDGE('',*,*,#27082,.T.);
#35357=ORIENTED_EDGE('',*,*,#27021,.F.);
#35358=ORIENTED_EDGE('',*,*,#27084,.F.);
#35359=ORIENTED_EDGE('',*,*,#27033,.F.);
#35360=ORIENTED_EDGE('',*,*,#27083,.T.);
#35361=ORIENTED_EDGE('',*,*,#27026,.F.);
#35362=ORIENTED_EDGE('',*,*,#27085,.F.);
#35363=ORIENTED_EDGE('',*,*,#27018,.F.);
#35364=ORIENTED_EDGE('',*,*,#27084,.T.);
#35365=ORIENTED_EDGE('',*,*,#27020,.F.);
#35366=ORIENTED_EDGE('',*,*,#27086,.F.);
#35367=ORIENTED_EDGE('',*,*,#27036,.F.);
#35368=ORIENTED_EDGE('',*,*,#27085,.T.);
#35369=ORIENTED_EDGE('',*,*,#27030,.F.);
#35370=ORIENTED_EDGE('',*,*,#27086,.T.);
#35371=ORIENTED_EDGE('',*,*,#27019,.F.);
#35372=ORIENTED_EDGE('',*,*,#27087,.T.);
#35373=ORIENTED_EDGE('',*,*,#27088,.F.);
#35374=ORIENTED_EDGE('',*,*,#27089,.T.);
#35375=ORIENTED_EDGE('',*,*,#27090,.F.);
#35376=ORIENTED_EDGE('',*,*,#27091,.T.);
#35377=ORIENTED_EDGE('',*,*,#27092,.F.);
#35378=ORIENTED_EDGE('',*,*,#27089,.F.);
#35379=ORIENTED_EDGE('',*,*,#27093,.F.);
#35380=ORIENTED_EDGE('',*,*,#27094,.T.);
#35381=ORIENTED_EDGE('',*,*,#27095,.F.);
#35382=ORIENTED_EDGE('',*,*,#27087,.F.);
#35383=ORIENTED_EDGE('',*,*,#27096,.F.);
#35384=ORIENTED_EDGE('',*,*,#27091,.F.);
#35385=ORIENTED_EDGE('',*,*,#27097,.F.);
#35386=ORIENTED_EDGE('',*,*,#27094,.F.);
#35387=ORIENTED_EDGE('',*,*,#27098,.F.);
#35388=ORIENTED_EDGE('',*,*,#27099,.T.);
#35389=ORIENTED_EDGE('',*,*,#27100,.F.);
#35390=ORIENTED_EDGE('',*,*,#27101,.T.);
#35391=ORIENTED_EDGE('',*,*,#27009,.F.);
#35392=ORIENTED_EDGE('',*,*,#27102,.T.);
#35393=ORIENTED_EDGE('',*,*,#27010,.T.);
#35394=ORIENTED_EDGE('',*,*,#27101,.F.);
#35395=ORIENTED_EDGE('',*,*,#27103,.T.);
#35396=ORIENTED_EDGE('',*,*,#27104,.T.);
#35397=ORIENTED_EDGE('',*,*,#27105,.T.);
#35398=ORIENTED_EDGE('',*,*,#27099,.F.);
#35399=ORIENTED_EDGE('',*,*,#27017,.T.);
#35400=ORIENTED_EDGE('',*,*,#27106,.T.);
#35401=ORIENTED_EDGE('',*,*,#27107,.F.);
#35402=ORIENTED_EDGE('',*,*,#27103,.F.);
#35403=ORIENTED_EDGE('',*,*,#27108,.F.);
#35404=ORIENTED_EDGE('',*,*,#27109,.T.);
#35405=ORIENTED_EDGE('',*,*,#27011,.F.);
#35406=ORIENTED_EDGE('',*,*,#27102,.F.);
#35407=ORIENTED_EDGE('',*,*,#27110,.F.);
#35408=ORIENTED_EDGE('',*,*,#27111,.T.);
#35409=ORIENTED_EDGE('',*,*,#27112,.F.);
#35410=ORIENTED_EDGE('',*,*,#27104,.F.);
#35411=ORIENTED_EDGE('',*,*,#27113,.F.);
#35412=ORIENTED_EDGE('',*,*,#27114,.T.);
#35413=ORIENTED_EDGE('',*,*,#27115,.F.);
#35414=ORIENTED_EDGE('',*,*,#27106,.F.);
#35415=ORIENTED_EDGE('',*,*,#27116,.F.);
#35416=ORIENTED_EDGE('',*,*,#27117,.T.);
#35417=ORIENTED_EDGE('',*,*,#27012,.T.);
#35418=ORIENTED_EDGE('',*,*,#27109,.F.);
#35419=ORIENTED_EDGE('',*,*,#27118,.T.);
#35420=ORIENTED_EDGE('',*,*,#27119,.T.);
#35421=ORIENTED_EDGE('',*,*,#27120,.T.);
#35422=ORIENTED_EDGE('',*,*,#27015,.F.);
#35423=ORIENTED_EDGE('',*,*,#27121,.T.);
#35424=ORIENTED_EDGE('',*,*,#27122,.T.);
#35425=ORIENTED_EDGE('',*,*,#27123,.F.);
#35426=ORIENTED_EDGE('',*,*,#27111,.F.);
#35427=ORIENTED_EDGE('',*,*,#27124,.F.);
#35428=ORIENTED_EDGE('',*,*,#27114,.F.);
#35429=ORIENTED_EDGE('',*,*,#27125,.F.);
#35430=ORIENTED_EDGE('',*,*,#27118,.F.);
#35431=ORIENTED_EDGE('',*,*,#27126,.F.);
#35432=ORIENTED_EDGE('',*,*,#27117,.F.);
#35433=ORIENTED_EDGE('',*,*,#27127,.F.);
#35434=ORIENTED_EDGE('',*,*,#27121,.F.);
#35435=ORIENTED_EDGE('',*,*,#27013,.F.);
#35436=ORIENTED_EDGE('',*,*,#27120,.F.);
#35437=ORIENTED_EDGE('',*,*,#27128,.F.);
#35438=ORIENTED_EDGE('',*,*,#27122,.F.);
#35439=ORIENTED_EDGE('',*,*,#27129,.F.);
#35440=ORIENTED_EDGE('',*,*,#27096,.T.);
#35441=ORIENTED_EDGE('',*,*,#27090,.T.);
#35442=ORIENTED_EDGE('',*,*,#27092,.T.);
#35443=ORIENTED_EDGE('',*,*,#27098,.T.);
#35444=ORIENTED_EDGE('',*,*,#27126,.T.);
#35445=ORIENTED_EDGE('',*,*,#27110,.T.);
#35446=ORIENTED_EDGE('',*,*,#27107,.T.);
#35447=ORIENTED_EDGE('',*,*,#27115,.T.);
#35448=ORIENTED_EDGE('',*,*,#27130,.T.);
#35449=ORIENTED_EDGE('',*,*,#27097,.T.);
#35450=ORIENTED_EDGE('',*,*,#27131,.F.);
#35451=ORIENTED_EDGE('',*,*,#27116,.T.);
#35452=ORIENTED_EDGE('',*,*,#27132,.T.);
#35453=ORIENTED_EDGE('',*,*,#27088,.T.);
#35454=ORIENTED_EDGE('',*,*,#27133,.F.);
#35455=ORIENTED_EDGE('',*,*,#27123,.T.);
#35456=ORIENTED_EDGE('',*,*,#27131,.T.);
#35457=ORIENTED_EDGE('',*,*,#27093,.T.);
#35458=ORIENTED_EDGE('',*,*,#27132,.F.);
#35459=ORIENTED_EDGE('',*,*,#27128,.T.);
#35460=ORIENTED_EDGE('',*,*,#27119,.F.);
#35461=ORIENTED_EDGE('',*,*,#27127,.T.);
#35462=ORIENTED_EDGE('',*,*,#27125,.T.);
#35463=ORIENTED_EDGE('',*,*,#27133,.T.);
#35464=ORIENTED_EDGE('',*,*,#27095,.T.);
#35465=ORIENTED_EDGE('',*,*,#27130,.F.);
#35466=ORIENTED_EDGE('',*,*,#27108,.T.);
#35467=ORIENTED_EDGE('',*,*,#27100,.T.);
#35468=ORIENTED_EDGE('',*,*,#27105,.F.);
#35469=ORIENTED_EDGE('',*,*,#27112,.T.);
#35470=ORIENTED_EDGE('',*,*,#27124,.T.);
#35471=ORIENTED_EDGE('',*,*,#27113,.T.);
#35472=ORIENTED_EDGE('',*,*,#27016,.T.);
#35473=ORIENTED_EDGE('',*,*,#27129,.T.);
#35474=ORIENTED_EDGE('',*,*,#27134,.T.);
#35475=ORIENTED_EDGE('',*,*,#27135,.F.);
#35476=ORIENTED_EDGE('',*,*,#27003,.T.);
#35477=ORIENTED_EDGE('',*,*,#27136,.F.);
#35478=ORIENTED_EDGE('',*,*,#27137,.T.);
#35479=ORIENTED_EDGE('',*,*,#27138,.F.);
#35480=ORIENTED_EDGE('',*,*,#27134,.F.);
#35481=ORIENTED_EDGE('',*,*,#27139,.F.);
#35482=ORIENTED_EDGE('',*,*,#27001,.F.);
#35483=ORIENTED_EDGE('',*,*,#27140,.F.);
#35484=ORIENTED_EDGE('',*,*,#27137,.F.);
#35485=ORIENTED_EDGE('',*,*,#27141,.F.);
#35486=ORIENTED_EDGE('',*,*,#27142,.T.);
#35487=ORIENTED_EDGE('',*,*,#26986,.F.);
#35488=ORIENTED_EDGE('',*,*,#27143,.T.);
#35489=ORIENTED_EDGE('',*,*,#27144,.F.);
#35490=ORIENTED_EDGE('',*,*,#27145,.T.);
#35491=ORIENTED_EDGE('',*,*,#27146,.T.);
#35492=ORIENTED_EDGE('',*,*,#27143,.F.);
#35493=ORIENTED_EDGE('',*,*,#26985,.T.);
#35494=ORIENTED_EDGE('',*,*,#27147,.T.);
#35495=ORIENTED_EDGE('',*,*,#26987,.T.);
#35496=ORIENTED_EDGE('',*,*,#27142,.F.);
#35497=ORIENTED_EDGE('',*,*,#27148,.T.);
#35498=ORIENTED_EDGE('',*,*,#27149,.T.);
#35499=ORIENTED_EDGE('',*,*,#27150,.F.);
#35500=ORIENTED_EDGE('',*,*,#27145,.F.);
#35501=ORIENTED_EDGE('',*,*,#26984,.F.);
#35502=ORIENTED_EDGE('',*,*,#27151,.T.);
#35503=ORIENTED_EDGE('',*,*,#27152,.F.);
#35504=ORIENTED_EDGE('',*,*,#27146,.F.);
#35505=ORIENTED_EDGE('',*,*,#27153,.F.);
#35506=ORIENTED_EDGE('',*,*,#27154,.T.);
#35507=ORIENTED_EDGE('',*,*,#27155,.F.);
#35508=ORIENTED_EDGE('',*,*,#27148,.F.);
#35509=ORIENTED_EDGE('',*,*,#27156,.F.);
#35510=ORIENTED_EDGE('',*,*,#27157,.T.);
#35511=ORIENTED_EDGE('',*,*,#26988,.F.);
#35512=ORIENTED_EDGE('',*,*,#27147,.F.);
#35513=ORIENTED_EDGE('',*,*,#27158,.F.);
#35514=ORIENTED_EDGE('',*,*,#27159,.T.);
#35515=ORIENTED_EDGE('',*,*,#27160,.T.);
#35516=ORIENTED_EDGE('',*,*,#27149,.F.);
#35517=ORIENTED_EDGE('',*,*,#27000,.T.);
#35518=ORIENTED_EDGE('',*,*,#27151,.F.);
#35519=ORIENTED_EDGE('',*,*,#27161,.F.);
#35520=ORIENTED_EDGE('',*,*,#27154,.F.);
#35521=ORIENTED_EDGE('',*,*,#27162,.F.);
#35522=ORIENTED_EDGE('',*,*,#27163,.T.);
#35523=ORIENTED_EDGE('',*,*,#26998,.T.);
#35524=ORIENTED_EDGE('',*,*,#27157,.F.);
#35525=ORIENTED_EDGE('',*,*,#27164,.T.);
#35526=ORIENTED_EDGE('',*,*,#26995,.T.);
#35527=ORIENTED_EDGE('',*,*,#27165,.F.);
#35528=ORIENTED_EDGE('',*,*,#27159,.F.);
#35529=ORIENTED_EDGE('',*,*,#27166,.F.);
#35530=ORIENTED_EDGE('',*,*,#26997,.T.);
#35531=ORIENTED_EDGE('',*,*,#27167,.F.);
#35532=ORIENTED_EDGE('',*,*,#27163,.F.);
#35533=ORIENTED_EDGE('',*,*,#27168,.F.);
#35534=ORIENTED_EDGE('',*,*,#27139,.T.);
#35535=ORIENTED_EDGE('',*,*,#27136,.T.);
#35536=ORIENTED_EDGE('',*,*,#27002,.T.);
#35537=ORIENTED_EDGE('',*,*,#27141,.T.);
#35538=ORIENTED_EDGE('',*,*,#27156,.T.);
#35539=ORIENTED_EDGE('',*,*,#27144,.T.);
#35540=ORIENTED_EDGE('',*,*,#27152,.T.);
#35541=ORIENTED_EDGE('',*,*,#27162,.T.);
#35542=ORIENTED_EDGE('',*,*,#27169,.F.);
#35543=ORIENTED_EDGE('',*,*,#27161,.T.);
#35544=ORIENTED_EDGE('',*,*,#27170,.T.);
#35545=ORIENTED_EDGE('',*,*,#27138,.T.);
#35546=ORIENTED_EDGE('',*,*,#27169,.T.);
#35547=ORIENTED_EDGE('',*,*,#27140,.T.);
#35548=ORIENTED_EDGE('',*,*,#26992,.F.);
#35549=ORIENTED_EDGE('',*,*,#27168,.T.);
#35550=ORIENTED_EDGE('',*,*,#27164,.F.);
#35551=ORIENTED_EDGE('',*,*,#27158,.T.);
#35552=ORIENTED_EDGE('',*,*,#27155,.T.);
#35553=ORIENTED_EDGE('',*,*,#26994,.T.);
#35554=ORIENTED_EDGE('',*,*,#27135,.T.);
#35555=ORIENTED_EDGE('',*,*,#27170,.F.);
#35556=ORIENTED_EDGE('',*,*,#27153,.T.);
#35557=ORIENTED_EDGE('',*,*,#27150,.T.);
#35558=ORIENTED_EDGE('',*,*,#27160,.F.);
#35559=ORIENTED_EDGE('',*,*,#27165,.T.);
#35560=ORIENTED_EDGE('',*,*,#27167,.T.);
#35561=ORIENTED_EDGE('',*,*,#26996,.T.);
#35562=ORIENTED_EDGE('',*,*,#27166,.T.);
#35563=ORIENTED_EDGE('',*,*,#26999,.T.);
#35564=ORIENTED_EDGE('',*,*,#27171,.T.);
#35565=ORIENTED_EDGE('',*,*,#27172,.F.);
#35566=ORIENTED_EDGE('',*,*,#26978,.T.);
#35567=ORIENTED_EDGE('',*,*,#27173,.F.);
#35568=ORIENTED_EDGE('',*,*,#27174,.T.);
#35569=ORIENTED_EDGE('',*,*,#27175,.F.);
#35570=ORIENTED_EDGE('',*,*,#27171,.F.);
#35571=ORIENTED_EDGE('',*,*,#27176,.F.);
#35572=ORIENTED_EDGE('',*,*,#26976,.F.);
#35573=ORIENTED_EDGE('',*,*,#27177,.F.);
#35574=ORIENTED_EDGE('',*,*,#27174,.F.);
#35575=ORIENTED_EDGE('',*,*,#27178,.F.);
#35576=ORIENTED_EDGE('',*,*,#27179,.T.);
#35577=ORIENTED_EDGE('',*,*,#26961,.F.);
#35578=ORIENTED_EDGE('',*,*,#27180,.T.);
#35579=ORIENTED_EDGE('',*,*,#27181,.F.);
#35580=ORIENTED_EDGE('',*,*,#27182,.T.);
#35581=ORIENTED_EDGE('',*,*,#27183,.T.);
#35582=ORIENTED_EDGE('',*,*,#27180,.F.);
#35583=ORIENTED_EDGE('',*,*,#26960,.T.);
#35584=ORIENTED_EDGE('',*,*,#27184,.T.);
#35585=ORIENTED_EDGE('',*,*,#26962,.T.);
#35586=ORIENTED_EDGE('',*,*,#27179,.F.);
#35587=ORIENTED_EDGE('',*,*,#27185,.T.);
#35588=ORIENTED_EDGE('',*,*,#27186,.T.);
#35589=ORIENTED_EDGE('',*,*,#27187,.F.);
#35590=ORIENTED_EDGE('',*,*,#27182,.F.);
#35591=ORIENTED_EDGE('',*,*,#26959,.F.);
#35592=ORIENTED_EDGE('',*,*,#27188,.T.);
#35593=ORIENTED_EDGE('',*,*,#27189,.F.);
#35594=ORIENTED_EDGE('',*,*,#27183,.F.);
#35595=ORIENTED_EDGE('',*,*,#27190,.F.);
#35596=ORIENTED_EDGE('',*,*,#27191,.T.);
#35597=ORIENTED_EDGE('',*,*,#27192,.F.);
#35598=ORIENTED_EDGE('',*,*,#27185,.F.);
#35599=ORIENTED_EDGE('',*,*,#27193,.F.);
#35600=ORIENTED_EDGE('',*,*,#27194,.T.);
#35601=ORIENTED_EDGE('',*,*,#26963,.F.);
#35602=ORIENTED_EDGE('',*,*,#27184,.F.);
#35603=ORIENTED_EDGE('',*,*,#27195,.F.);
#35604=ORIENTED_EDGE('',*,*,#27196,.T.);
#35605=ORIENTED_EDGE('',*,*,#27197,.T.);
#35606=ORIENTED_EDGE('',*,*,#27186,.F.);
#35607=ORIENTED_EDGE('',*,*,#26975,.T.);
#35608=ORIENTED_EDGE('',*,*,#27188,.F.);
#35609=ORIENTED_EDGE('',*,*,#27198,.F.);
#35610=ORIENTED_EDGE('',*,*,#27191,.F.);
#35611=ORIENTED_EDGE('',*,*,#27199,.F.);
#35612=ORIENTED_EDGE('',*,*,#27200,.T.);
#35613=ORIENTED_EDGE('',*,*,#26973,.T.);
#35614=ORIENTED_EDGE('',*,*,#27194,.F.);
#35615=ORIENTED_EDGE('',*,*,#27201,.T.);
#35616=ORIENTED_EDGE('',*,*,#26970,.T.);
#35617=ORIENTED_EDGE('',*,*,#27202,.F.);
#35618=ORIENTED_EDGE('',*,*,#27196,.F.);
#35619=ORIENTED_EDGE('',*,*,#27203,.F.);
#35620=ORIENTED_EDGE('',*,*,#26972,.T.);
#35621=ORIENTED_EDGE('',*,*,#27204,.F.);
#35622=ORIENTED_EDGE('',*,*,#27200,.F.);
#35623=ORIENTED_EDGE('',*,*,#27205,.F.);
#35624=ORIENTED_EDGE('',*,*,#27176,.T.);
#35625=ORIENTED_EDGE('',*,*,#27173,.T.);
#35626=ORIENTED_EDGE('',*,*,#26977,.T.);
#35627=ORIENTED_EDGE('',*,*,#27178,.T.);
#35628=ORIENTED_EDGE('',*,*,#27193,.T.);
#35629=ORIENTED_EDGE('',*,*,#27181,.T.);
#35630=ORIENTED_EDGE('',*,*,#27189,.T.);
#35631=ORIENTED_EDGE('',*,*,#27199,.T.);
#35632=ORIENTED_EDGE('',*,*,#27206,.F.);
#35633=ORIENTED_EDGE('',*,*,#27198,.T.);
#35634=ORIENTED_EDGE('',*,*,#27207,.T.);
#35635=ORIENTED_EDGE('',*,*,#27175,.T.);
#35636=ORIENTED_EDGE('',*,*,#27206,.T.);
#35637=ORIENTED_EDGE('',*,*,#27177,.T.);
#35638=ORIENTED_EDGE('',*,*,#26967,.F.);
#35639=ORIENTED_EDGE('',*,*,#27205,.T.);
#35640=ORIENTED_EDGE('',*,*,#27201,.F.);
#35641=ORIENTED_EDGE('',*,*,#27195,.T.);
#35642=ORIENTED_EDGE('',*,*,#27192,.T.);
#35643=ORIENTED_EDGE('',*,*,#26969,.T.);
#35644=ORIENTED_EDGE('',*,*,#27172,.T.);
#35645=ORIENTED_EDGE('',*,*,#27207,.F.);
#35646=ORIENTED_EDGE('',*,*,#27190,.T.);
#35647=ORIENTED_EDGE('',*,*,#27187,.T.);
#35648=ORIENTED_EDGE('',*,*,#27197,.F.);
#35649=ORIENTED_EDGE('',*,*,#27202,.T.);
#35650=ORIENTED_EDGE('',*,*,#27204,.T.);
#35651=ORIENTED_EDGE('',*,*,#26971,.T.);
#35652=ORIENTED_EDGE('',*,*,#27203,.T.);
#35653=ORIENTED_EDGE('',*,*,#26974,.T.);
#35654=ORIENTED_EDGE('',*,*,#27208,.T.);
#35655=ORIENTED_EDGE('',*,*,#27209,.F.);
#35656=ORIENTED_EDGE('',*,*,#26953,.T.);
#35657=ORIENTED_EDGE('',*,*,#27210,.F.);
#35658=ORIENTED_EDGE('',*,*,#27211,.T.);
#35659=ORIENTED_EDGE('',*,*,#27212,.F.);
#35660=ORIENTED_EDGE('',*,*,#27208,.F.);
#35661=ORIENTED_EDGE('',*,*,#27213,.F.);
#35662=ORIENTED_EDGE('',*,*,#26951,.F.);
#35663=ORIENTED_EDGE('',*,*,#27214,.F.);
#35664=ORIENTED_EDGE('',*,*,#27211,.F.);
#35665=ORIENTED_EDGE('',*,*,#27215,.F.);
#35666=ORIENTED_EDGE('',*,*,#27216,.T.);
#35667=ORIENTED_EDGE('',*,*,#26936,.F.);
#35668=ORIENTED_EDGE('',*,*,#27217,.T.);
#35669=ORIENTED_EDGE('',*,*,#27218,.F.);
#35670=ORIENTED_EDGE('',*,*,#27219,.T.);
#35671=ORIENTED_EDGE('',*,*,#27220,.T.);
#35672=ORIENTED_EDGE('',*,*,#27217,.F.);
#35673=ORIENTED_EDGE('',*,*,#26935,.T.);
#35674=ORIENTED_EDGE('',*,*,#27221,.T.);
#35675=ORIENTED_EDGE('',*,*,#26937,.T.);
#35676=ORIENTED_EDGE('',*,*,#27216,.F.);
#35677=ORIENTED_EDGE('',*,*,#27222,.T.);
#35678=ORIENTED_EDGE('',*,*,#27223,.T.);
#35679=ORIENTED_EDGE('',*,*,#27224,.F.);
#35680=ORIENTED_EDGE('',*,*,#27219,.F.);
#35681=ORIENTED_EDGE('',*,*,#26934,.F.);
#35682=ORIENTED_EDGE('',*,*,#27225,.T.);
#35683=ORIENTED_EDGE('',*,*,#27226,.F.);
#35684=ORIENTED_EDGE('',*,*,#27220,.F.);
#35685=ORIENTED_EDGE('',*,*,#27227,.F.);
#35686=ORIENTED_EDGE('',*,*,#27228,.T.);
#35687=ORIENTED_EDGE('',*,*,#27229,.F.);
#35688=ORIENTED_EDGE('',*,*,#27222,.F.);
#35689=ORIENTED_EDGE('',*,*,#27230,.F.);
#35690=ORIENTED_EDGE('',*,*,#27231,.T.);
#35691=ORIENTED_EDGE('',*,*,#26938,.F.);
#35692=ORIENTED_EDGE('',*,*,#27221,.F.);
#35693=ORIENTED_EDGE('',*,*,#27232,.F.);
#35694=ORIENTED_EDGE('',*,*,#27233,.T.);
#35695=ORIENTED_EDGE('',*,*,#27234,.T.);
#35696=ORIENTED_EDGE('',*,*,#27223,.F.);
#35697=ORIENTED_EDGE('',*,*,#26950,.T.);
#35698=ORIENTED_EDGE('',*,*,#27225,.F.);
#35699=ORIENTED_EDGE('',*,*,#27235,.F.);
#35700=ORIENTED_EDGE('',*,*,#27228,.F.);
#35701=ORIENTED_EDGE('',*,*,#27236,.F.);
#35702=ORIENTED_EDGE('',*,*,#27237,.T.);
#35703=ORIENTED_EDGE('',*,*,#26948,.T.);
#35704=ORIENTED_EDGE('',*,*,#27231,.F.);
#35705=ORIENTED_EDGE('',*,*,#27238,.T.);
#35706=ORIENTED_EDGE('',*,*,#26945,.T.);
#35707=ORIENTED_EDGE('',*,*,#27239,.F.);
#35708=ORIENTED_EDGE('',*,*,#27233,.F.);
#35709=ORIENTED_EDGE('',*,*,#27240,.F.);
#35710=ORIENTED_EDGE('',*,*,#26947,.T.);
#35711=ORIENTED_EDGE('',*,*,#27241,.F.);
#35712=ORIENTED_EDGE('',*,*,#27237,.F.);
#35713=ORIENTED_EDGE('',*,*,#27242,.F.);
#35714=ORIENTED_EDGE('',*,*,#27213,.T.);
#35715=ORIENTED_EDGE('',*,*,#27210,.T.);
#35716=ORIENTED_EDGE('',*,*,#26952,.T.);
#35717=ORIENTED_EDGE('',*,*,#27215,.T.);
#35718=ORIENTED_EDGE('',*,*,#27230,.T.);
#35719=ORIENTED_EDGE('',*,*,#27218,.T.);
#35720=ORIENTED_EDGE('',*,*,#27226,.T.);
#35721=ORIENTED_EDGE('',*,*,#27236,.T.);
#35722=ORIENTED_EDGE('',*,*,#27243,.F.);
#35723=ORIENTED_EDGE('',*,*,#27235,.T.);
#35724=ORIENTED_EDGE('',*,*,#27244,.T.);
#35725=ORIENTED_EDGE('',*,*,#27212,.T.);
#35726=ORIENTED_EDGE('',*,*,#27243,.T.);
#35727=ORIENTED_EDGE('',*,*,#27214,.T.);
#35728=ORIENTED_EDGE('',*,*,#26942,.F.);
#35729=ORIENTED_EDGE('',*,*,#27242,.T.);
#35730=ORIENTED_EDGE('',*,*,#27238,.F.);
#35731=ORIENTED_EDGE('',*,*,#27232,.T.);
#35732=ORIENTED_EDGE('',*,*,#27229,.T.);
#35733=ORIENTED_EDGE('',*,*,#26944,.T.);
#35734=ORIENTED_EDGE('',*,*,#27209,.T.);
#35735=ORIENTED_EDGE('',*,*,#27244,.F.);
#35736=ORIENTED_EDGE('',*,*,#27227,.T.);
#35737=ORIENTED_EDGE('',*,*,#27224,.T.);
#35738=ORIENTED_EDGE('',*,*,#27234,.F.);
#35739=ORIENTED_EDGE('',*,*,#27239,.T.);
#35740=ORIENTED_EDGE('',*,*,#27241,.T.);
#35741=ORIENTED_EDGE('',*,*,#26946,.T.);
#35742=ORIENTED_EDGE('',*,*,#27240,.T.);
#35743=ORIENTED_EDGE('',*,*,#26949,.T.);
#35744=ORIENTED_EDGE('',*,*,#26925,.F.);
#35745=ORIENTED_EDGE('',*,*,#27245,.F.);
#35746=ORIENTED_EDGE('',*,*,#26919,.F.);
#35747=ORIENTED_EDGE('',*,*,#27246,.F.);
#35748=ORIENTED_EDGE('',*,*,#26913,.F.);
#35749=ORIENTED_EDGE('',*,*,#27247,.F.);
#35750=ORIENTED_EDGE('',*,*,#27248,.T.);
#35751=ORIENTED_EDGE('',*,*,#27063,.T.);
#35752=ORIENTED_EDGE('',*,*,#27249,.T.);
#35753=ORIENTED_EDGE('',*,*,#27250,.F.);
#35754=ORIENTED_EDGE('',*,*,#27249,.F.);
#35755=ORIENTED_EDGE('',*,*,#27057,.T.);
#35756=ORIENTED_EDGE('',*,*,#27251,.T.);
#35757=ORIENTED_EDGE('',*,*,#27252,.F.);
#35758=ORIENTED_EDGE('',*,*,#27072,.T.);
#35759=ORIENTED_EDGE('',*,*,#27061,.T.);
#35760=ORIENTED_EDGE('',*,*,#27248,.F.);
#35761=ORIENTED_EDGE('',*,*,#27253,.F.);
#35762=ORIENTED_EDGE('',*,*,#27254,.T.);
#35763=ORIENTED_EDGE('',*,*,#27070,.T.);
#35764=ORIENTED_EDGE('',*,*,#27251,.F.);
#35765=ORIENTED_EDGE('',*,*,#27052,.T.);
#35766=ORIENTED_EDGE('',*,*,#27255,.T.);
#35767=ORIENTED_EDGE('',*,*,#27256,.F.);
#35768=ORIENTED_EDGE('',*,*,#27257,.T.);
#35769=ORIENTED_EDGE('',*,*,#27071,.T.);
#35770=ORIENTED_EDGE('',*,*,#27254,.F.);
#35771=ORIENTED_EDGE('',*,*,#27258,.F.);
#35772=ORIENTED_EDGE('',*,*,#27255,.F.);
#35773=ORIENTED_EDGE('',*,*,#27051,.T.);
#35774=ORIENTED_EDGE('',*,*,#27259,.T.);
#35775=ORIENTED_EDGE('',*,*,#27260,.F.);
#35776=ORIENTED_EDGE('',*,*,#27261,.T.);
#35777=ORIENTED_EDGE('',*,*,#27066,.T.);
#35778=ORIENTED_EDGE('',*,*,#27074,.T.);
#35779=ORIENTED_EDGE('',*,*,#27067,.T.);
#35780=ORIENTED_EDGE('',*,*,#27257,.F.);
#35781=ORIENTED_EDGE('',*,*,#27262,.F.);
#35782=ORIENTED_EDGE('',*,*,#27259,.F.);
#35783=ORIENTED_EDGE('',*,*,#27050,.T.);
#35784=ORIENTED_EDGE('',*,*,#27263,.T.);
#35785=ORIENTED_EDGE('',*,*,#27264,.F.);
#35786=ORIENTED_EDGE('',*,*,#27265,.T.);
#35787=ORIENTED_EDGE('',*,*,#27064,.T.);
#35788=ORIENTED_EDGE('',*,*,#27261,.F.);
#35789=ORIENTED_EDGE('',*,*,#27266,.F.);
#35790=ORIENTED_EDGE('',*,*,#27263,.F.);
#35791=ORIENTED_EDGE('',*,*,#27049,.T.);
#35792=ORIENTED_EDGE('',*,*,#27267,.T.);
#35793=ORIENTED_EDGE('',*,*,#27268,.F.);
#35794=ORIENTED_EDGE('',*,*,#27269,.T.);
#35795=ORIENTED_EDGE('',*,*,#27059,.T.);
#35796=ORIENTED_EDGE('',*,*,#27265,.F.);
#35797=ORIENTED_EDGE('',*,*,#27270,.F.);
#35798=ORIENTED_EDGE('',*,*,#27267,.F.);
#35799=ORIENTED_EDGE('',*,*,#27048,.T.);
#35800=ORIENTED_EDGE('',*,*,#27271,.T.);
#35801=ORIENTED_EDGE('',*,*,#27272,.F.);
#35802=ORIENTED_EDGE('',*,*,#27271,.F.);
#35803=ORIENTED_EDGE('',*,*,#27055,.T.);
#35804=ORIENTED_EDGE('',*,*,#27269,.F.);
#35805=ORIENTED_EDGE('',*,*,#27273,.F.);
#35806=ORIENTED_EDGE('',*,*,#27274,.F.);
#35807=ORIENTED_EDGE('',*,*,#27262,.T.);
#35808=ORIENTED_EDGE('',*,*,#27275,.F.);
#35809=ORIENTED_EDGE('',*,*,#27276,.T.);
#35810=ORIENTED_EDGE('',*,*,#27277,.T.);
#35811=ORIENTED_EDGE('',*,*,#27278,.F.);
#35812=ORIENTED_EDGE('',*,*,#27276,.F.);
#35813=ORIENTED_EDGE('',*,*,#27279,.F.);
#35814=ORIENTED_EDGE('',*,*,#27280,.T.);
#35815=ORIENTED_EDGE('',*,*,#27281,.F.);
#35816=ORIENTED_EDGE('',*,*,#27277,.F.);
#35817=ORIENTED_EDGE('',*,*,#27282,.F.);
#35818=ORIENTED_EDGE('',*,*,#27283,.T.);
#35819=ORIENTED_EDGE('',*,*,#27284,.T.);
#35820=ORIENTED_EDGE('',*,*,#27280,.F.);
#35821=ORIENTED_EDGE('',*,*,#27285,.T.);
#35822=ORIENTED_EDGE('',*,*,#27286,.T.);
#35823=ORIENTED_EDGE('',*,*,#26896,.F.);
#35824=ORIENTED_EDGE('',*,*,#27283,.F.);
#35825=ORIENTED_EDGE('',*,*,#27287,.F.);
#35826=ORIENTED_EDGE('',*,*,#27288,.T.);
#35827=ORIENTED_EDGE('',*,*,#27289,.F.);
#35828=ORIENTED_EDGE('',*,*,#27284,.F.);
#35829=ORIENTED_EDGE('',*,*,#26895,.F.);
#35830=ORIENTED_EDGE('',*,*,#27290,.T.);
#35831=ORIENTED_EDGE('',*,*,#27291,.T.);
#35832=ORIENTED_EDGE('',*,*,#27286,.F.);
#35833=ORIENTED_EDGE('',*,*,#27292,.T.);
#35834=ORIENTED_EDGE('',*,*,#27293,.T.);
#35835=ORIENTED_EDGE('',*,*,#27294,.F.);
#35836=ORIENTED_EDGE('',*,*,#27288,.F.);
#35837=ORIENTED_EDGE('',*,*,#26894,.F.);
#35838=ORIENTED_EDGE('',*,*,#27295,.T.);
#35839=ORIENTED_EDGE('',*,*,#27296,.F.);
#35840=ORIENTED_EDGE('',*,*,#27290,.F.);
#35841=ORIENTED_EDGE('',*,*,#27297,.F.);
#35842=ORIENTED_EDGE('',*,*,#27298,.T.);
#35843=ORIENTED_EDGE('',*,*,#26897,.F.);
#35844=ORIENTED_EDGE('',*,*,#27291,.F.);
#35845=ORIENTED_EDGE('',*,*,#27299,.F.);
#35846=ORIENTED_EDGE('',*,*,#27300,.T.);
#35847=ORIENTED_EDGE('',*,*,#27301,.F.);
#35848=ORIENTED_EDGE('',*,*,#27293,.F.);
#35849=ORIENTED_EDGE('',*,*,#26893,.F.);
#35850=ORIENTED_EDGE('',*,*,#27302,.F.);
#35851=ORIENTED_EDGE('',*,*,#27253,.T.);
#35852=ORIENTED_EDGE('',*,*,#27303,.F.);
#35853=ORIENTED_EDGE('',*,*,#27295,.F.);
#35854=ORIENTED_EDGE('',*,*,#27304,.T.);
#35855=ORIENTED_EDGE('',*,*,#26898,.F.);
#35856=ORIENTED_EDGE('',*,*,#27298,.F.);
#35857=ORIENTED_EDGE('',*,*,#27305,.F.);
#35858=ORIENTED_EDGE('',*,*,#27306,.T.);
#35859=ORIENTED_EDGE('',*,*,#27307,.F.);
#35860=ORIENTED_EDGE('',*,*,#27300,.F.);
#35861=ORIENTED_EDGE('',*,*,#27308,.T.);
#35862=ORIENTED_EDGE('',*,*,#26899,.F.);
#35863=ORIENTED_EDGE('',*,*,#27304,.F.);
#35864=ORIENTED_EDGE('',*,*,#27309,.F.);
#35865=ORIENTED_EDGE('',*,*,#27310,.T.);
#35866=ORIENTED_EDGE('',*,*,#27311,.F.);
#35867=ORIENTED_EDGE('',*,*,#27306,.F.);
#35868=ORIENTED_EDGE('',*,*,#26892,.F.);
#35869=ORIENTED_EDGE('',*,*,#27312,.F.);
#35870=ORIENTED_EDGE('',*,*,#27313,.T.);
#35871=ORIENTED_EDGE('',*,*,#27308,.F.);
#35872=ORIENTED_EDGE('',*,*,#27314,.T.);
#35873=ORIENTED_EDGE('',*,*,#27315,.F.);
#35874=ORIENTED_EDGE('',*,*,#27310,.F.);
#35875=ORIENTED_EDGE('',*,*,#26891,.F.);
#35876=ORIENTED_EDGE('',*,*,#26910,.F.);
#35877=ORIENTED_EDGE('',*,*,#27316,.T.);
#35878=ORIENTED_EDGE('',*,*,#26900,.F.);
#35879=ORIENTED_EDGE('',*,*,#27313,.F.);
#35880=ORIENTED_EDGE('',*,*,#27317,.F.);
#35881=ORIENTED_EDGE('',*,*,#27318,.T.);
#35882=ORIENTED_EDGE('',*,*,#27319,.F.);
#35883=ORIENTED_EDGE('',*,*,#27314,.F.);
#35884=ORIENTED_EDGE('',*,*,#26909,.F.);
#35885=ORIENTED_EDGE('',*,*,#27320,.T.);
#35886=ORIENTED_EDGE('',*,*,#26901,.F.);
#35887=ORIENTED_EDGE('',*,*,#27316,.F.);
#35888=ORIENTED_EDGE('',*,*,#27321,.F.);
#35889=ORIENTED_EDGE('',*,*,#27322,.T.);
#35890=ORIENTED_EDGE('',*,*,#27268,.T.);
#35891=ORIENTED_EDGE('',*,*,#27323,.F.);
#35892=ORIENTED_EDGE('',*,*,#27318,.F.);
#35893=ORIENTED_EDGE('',*,*,#26908,.F.);
#35894=ORIENTED_EDGE('',*,*,#27324,.T.);
#35895=ORIENTED_EDGE('',*,*,#26905,.F.);
#35896=ORIENTED_EDGE('',*,*,#26902,.F.);
#35897=ORIENTED_EDGE('',*,*,#27320,.F.);
#35898=ORIENTED_EDGE('',*,*,#27325,.F.);
#35899=ORIENTED_EDGE('',*,*,#27326,.T.);
#35900=ORIENTED_EDGE('',*,*,#27264,.T.);
#35901=ORIENTED_EDGE('',*,*,#27322,.F.);
#35902=ORIENTED_EDGE('',*,*,#26907,.F.);
#35903=ORIENTED_EDGE('',*,*,#27327,.F.);
#35904=ORIENTED_EDGE('',*,*,#27260,.T.);
#35905=ORIENTED_EDGE('',*,*,#27326,.F.);
#35906=ORIENTED_EDGE('',*,*,#26906,.F.);
#35907=ORIENTED_EDGE('',*,*,#27324,.F.);
#35908=ORIENTED_EDGE('',*,*,#26912,.T.);
#35909=ORIENTED_EDGE('',*,*,#27006,.F.);
#35910=ORIENTED_EDGE('',*,*,#27328,.T.);
#35911=ORIENTED_EDGE('',*,*,#27329,.F.);
#35912=ORIENTED_EDGE('',*,*,#27330,.T.);
#35913=ORIENTED_EDGE('',*,*,#27331,.F.);
#35914=ORIENTED_EDGE('',*,*,#27332,.T.);
#35915=ORIENTED_EDGE('',*,*,#27333,.T.);
#35916=ORIENTED_EDGE('',*,*,#27330,.F.);
#35917=ORIENTED_EDGE('',*,*,#27334,.T.);
#35918=ORIENTED_EDGE('',*,*,#27335,.F.);
#35919=ORIENTED_EDGE('',*,*,#27315,.T.);
#35920=ORIENTED_EDGE('',*,*,#27336,.F.);
#35921=ORIENTED_EDGE('',*,*,#27328,.F.);
#35922=ORIENTED_EDGE('',*,*,#27337,.T.);
#35923=ORIENTED_EDGE('',*,*,#27338,.F.);
#35924=ORIENTED_EDGE('',*,*,#27332,.F.);
#35925=ORIENTED_EDGE('',*,*,#27339,.F.);
#35926=ORIENTED_EDGE('',*,*,#27340,.F.);
#35927=ORIENTED_EDGE('',*,*,#27341,.F.);
#35928=ORIENTED_EDGE('',*,*,#27342,.T.);
#35929=ORIENTED_EDGE('',*,*,#27343,.T.);
#35930=ORIENTED_EDGE('',*,*,#27344,.T.);
#35931=ORIENTED_EDGE('',*,*,#27345,.F.);
#35932=ORIENTED_EDGE('',*,*,#27337,.F.);
#35933=ORIENTED_EDGE('',*,*,#27346,.F.);
#35934=ORIENTED_EDGE('',*,*,#27347,.T.);
#35935=ORIENTED_EDGE('',*,*,#27348,.F.);
#35936=ORIENTED_EDGE('',*,*,#27342,.F.);
#35937=ORIENTED_EDGE('',*,*,#27349,.F.);
#35938=ORIENTED_EDGE('',*,*,#27350,.F.);
#35939=ORIENTED_EDGE('',*,*,#27305,.T.);
#35940=ORIENTED_EDGE('',*,*,#27351,.F.);
#35941=ORIENTED_EDGE('',*,*,#27347,.F.);
#35942=ORIENTED_EDGE('',*,*,#27352,.T.);
#35943=ORIENTED_EDGE('',*,*,#26928,.T.);
#35944=ORIENTED_EDGE('',*,*,#27353,.T.);
#35945=ORIENTED_EDGE('',*,*,#27338,.T.);
#35946=ORIENTED_EDGE('',*,*,#27345,.T.);
#35947=ORIENTED_EDGE('',*,*,#27354,.T.);
#35948=ORIENTED_EDGE('',*,*,#27301,.T.);
#35949=ORIENTED_EDGE('',*,*,#27355,.T.);
#35950=ORIENTED_EDGE('',*,*,#26922,.T.);
#35951=ORIENTED_EDGE('',*,*,#27356,.T.);
#35952=ORIENTED_EDGE('',*,*,#26916,.T.);
#35953=ORIENTED_EDGE('',*,*,#27005,.F.);
#35954=ORIENTED_EDGE('',*,*,#26980,.F.);
#35955=ORIENTED_EDGE('',*,*,#26955,.F.);
#35956=ORIENTED_EDGE('',*,*,#27357,.F.);
#35957=ORIENTED_EDGE('',*,*,#27270,.T.);
#35958=ORIENTED_EDGE('',*,*,#27358,.F.);
#35959=ORIENTED_EDGE('',*,*,#27359,.T.);
#35960=ORIENTED_EDGE('',*,*,#27334,.F.);
#35961=ORIENTED_EDGE('',*,*,#27329,.T.);
#35962=ORIENTED_EDGE('',*,*,#27360,.T.);
#35963=ORIENTED_EDGE('',*,*,#27361,.F.);
#35964=ORIENTED_EDGE('',*,*,#27359,.F.);
#35965=ORIENTED_EDGE('',*,*,#27362,.F.);
#35966=ORIENTED_EDGE('',*,*,#27339,.T.);
#35967=ORIENTED_EDGE('',*,*,#27363,.F.);
#35968=ORIENTED_EDGE('',*,*,#27325,.T.);
#35969=ORIENTED_EDGE('',*,*,#27364,.T.);
#35970=ORIENTED_EDGE('',*,*,#27343,.F.);
#35971=ORIENTED_EDGE('',*,*,#27348,.T.);
#35972=ORIENTED_EDGE('',*,*,#27365,.F.);
#35973=ORIENTED_EDGE('',*,*,#27366,.T.);
#35974=ORIENTED_EDGE('',*,*,#27367,.F.);
#35975=ORIENTED_EDGE('',*,*,#27252,.T.);
#35976=ORIENTED_EDGE('',*,*,#27368,.F.);
#35977=ORIENTED_EDGE('',*,*,#27366,.F.);
#35978=ORIENTED_EDGE('',*,*,#27369,.T.);
#35979=ORIENTED_EDGE('',*,*,#27273,.T.);
#35980=ORIENTED_EDGE('',*,*,#27357,.T.);
#35981=ORIENTED_EDGE('',*,*,#27361,.T.);
#35982=ORIENTED_EDGE('',*,*,#27368,.T.);
#35983=ORIENTED_EDGE('',*,*,#27256,.T.);
#35984=ORIENTED_EDGE('',*,*,#27327,.T.);
#35985=ORIENTED_EDGE('',*,*,#27363,.T.);
#35986=ORIENTED_EDGE('',*,*,#27275,.T.);
#35987=ORIENTED_EDGE('',*,*,#27258,.T.);
#35988=ORIENTED_EDGE('',*,*,#27302,.T.);
#35989=ORIENTED_EDGE('',*,*,#27297,.T.);
#35990=ORIENTED_EDGE('',*,*,#27292,.F.);
#35991=ORIENTED_EDGE('',*,*,#27287,.T.);
#35992=ORIENTED_EDGE('',*,*,#27285,.F.);
#35993=ORIENTED_EDGE('',*,*,#27282,.T.);
#35994=ORIENTED_EDGE('',*,*,#27279,.T.);
#35995=ORIENTED_EDGE('',*,*,#27358,.T.);
#35996=ORIENTED_EDGE('',*,*,#27266,.T.);
#35997=ORIENTED_EDGE('',*,*,#27274,.T.);
#35998=ORIENTED_EDGE('',*,*,#27370,.F.);
#35999=ORIENTED_EDGE('',*,*,#27303,.T.);
#36000=ORIENTED_EDGE('',*,*,#27250,.T.);
#36001=ORIENTED_EDGE('',*,*,#27367,.T.);
#36002=ORIENTED_EDGE('',*,*,#27371,.T.);
#36003=ORIENTED_EDGE('',*,*,#27299,.T.);
#36004=ORIENTED_EDGE('',*,*,#27296,.T.);
#36005=ORIENTED_EDGE('',*,*,#27371,.F.);
#36006=ORIENTED_EDGE('',*,*,#27365,.T.);
#36007=ORIENTED_EDGE('',*,*,#27351,.T.);
#36008=ORIENTED_EDGE('',*,*,#27370,.T.);
#36009=ORIENTED_EDGE('',*,*,#27278,.T.);
#36010=ORIENTED_EDGE('',*,*,#27372,.F.);
#36011=ORIENTED_EDGE('',*,*,#27346,.T.);
#36012=ORIENTED_EDGE('',*,*,#27362,.T.);
#36013=ORIENTED_EDGE('',*,*,#27364,.F.);
#36014=ORIENTED_EDGE('',*,*,#27321,.T.);
#36015=ORIENTED_EDGE('',*,*,#27373,.F.);
#36016=ORIENTED_EDGE('',*,*,#27340,.T.);
#36017=ORIENTED_EDGE('',*,*,#27374,.F.);
#36018=ORIENTED_EDGE('',*,*,#27312,.T.);
#36019=ORIENTED_EDGE('',*,*,#27375,.F.);
#36020=ORIENTED_EDGE('',*,*,#27341,.T.);
#36021=ORIENTED_EDGE('',*,*,#27376,.F.);
#36022=ORIENTED_EDGE('',*,*,#27294,.T.);
#36023=ORIENTED_EDGE('',*,*,#27354,.F.);
#36024=ORIENTED_EDGE('',*,*,#27344,.F.);
#36025=ORIENTED_EDGE('',*,*,#27375,.T.);
#36026=ORIENTED_EDGE('',*,*,#27309,.T.);
#36027=ORIENTED_EDGE('',*,*,#27350,.T.);
#36028=ORIENTED_EDGE('',*,*,#27349,.T.);
#36029=ORIENTED_EDGE('',*,*,#27373,.T.);
#36030=ORIENTED_EDGE('',*,*,#27317,.T.);
#36031=ORIENTED_EDGE('',*,*,#27374,.T.);
#36032=ORIENTED_EDGE('',*,*,#27336,.T.);
#36033=ORIENTED_EDGE('',*,*,#27319,.T.);
#36034=ORIENTED_EDGE('',*,*,#27377,.F.);
#36035=ORIENTED_EDGE('',*,*,#27360,.F.);
#36036=ORIENTED_EDGE('',*,*,#27372,.T.);
#36037=ORIENTED_EDGE('',*,*,#27281,.T.);
#36038=ORIENTED_EDGE('',*,*,#27289,.T.);
#36039=ORIENTED_EDGE('',*,*,#27376,.T.);
#36040=ORIENTED_EDGE('',*,*,#27323,.T.);
#36041=ORIENTED_EDGE('',*,*,#27272,.T.);
#36042=ORIENTED_EDGE('',*,*,#27369,.F.);
#36043=ORIENTED_EDGE('',*,*,#27377,.T.);
#36044=ORIENTED_EDGE('',*,*,#26921,.F.);
#36045=ORIENTED_EDGE('',*,*,#27378,.F.);
#36046=ORIENTED_EDGE('',*,*,#26917,.F.);
#36047=ORIENTED_EDGE('',*,*,#27356,.F.);
#36048=ORIENTED_EDGE('',*,*,#26923,.F.);
#36049=ORIENTED_EDGE('',*,*,#27355,.F.);
#36050=ORIENTED_EDGE('',*,*,#27307,.T.);
#36051=ORIENTED_EDGE('',*,*,#27379,.F.);
#36052=ORIENTED_EDGE('',*,*,#26927,.F.);
#36053=ORIENTED_EDGE('',*,*,#27380,.F.);
#36054=ORIENTED_EDGE('',*,*,#27333,.F.);
#36055=ORIENTED_EDGE('',*,*,#27353,.F.);
#36056=ORIENTED_EDGE('',*,*,#26929,.F.);
#36057=ORIENTED_EDGE('',*,*,#27352,.F.);
#36058=ORIENTED_EDGE('',*,*,#26915,.F.);
#36059=ORIENTED_EDGE('',*,*,#27381,.F.);
#36060=ORIENTED_EDGE('',*,*,#26930,.F.);
#36061=ORIENTED_EDGE('',*,*,#27381,.T.);
#36062=ORIENTED_EDGE('',*,*,#26914,.F.);
#36063=ORIENTED_EDGE('',*,*,#27247,.T.);
#36064=ORIENTED_EDGE('',*,*,#26918,.F.);
#36065=ORIENTED_EDGE('',*,*,#27378,.T.);
#36066=ORIENTED_EDGE('',*,*,#26920,.F.);
#36067=ORIENTED_EDGE('',*,*,#27246,.T.);
#36068=ORIENTED_EDGE('',*,*,#26924,.F.);
#36069=ORIENTED_EDGE('',*,*,#27379,.T.);
#36070=ORIENTED_EDGE('',*,*,#27311,.T.);
#36071=ORIENTED_EDGE('',*,*,#27335,.T.);
#36072=ORIENTED_EDGE('',*,*,#27331,.T.);
#36073=ORIENTED_EDGE('',*,*,#27380,.T.);
#36074=ORIENTED_EDGE('',*,*,#26926,.F.);
#36075=ORIENTED_EDGE('',*,*,#27245,.T.);
#41963=TOROIDAL_SURFACE('',#48190,27.5226030790361,1.);
#41964=TOROIDAL_SURFACE('',#48211,4.46802221877416,0.5);
#41965=TOROIDAL_SURFACE('',#48215,15.5,0.5);
#41966=TOROIDAL_SURFACE('',#48217,3.46802221877416,0.5);
#41967=TOROIDAL_SURFACE('',#48221,15.5,0.5);
#41968=TOROIDAL_SURFACE('',#48233,4.46802221877416,0.5);
#41969=TOROIDAL_SURFACE('',#48237,15.5,0.5);
#41970=TOROIDAL_SURFACE('',#48239,3.46802221877416,0.5);
#41971=TOROIDAL_SURFACE('',#48243,15.5,0.5);
#41972=TOROIDAL_SURFACE('',#48255,4.46802221877416,0.5);
#41973=TOROIDAL_SURFACE('',#48259,15.5,0.5);
#41974=TOROIDAL_SURFACE('',#48261,3.46802221877416,0.5);
#41975=TOROIDAL_SURFACE('',#48265,15.5,0.5);
#41976=TOROIDAL_SURFACE('',#48273,25.3226030790361,0.7);
#41977=TOROIDAL_SURFACE('',#48290,29.5,0.5);
#41978=TOROIDAL_SURFACE('',#48293,29.5,0.5);
#41979=TOROIDAL_SURFACE('',#48322,29.5,0.5);
#41980=TOROIDAL_SURFACE('',#48324,29.5,0.5);
#41981=TOROIDAL_SURFACE('',#48327,4.05563473233925,0.7);
#41982=TOROIDAL_SURFACE('',#48336,4.05563473233925,0.7);
#41983=TOROIDAL_SURFACE('',#48346,26.7226030790361,0.7);
#41984=TOROIDAL_SURFACE('',#48351,4.05563473233925,0.7);
#41985=TOROIDAL_SURFACE('',#48358,5.45563473233925,0.7);
#41986=TOROIDAL_SURFACE('',#48374,3.46802221877416,0.5);
#41987=TOROIDAL_SURFACE('',#48379,16.5,0.5);
#41988=TOROIDAL_SURFACE('',#48394,3.46802221877416,0.5);
#41989=TOROIDAL_SURFACE('',#48408,3.46802221877416,0.5);
#41990=TOROIDAL_SURFACE('',#48413,16.5,0.5);
#41991=TOROIDAL_SURFACE('',#48428,3.46802221877416,0.5);
#41992=TOROIDAL_SURFACE('',#48442,3.46802221877416,0.5);
#41993=TOROIDAL_SURFACE('',#48447,16.5,0.5);
#41994=TOROIDAL_SURFACE('',#48462,3.46802221877416,0.5);
#41995=TOROIDAL_SURFACE('',#48480,29.5,0.5);
#41996=TOROIDAL_SURFACE('',#48495,29.5,0.5);
#41997=TOROIDAL_SURFACE('',#48503,2.,1.);
#41998=TOROIDAL_SURFACE('',#48507,27.5226030790361,1.);
#41999=TOROIDAL_SURFACE('',#48512,2.,1.);
#42000=TOROIDAL_SURFACE('',#48520,29.5226030790361,1.);
#42001=TOROIDAL_SURFACE('',#48528,29.5226030790361,1.);
#43476=ADVANCED_FACE('',(#10896),#8541,.F.);
#43477=ADVANCED_FACE('',(#10897),#3575,.F.);
#43478=ADVANCED_FACE('',(#10898),#8542,.F.);
#43479=ADVANCED_FACE('',(#10899),#3576,.F.);
#43480=ADVANCED_FACE('',(#10900),#3577,.F.);
#43481=ADVANCED_FACE('',(#10901),#3578,.F.);
#43482=ADVANCED_FACE('',(#10902),#3579,.T.);
#43483=ADVANCED_FACE('',(#10903),#3580,.F.);
#43484=ADVANCED_FACE('',(#10904),#8543,.F.);
#43485=ADVANCED_FACE('',(#10905),#3581,.F.);
#43486=ADVANCED_FACE('',(#10906),#8544,.F.);
#43487=ADVANCED_FACE('',(#10907),#3582,.F.);
#43488=ADVANCED_FACE('',(#10908),#8545,.T.);
#43489=ADVANCED_FACE('',(#10909),#41963,.T.);
#43490=ADVANCED_FACE('',(#10910),#8546,.F.);
#43491=ADVANCED_FACE('',(#10911),#8547,.F.);
#43492=ADVANCED_FACE('',(#10912),#8548,.F.);
#43493=ADVANCED_FACE('',(#10913),#8549,.T.);
#43494=ADVANCED_FACE('',(#10914),#8550,.T.);
#43495=ADVANCED_FACE('',(#10915),#41964,.F.);
#43496=ADVANCED_FACE('',(#10916),#41965,.T.);
#43497=ADVANCED_FACE('',(#10917),#41966,.T.);
#43498=ADVANCED_FACE('',(#10918),#41967,.T.);
#43499=ADVANCED_FACE('',(#10919),#8551,.T.);
#43500=ADVANCED_FACE('',(#10920),#8552,.T.);
#43501=ADVANCED_FACE('',(#10921),#41968,.F.);
#43502=ADVANCED_FACE('',(#10922),#41969,.T.);
#43503=ADVANCED_FACE('',(#10923),#41970,.T.);
#43504=ADVANCED_FACE('',(#10924),#41971,.T.);
#43505=ADVANCED_FACE('',(#10925),#8553,.T.);
#43506=ADVANCED_FACE('',(#10926),#8554,.T.);
#43507=ADVANCED_FACE('',(#10927),#41972,.F.);
#43508=ADVANCED_FACE('',(#10928),#41973,.T.);
#43509=ADVANCED_FACE('',(#10929),#41974,.T.);
#43510=ADVANCED_FACE('',(#10930),#41975,.T.);
#43511=ADVANCED_FACE('',(#10931),#8555,.T.);
#43512=ADVANCED_FACE('',(#10932),#41976,.T.);
#43513=ADVANCED_FACE('',(#10933),#3583,.F.);
#43514=ADVANCED_FACE('',(#10934),#8556,.T.);
#43515=ADVANCED_FACE('',(#10935),#50,.T.);
#43516=ADVANCED_FACE('',(#10936),#8557,.T.);
#43517=ADVANCED_FACE('',(#10937),#51,.T.);
#43518=ADVANCED_FACE('',(#10938),#3584,.T.);
#43519=ADVANCED_FACE('',(#10939),#3585,.F.);
#43520=ADVANCED_FACE('',(#10940),#3586,.F.);
#43521=ADVANCED_FACE('',(#10941),#1607,.T.);
#43522=ADVANCED_FACE('',(#10942),#1608,.T.);
#43523=ADVANCED_FACE('',(#10943),#41977,.T.);
#43524=ADVANCED_FACE('',(#10944),#41978,.T.);
#43525=ADVANCED_FACE('',(#10945),#8558,.T.);
#43526=ADVANCED_FACE('',(#10946),#8559,.T.);
#43527=ADVANCED_FACE('',(#10947),#8560,.T.);
#43528=ADVANCED_FACE('',(#10948),#60,.T.);
#43529=ADVANCED_FACE('',(#10949),#61,.T.);
#43530=ADVANCED_FACE('',(#10950),#8561,.T.);
#43531=ADVANCED_FACE('',(#10951),#8562,.T.);
#43532=ADVANCED_FACE('',(#10952),#8563,.T.);
#43533=ADVANCED_FACE('',(#10953),#62,.T.);
#43534=ADVANCED_FACE('',(#10954),#63,.T.);
#43535=ADVANCED_FACE('',(#10955),#8564,.T.);
#43536=ADVANCED_FACE('',(#10956),#8565,.T.);
#43537=ADVANCED_FACE('',(#10957),#41979,.T.);
#43538=ADVANCED_FACE('',(#10958),#41980,.T.);
#43539=ADVANCED_FACE('',(#10959),#1609,.T.);
#43540=ADVANCED_FACE('',(#10960),#1610,.T.);
#43541=ADVANCED_FACE('',(#10961),#41981,.T.);
#43542=ADVANCED_FACE('',(#10962),#8566,.T.);
#43543=ADVANCED_FACE('',(#10963),#8567,.T.);
#43544=ADVANCED_FACE('',(#10964),#41982,.T.);
#43545=ADVANCED_FACE('',(#10965),#8568,.F.);
#43546=ADVANCED_FACE('',(#10966),#1611,.F.);
#43547=ADVANCED_FACE('',(#10967),#1612,.F.);
#43548=ADVANCED_FACE('',(#10968),#8569,.T.);
#43549=ADVANCED_FACE('',(#10969),#41983,.F.);
#43550=ADVANCED_FACE('',(#10970),#8570,.F.);
#43551=ADVANCED_FACE('',(#10971),#41984,.T.);
#43552=ADVANCED_FACE('',(#10972),#1613,.F.);
#43553=ADVANCED_FACE('',(#10973),#1614,.F.);
#43554=ADVANCED_FACE('',(#10974),#41985,.F.);
#43555=ADVANCED_FACE('',(#10975),#8571,.T.);
#43556=ADVANCED_FACE('',(#10976),#8572,.F.);
#43557=ADVANCED_FACE('',(#10977),#8573,.F.);
#43558=ADVANCED_FACE('',(#10978),#3587,.T.);
#43559=ADVANCED_FACE('',(#10979),#3588,.F.);
#43560=ADVANCED_FACE('',(#10980),#8574,.T.);
#43561=ADVANCED_FACE('',(#10981),#8575,.T.);
#43562=ADVANCED_FACE('',(#10982),#3589,.T.);
#43563=ADVANCED_FACE('',(#10983),#3590,.T.);
#43564=ADVANCED_FACE('',(#10984),#3591,.T.);
#43565=ADVANCED_FACE('',(#10985),#8576,.T.);
#43566=ADVANCED_FACE('',(#10986),#41986,.T.);
#43567=ADVANCED_FACE('',(#10987),#8577,.T.);
#43568=ADVANCED_FACE('',(#10988),#41987,.F.);
#43569=ADVANCED_FACE('',(#10989),#1615,.F.);
#43570=ADVANCED_FACE('',(#10990),#1616,.F.);
#43571=ADVANCED_FACE('',(#10991),#8578,.F.);
#43572=ADVANCED_FACE('',(#10992),#8579,.T.);
#43573=ADVANCED_FACE('',(#10993),#8580,.T.);
#43574=ADVANCED_FACE('',(#10994),#8581,.F.);
#43575=ADVANCED_FACE('',(#10995),#1617,.F.);
#43576=ADVANCED_FACE('',(#10996),#41988,.T.);
#43577=ADVANCED_FACE('',(#10997),#1618,.F.);
#43578=ADVANCED_FACE('',(#10998),#8582,.F.);
#43579=ADVANCED_FACE('',(#10999),#8583,.F.);
#43580=ADVANCED_FACE('',(#11000),#3592,.T.);
#43581=ADVANCED_FACE('',(#11001),#3593,.F.);
#43582=ADVANCED_FACE('',(#11002),#8584,.T.);
#43583=ADVANCED_FACE('',(#11003),#3594,.T.);
#43584=ADVANCED_FACE('',(#11004),#3595,.T.);
#43585=ADVANCED_FACE('',(#11005),#3596,.T.);
#43586=ADVANCED_FACE('',(#11006),#8585,.T.);
#43587=ADVANCED_FACE('',(#11007),#41989,.T.);
#43588=ADVANCED_FACE('',(#11008),#8586,.T.);
#43589=ADVANCED_FACE('',(#11009),#41990,.F.);
#43590=ADVANCED_FACE('',(#11010),#1619,.F.);
#43591=ADVANCED_FACE('',(#11011),#1620,.F.);
#43592=ADVANCED_FACE('',(#11012),#8587,.F.);
#43593=ADVANCED_FACE('',(#11013),#8588,.T.);
#43594=ADVANCED_FACE('',(#11014),#8589,.T.);
#43595=ADVANCED_FACE('',(#11015),#8590,.F.);
#43596=ADVANCED_FACE('',(#11016),#1621,.F.);
#43597=ADVANCED_FACE('',(#11017),#41991,.T.);
#43598=ADVANCED_FACE('',(#11018),#1622,.F.);
#43599=ADVANCED_FACE('',(#11019),#8591,.F.);
#43600=ADVANCED_FACE('',(#11020),#8592,.F.);
#43601=ADVANCED_FACE('',(#11021),#3597,.T.);
#43602=ADVANCED_FACE('',(#11022),#3598,.F.);
#43603=ADVANCED_FACE('',(#11023),#8593,.T.);
#43604=ADVANCED_FACE('',(#11024),#3599,.T.);
#43605=ADVANCED_FACE('',(#11025),#3600,.T.);
#43606=ADVANCED_FACE('',(#11026),#3601,.T.);
#43607=ADVANCED_FACE('',(#11027),#8594,.T.);
#43608=ADVANCED_FACE('',(#11028),#41992,.T.);
#43609=ADVANCED_FACE('',(#11029),#8595,.T.);
#43610=ADVANCED_FACE('',(#11030),#41993,.F.);
#43611=ADVANCED_FACE('',(#11031),#1623,.F.);
#43612=ADVANCED_FACE('',(#11032),#1624,.F.);
#43613=ADVANCED_FACE('',(#11033),#8596,.F.);
#43614=ADVANCED_FACE('',(#11034),#8597,.T.);
#43615=ADVANCED_FACE('',(#11035),#8598,.T.);
#43616=ADVANCED_FACE('',(#11036),#8599,.F.);
#43617=ADVANCED_FACE('',(#11037),#1625,.F.);
#43618=ADVANCED_FACE('',(#11038),#41994,.T.);
#43619=ADVANCED_FACE('',(#11039),#1626,.F.);
#43620=ADVANCED_FACE('',(#11040),#8600,.F.);
#43621=ADVANCED_FACE('',(#11041),#8601,.F.);
#43622=ADVANCED_FACE('',(#11042),#3602,.T.);
#43623=ADVANCED_FACE('',(#11043),#3603,.F.);
#43624=ADVANCED_FACE('',(#11044),#8602,.T.);
#43625=ADVANCED_FACE('',(#11045),#3604,.T.);
#43626=ADVANCED_FACE('',(#11046),#3605,.T.);
#43627=ADVANCED_FACE('',(#11047),#3606,.T.);
#43628=ADVANCED_FACE('',(#11048),#3607,.F.);
#43629=ADVANCED_FACE('',(#11049),#3608,.F.);
#43630=ADVANCED_FACE('',(#11050),#3609,.F.);
#43631=ADVANCED_FACE('',(#11051),#8603,.T.);
#43632=ADVANCED_FACE('',(#11052),#41995,.T.);
#43633=ADVANCED_FACE('',(#11053),#1627,.F.);
#43634=ADVANCED_FACE('',(#11054),#1628,.T.);
#43635=ADVANCED_FACE('',(#11055),#8604,.T.);
#43636=ADVANCED_FACE('',(#11056),#1629,.T.);
#43637=ADVANCED_FACE('',(#11057),#1630,.F.);
#43638=ADVANCED_FACE('',(#11058),#1631,.T.);
#43639=ADVANCED_FACE('',(#11059),#8605,.T.);
#43640=ADVANCED_FACE('',(#11060),#1632,.T.);
#43641=ADVANCED_FACE('',(#11061),#41996,.T.);
#43642=ADVANCED_FACE('',(#11062),#1633,.T.);
#43643=ADVANCED_FACE('',(#11063),#1634,.T.);
#43644=ADVANCED_FACE('',(#11064),#8606,.T.);
#43645=ADVANCED_FACE('',(#11065),#1635,.T.);
#43646=ADVANCED_FACE('',(#11066),#1636,.T.);
#43647=ADVANCED_FACE('',(#11067),#41997,.T.);
#43648=ADVANCED_FACE('',(#11068),#41998,.T.);
#43649=ADVANCED_FACE('',(#11069),#8607,.F.);
#43650=ADVANCED_FACE('',(#11070),#41999,.T.);
#43651=ADVANCED_FACE('',(#11071),#1637,.F.);
#43652=ADVANCED_FACE('',(#11072),#1638,.T.);
#43653=ADVANCED_FACE('',(#11073),#8608,.F.);
#43654=ADVANCED_FACE('',(#11074),#42000,.F.);
#43655=ADVANCED_FACE('',(#11075),#8609,.T.);
#43656=ADVANCED_FACE('',(#11076),#1639,.F.);
#43657=ADVANCED_FACE('',(#11077),#64,.F.);
#43658=ADVANCED_FACE('',(#11078),#42001,.F.);
#43659=ADVANCED_FACE('',(#11079),#8610,.F.);
#43660=ADVANCED_FACE('',(#11080),#65,.F.);
#43661=ADVANCED_FACE('',(#11081),#1640,.F.);
#43662=ADVANCED_FACE('',(#11082),#8611,.F.);
#43663=ADVANCED_FACE('',(#11083),#1641,.F.);
#43664=ADVANCED_FACE('',(#11084),#1642,.F.);
#43665=ADVANCED_FACE('',(#11085),#1643,.F.);
#43666=ADVANCED_FACE('',(#11086),#1644,.F.);
#43667=ADVANCED_FACE('',(#11087),#1645,.F.);
#43668=ADVANCED_FACE('',(#11088),#1646,.F.);
#43669=ADVANCED_FACE('',(#11089,#717),#3610,.F.);
#43670=ADVANCED_FACE('',(#11090),#1647,.T.);
#43671=ADVANCED_FACE('',(#11091),#1648,.T.);
#43672=ADVANCED_FACE('',(#11092),#1649,.T.);
#43673=ADVANCED_FACE('',(#11093),#1650,.T.);
#43674=ADVANCED_FACE('',(#11094),#1651,.T.);
#43675=ADVANCED_FACE('',(#11095),#1652,.T.);
#43676=ADVANCED_FACE('',(#11096),#1653,.T.);
#43677=ADVANCED_FACE('',(#11097),#1654,.T.);
#43678=ADVANCED_FACE('',(#11098,#718,#719,#720),#3611,.F.);
#43679=ADVANCED_FACE('',(#11099),#8612,.T.);
#43680=ADVANCED_FACE('',(#11100),#1655,.T.);
#43681=ADVANCED_FACE('',(#11101),#1656,.T.);
#43682=ADVANCED_FACE('',(#11102),#8613,.T.);
#43683=ADVANCED_FACE('',(#11103),#52,.T.);
#43684=ADVANCED_FACE('',(#11104),#53,.T.);
#43685=ADVANCED_FACE('',(#11105),#3612,.T.);
#43686=ADVANCED_FACE('',(#11106),#3613,.F.);
#43687=ADVANCED_FACE('',(#11107),#3614,.F.);
#43688=ADVANCED_FACE('',(#11108),#54,.F.);
#43689=ADVANCED_FACE('',(#11109),#55,.F.);
#43690=ADVANCED_FACE('',(#11110),#1657,.T.);
#43691=ADVANCED_FACE('',(#11111),#8614,.F.);
#43692=ADVANCED_FACE('',(#11112),#1658,.T.);
#43693=ADVANCED_FACE('',(#11113),#3615,.F.);
#43694=ADVANCED_FACE('',(#11114),#3616,.F.);
#43695=ADVANCED_FACE('',(#11115),#1659,.T.);
#43696=ADVANCED_FACE('',(#11116),#56,.F.);
#43697=ADVANCED_FACE('',(#11117),#57,.T.);
#43698=ADVANCED_FACE('',(#11118),#8615,.F.);
#43699=ADVANCED_FACE('',(#11119),#8616,.F.);
#43700=ADVANCED_FACE('',(#11120),#8617,.F.);
#43701=ADVANCED_FACE('',(#11121),#8618,.F.);
#43702=ADVANCED_FACE('',(#11122),#3617,.F.);
#45453=CLOSED_SHELL('',(#43476,#43477,#43478,#43479,#43480,#43481));
#45454=CLOSED_SHELL('',(#43482,#43483,#43484,#43485,#43486,#43487));
#45455=CLOSED_SHELL('',(#43488,#43489,#43490,#43491,#43492,#43493,#43494,
#43495,#43496,#43497,#43498,#43499,#43500,#43501,#43502,#43503,#43504,#43505,
#43506,#43507,#43508,#43509,#43510,#43511,#43512,#43513,#43514,#43515,#43516,
#43517,#43518,#43519,#43520,#43521,#43522,#43523,#43524,#43525,#43526,#43527,
#43528,#43529,#43530,#43531,#43532,#43533,#43534,#43535,#43536,#43537,#43538,
#43539,#43540,#43541,#43542,#43543,#43544,#43545,#43546,#43547,#43548,#43549,
#43550,#43551,#43552,#43553,#43554,#43555,#43556,#43557,#43558,#43559,#43560,
#43561,#43562,#43563,#43564,#43565,#43566,#43567,#43568,#43569,#43570,#43571,
#43572,#43573,#43574,#43575,#43576,#43577,#43578,#43579,#43580,#43581,#43582,
#43583,#43584,#43585,#43586,#43587,#43588,#43589,#43590,#43591,#43592,#43593,
#43594,#43595,#43596,#43597,#43598,#43599,#43600,#43601,#43602,#43603,#43604,
#43605,#43606,#43607,#43608,#43609,#43610,#43611,#43612,#43613,#43614,#43615,
#43616,#43617,#43618,#43619,#43620,#43621,#43622,#43623,#43624,#43625,#43626,
#43627,#43628,#43629,#43630,#43631,#43632,#43633,#43634,#43635,#43636,#43637,
#43638,#43639,#43640,#43641,#43642,#43643,#43644,#43645,#43646,#43647,#43648,
#43649,#43650,#43651,#43652,#43653,#43654,#43655,#43656,#43657,#43658,#43659,
#43660,#43661,#43662,#43663,#43664,#43665,#43666,#43667,#43668,#43669,#43670,
#43671,#43672,#43673,#43674,#43675,#43676,#43677,#43678,#43679,#43680,#43681,
#43682,#43683,#43684,#43685,#43686,#43687,#43688,#43689,#43690,#43691,#43692,
#43693,#43694,#43695,#43696,#43697,#43698,#43699,#43700,#43701,#43702));
#48162=AXIS2_PLACEMENT_3D('',#85906,#57537,#57538);
#48163=AXIS2_PLACEMENT_3D('',#85907,#57539,#57540);
#48164=AXIS2_PLACEMENT_3D('',#85912,#57542,#57543);
#48165=AXIS2_PLACEMENT_3D('',#85915,#57545,#57546);
#48166=AXIS2_PLACEMENT_3D('',#85916,#57547,#57548);
#48167=AXIS2_PLACEMENT_3D('',#85922,#57552,#57553);
#48168=AXIS2_PLACEMENT_3D('',#85926,#57555,#57556);
#48169=AXIS2_PLACEMENT_3D('',#85927,#57557,#57558);
#48170=AXIS2_PLACEMENT_3D('',#85928,#57559,#57560);
#48171=AXIS2_PLACEMENT_3D('',#85931,#57563,#57564);
#48172=AXIS2_PLACEMENT_3D('',#85932,#57565,#57566);
#48173=AXIS2_PLACEMENT_3D('',#85933,#57567,#57568);
#48174=AXIS2_PLACEMENT_3D('',#85936,#57569,#57570);
#48175=AXIS2_PLACEMENT_3D('',#85940,#57572,#57573);
#48176=AXIS2_PLACEMENT_3D('',#85942,#57575,#57576);
#48177=AXIS2_PLACEMENT_3D('',#85948,#57580,#57581);
#48178=AXIS2_PLACEMENT_3D('',#85950,#57582,#57583);
#48179=AXIS2_PLACEMENT_3D('',#85952,#57585,#57586);
#48180=AXIS2_PLACEMENT_3D('',#85956,#57589,#57590);
#48181=AXIS2_PLACEMENT_3D('',#85957,#57591,#57592);
#48182=AXIS2_PLACEMENT_3D('',#85958,#57593,#57594);
#48183=AXIS2_PLACEMENT_3D('',#85959,#57595,#57596);
#48184=AXIS2_PLACEMENT_3D('',#86020,#57598,#57599);
#48185=AXIS2_PLACEMENT_3D('',#86083,#57601,#57602);
#48186=AXIS2_PLACEMENT_3D('',#86143,#57604,#57605);
#48187=AXIS2_PLACEMENT_3D('',#86185,#57607,#57608);
#48188=AXIS2_PLACEMENT_3D('',#86188,#57610,#57611);
#48189=AXIS2_PLACEMENT_3D('',#86377,#57612,#57613);
#48190=AXIS2_PLACEMENT_3D('',#86378,#57614,#57615);
#48191=AXIS2_PLACEMENT_3D('',#86380,#57616,#57617);
#48192=AXIS2_PLACEMENT_3D('',#86381,#57618,#57619);
#48193=AXIS2_PLACEMENT_3D('',#86382,#57620,#57621);
#48194=AXIS2_PLACEMENT_3D('',#86385,#57622,#57623);
#48195=AXIS2_PLACEMENT_3D('',#86400,#57625,#57626);
#48196=AXIS2_PLACEMENT_3D('',#86413,#57628,#57629);
#48197=AXIS2_PLACEMENT_3D('',#86416,#57630,#57631);
#48198=AXIS2_PLACEMENT_3D('',#86431,#57633,#57634);
#48199=AXIS2_PLACEMENT_3D('',#86444,#57636,#57637);
#48200=AXIS2_PLACEMENT_3D('',#86447,#57638,#57639);
#48201=AXIS2_PLACEMENT_3D('',#86462,#57641,#57642);
#48202=AXIS2_PLACEMENT_3D('',#86475,#57644,#57645);
#48203=AXIS2_PLACEMENT_3D('',#86478,#57646,#57647);
#48204=AXIS2_PLACEMENT_3D('',#86482,#57649,#57650);
#48205=AXIS2_PLACEMENT_3D('',#86536,#57652,#57653);
#48206=AXIS2_PLACEMENT_3D('',#86598,#57655,#57656);
#48207=AXIS2_PLACEMENT_3D('',#86599,#57657,#57658);
#48208=AXIS2_PLACEMENT_3D('',#86600,#57659,#57660);
#48209=AXIS2_PLACEMENT_3D('',#86603,#57661,#57662);
#48210=AXIS2_PLACEMENT_3D('',#86607,#57664,#57665);
#48211=AXIS2_PLACEMENT_3D('',#86609,#57667,#57668);
#48212=AXIS2_PLACEMENT_3D('',#86611,#57669,#57670);
#48213=AXIS2_PLACEMENT_3D('',#86613,#57671,#57672);
#48214=AXIS2_PLACEMENT_3D('',#86614,#57673,#57674);
#48215=AXIS2_PLACEMENT_3D('',#86615,#57675,#57676);
#48216=AXIS2_PLACEMENT_3D('',#86661,#57677,#57678);
#48217=AXIS2_PLACEMENT_3D('',#86708,#57679,#57680);
#48218=AXIS2_PLACEMENT_3D('',#86710,#57681,#57682);
#48219=AXIS2_PLACEMENT_3D('',#86712,#57683,#57684);
#48220=AXIS2_PLACEMENT_3D('',#86713,#57685,#57686);
#48221=AXIS2_PLACEMENT_3D('',#86714,#57687,#57688);
#48222=AXIS2_PLACEMENT_3D('',#86716,#57689,#57690);
#48223=AXIS2_PLACEMENT_3D('',#86717,#57691,#57692);
#48224=AXIS2_PLACEMENT_3D('',#86718,#57693,#57694);
#48225=AXIS2_PLACEMENT_3D('',#86721,#57695,#57696);
#48226=AXIS2_PLACEMENT_3D('',#86725,#57698,#57699);
#48227=AXIS2_PLACEMENT_3D('',#86779,#57701,#57702);
#48228=AXIS2_PLACEMENT_3D('',#86841,#57704,#57705);
#48229=AXIS2_PLACEMENT_3D('',#86842,#57706,#57707);
#48230=AXIS2_PLACEMENT_3D('',#86843,#57708,#57709);
#48231=AXIS2_PLACEMENT_3D('',#86846,#57710,#57711);
#48232=AXIS2_PLACEMENT_3D('',#86850,#57713,#57714);
#48233=AXIS2_PLACEMENT_3D('',#86852,#57716,#57717);
#48234=AXIS2_PLACEMENT_3D('',#86854,#57718,#57719);
#48235=AXIS2_PLACEMENT_3D('',#86856,#57720,#57721);
#48236=AXIS2_PLACEMENT_3D('',#86857,#57722,#57723);
#48237=AXIS2_PLACEMENT_3D('',#86858,#57724,#57725);
#48238=AXIS2_PLACEMENT_3D('',#86904,#57726,#57727);
#48239=AXIS2_PLACEMENT_3D('',#86951,#57728,#57729);
#48240=AXIS2_PLACEMENT_3D('',#86953,#57730,#57731);
#48241=AXIS2_PLACEMENT_3D('',#86955,#57732,#57733);
#48242=AXIS2_PLACEMENT_3D('',#86956,#57734,#57735);
#48243=AXIS2_PLACEMENT_3D('',#86957,#57736,#57737);
#48244=AXIS2_PLACEMENT_3D('',#86959,#57738,#57739);
#48245=AXIS2_PLACEMENT_3D('',#86960,#57740,#57741);
#48246=AXIS2_PLACEMENT_3D('',#86961,#57742,#57743);
#48247=AXIS2_PLACEMENT_3D('',#86964,#57744,#57745);
#48248=AXIS2_PLACEMENT_3D('',#86968,#57747,#57748);
#48249=AXIS2_PLACEMENT_3D('',#87022,#57750,#57751);
#48250=AXIS2_PLACEMENT_3D('',#87084,#57753,#57754);
#48251=AXIS2_PLACEMENT_3D('',#87085,#57755,#57756);
#48252=AXIS2_PLACEMENT_3D('',#87086,#57757,#57758);
#48253=AXIS2_PLACEMENT_3D('',#87089,#57759,#57760);
#48254=AXIS2_PLACEMENT_3D('',#87093,#57762,#57763);
#48255=AXIS2_PLACEMENT_3D('',#87095,#57765,#57766);
#48256=AXIS2_PLACEMENT_3D('',#87097,#57767,#57768);
#48257=AXIS2_PLACEMENT_3D('',#87099,#57769,#57770);
#48258=AXIS2_PLACEMENT_3D('',#87100,#57771,#57772);
#48259=AXIS2_PLACEMENT_3D('',#87101,#57773,#57774);
#48260=AXIS2_PLACEMENT_3D('',#87147,#57775,#57776);
#48261=AXIS2_PLACEMENT_3D('',#87194,#57777,#57778);
#48262=AXIS2_PLACEMENT_3D('',#87196,#57779,#57780);
#48263=AXIS2_PLACEMENT_3D('',#87198,#57781,#57782);
#48264=AXIS2_PLACEMENT_3D('',#87199,#57783,#57784);
#48265=AXIS2_PLACEMENT_3D('',#87200,#57785,#57786);
#48266=AXIS2_PLACEMENT_3D('',#87202,#57787,#57788);
#48267=AXIS2_PLACEMENT_3D('',#87203,#57789,#57790);
#48268=AXIS2_PLACEMENT_3D('',#87204,#57791,#57792);
#48269=AXIS2_PLACEMENT_3D('',#87206,#57793,#57794);
#48270=AXIS2_PLACEMENT_3D('',#87210,#57796,#57797);
#48271=AXIS2_PLACEMENT_3D('',#87273,#57799,#57800);
#48272=AXIS2_PLACEMENT_3D('',#87332,#57802,#57803);
#48273=AXIS2_PLACEMENT_3D('',#87333,#57804,#57805);
#48274=AXIS2_PLACEMENT_3D('',#87385,#57806,#57807);
#48275=AXIS2_PLACEMENT_3D('',#87429,#57808,#57809);
#48276=AXIS2_PLACEMENT_3D('',#87432,#57810,#57811);
#48277=AXIS2_PLACEMENT_3D('',#87603,#57812,#57813);
#48278=AXIS2_PLACEMENT_3D('',#87609,#57817,#57818);
#48279=AXIS2_PLACEMENT_3D('',#87614,#57820,#57821);
#48280=AXIS2_PLACEMENT_3D('',#87617,#57823,#57824);
#48281=AXIS2_PLACEMENT_3D('',#88054,#57826,#57827);
#48282=AXIS2_PLACEMENT_3D('',#88059,#57829,#57830);
#48283=AXIS2_PLACEMENT_3D('',#88062,#57832,#57833);
#48284=AXIS2_PLACEMENT_3D('',#88496,#57834,#57835);
#48285=AXIS2_PLACEMENT_3D('',#88505,#57840,#57841);
#48286=AXIS2_PLACEMENT_3D('',#88511,#57845,#57846);
#48287=AXIS2_PLACEMENT_3D('',#88826,#57850,#57851);
#48288=AXIS2_PLACEMENT_3D('',#88827,#57852,#57853);
#48289=AXIS2_PLACEMENT_3D('',#89265,#57854,#57855);
#48290=AXIS2_PLACEMENT_3D('',#89266,#57856,#57857);
#48291=AXIS2_PLACEMENT_3D('',#89268,#57858,#57859);
#48292=AXIS2_PLACEMENT_3D('',#89269,#57860,#57861);
#48293=AXIS2_PLACEMENT_3D('',#89270,#57862,#57863);
#48294=AXIS2_PLACEMENT_3D('',#89272,#57864,#57865);
#48295=AXIS2_PLACEMENT_3D('',#89273,#57866,#57867);
#48296=AXIS2_PLACEMENT_3D('',#89274,#57868,#57869);
#48297=AXIS2_PLACEMENT_3D('',#89283,#57870,#57871);
#48298=AXIS2_PLACEMENT_3D('',#89285,#57873,#57874);
#48299=AXIS2_PLACEMENT_3D('',#89289,#57876,#57877);
#48300=AXIS2_PLACEMENT_3D('',#89298,#57878,#57879);
#48301=AXIS2_PLACEMENT_3D('',#89307,#57880,#57881);
#48302=AXIS2_PLACEMENT_3D('',#89309,#57882,#57883);
#48303=AXIS2_PLACEMENT_3D('',#89320,#57885,#57886);
#48304=AXIS2_PLACEMENT_3D('',#89327,#57887,#57888);
#48305=AXIS2_PLACEMENT_3D('',#89328,#57889,#57890);
#48306=AXIS2_PLACEMENT_3D('',#89335,#57891,#57892);
#48307=AXIS2_PLACEMENT_3D('',#89336,#57893,#57894);
#48308=AXIS2_PLACEMENT_3D('',#89337,#57895,#57896);
#48309=AXIS2_PLACEMENT_3D('',#89338,#57897,#57898);
#48310=AXIS2_PLACEMENT_3D('',#89339,#57899,#57900);
#48311=AXIS2_PLACEMENT_3D('',#89340,#57901,#57902);
#48312=AXIS2_PLACEMENT_3D('',#89341,#57903,#57904);
#48313=AXIS2_PLACEMENT_3D('',#89342,#57905,#57906);
#48314=AXIS2_PLACEMENT_3D('',#89343,#57907,#57908);
#48315=AXIS2_PLACEMENT_3D('',#89344,#57909,#57910);
#48316=AXIS2_PLACEMENT_3D('',#89345,#57911,#57912);
#48317=AXIS2_PLACEMENT_3D('',#89346,#57913,#57914);
#48318=AXIS2_PLACEMENT_3D('',#89347,#57915,#57916);
#48319=AXIS2_PLACEMENT_3D('',#89348,#57917,#57918);
#48320=AXIS2_PLACEMENT_3D('',#89349,#57919,#57920);
#48321=AXIS2_PLACEMENT_3D('',#89350,#57921,#57922);
#48322=AXIS2_PLACEMENT_3D('',#89351,#57923,#57924);
#48323=AXIS2_PLACEMENT_3D('',#89352,#57925,#57926);
#48324=AXIS2_PLACEMENT_3D('',#89353,#57927,#57928);
#48325=AXIS2_PLACEMENT_3D('',#89354,#57929,#57930);
#48326=AXIS2_PLACEMENT_3D('',#89523,#57931,#57932);
#48327=AXIS2_PLACEMENT_3D('',#89698,#57933,#57934);
#48328=AXIS2_PLACEMENT_3D('',#89701,#57935,#57936);
#48329=AXIS2_PLACEMENT_3D('',#89703,#57937,#57938);
#48330=AXIS2_PLACEMENT_3D('',#89705,#57939,#57940);
#48331=AXIS2_PLACEMENT_3D('',#89706,#57941,#57942);
#48332=AXIS2_PLACEMENT_3D('',#89707,#57943,#57944);
#48333=AXIS2_PLACEMENT_3D('',#89710,#57945,#57946);
#48334=AXIS2_PLACEMENT_3D('',#89713,#57949,#57950);
#48335=AXIS2_PLACEMENT_3D('',#89716,#57951,#57952);
#48336=AXIS2_PLACEMENT_3D('',#89719,#57955,#57956);
#48337=AXIS2_PLACEMENT_3D('',#89720,#57957,#57958);
#48338=AXIS2_PLACEMENT_3D('',#89721,#57959,#57960);
#48339=AXIS2_PLACEMENT_3D('',#89722,#57961,#57962);
#48340=AXIS2_PLACEMENT_3D('',#89724,#57963,#57964);
#48341=AXIS2_PLACEMENT_3D('',#89727,#57966,#57967);
#48342=AXIS2_PLACEMENT_3D('',#89765,#57968,#57969);
#48343=AXIS2_PLACEMENT_3D('',#89846,#57970,#57971);
#48344=AXIS2_PLACEMENT_3D('',#89902,#57972,#57973);
#48345=AXIS2_PLACEMENT_3D('',#89905,#57974,#57975);
#48346=AXIS2_PLACEMENT_3D('',#89908,#57978,#57979);
#48347=AXIS2_PLACEMENT_3D('',#89910,#57980,#57981);
#48348=AXIS2_PLACEMENT_3D('',#89911,#57982,#57983);
#48349=AXIS2_PLACEMENT_3D('',#89912,#57984,#57985);
#48350=AXIS2_PLACEMENT_3D('',#89915,#57986,#57987);
#48351=AXIS2_PLACEMENT_3D('',#89918,#57990,#57991);
#48352=AXIS2_PLACEMENT_3D('',#89921,#57992,#57993);
#48353=AXIS2_PLACEMENT_3D('',#89922,#57994,#57995);
#48354=AXIS2_PLACEMENT_3D('',#89923,#57996,#57997);
#48355=AXIS2_PLACEMENT_3D('',#89961,#57998,#57999);
#48356=AXIS2_PLACEMENT_3D('',#90104,#58000,#58001);
#48357=AXIS2_PLACEMENT_3D('',#90105,#58002,#58003);
#48358=AXIS2_PLACEMENT_3D('',#90106,#58004,#58005);
#48359=AXIS2_PLACEMENT_3D('',#90109,#58006,#58007);
#48360=AXIS2_PLACEMENT_3D('',#90110,#58008,#58009);
#48361=AXIS2_PLACEMENT_3D('',#90111,#58010,#58011);
#48362=AXIS2_PLACEMENT_3D('',#90112,#58012,#58013);
#48363=AXIS2_PLACEMENT_3D('',#90115,#58016,#58017);
#48364=AXIS2_PLACEMENT_3D('',#90117,#58019,#58020);
#48365=AXIS2_PLACEMENT_3D('',#90120,#58023,#58024);
#48366=AXIS2_PLACEMENT_3D('',#90121,#58025,#58026);
#48367=AXIS2_PLACEMENT_3D('',#90122,#58027,#58028);
#48368=AXIS2_PLACEMENT_3D('',#90125,#58031,#58032);
#48369=AXIS2_PLACEMENT_3D('',#90128,#58035,#58036);
#48370=AXIS2_PLACEMENT_3D('',#90129,#58037,#58038);
#48371=AXIS2_PLACEMENT_3D('',#90130,#58039,#58040);
#48372=AXIS2_PLACEMENT_3D('',#90131,#58041,#58042);
#48373=AXIS2_PLACEMENT_3D('',#90134,#58043,#58044);
#48374=AXIS2_PLACEMENT_3D('',#90137,#58047,#58048);
#48375=AXIS2_PLACEMENT_3D('',#90140,#58049,#58050);
#48376=AXIS2_PLACEMENT_3D('',#90141,#58051,#58052);
#48377=AXIS2_PLACEMENT_3D('',#90142,#58053,#58054);
#48378=AXIS2_PLACEMENT_3D('',#90143,#58055,#58056);
#48379=AXIS2_PLACEMENT_3D('',#90146,#58059,#58060);
#48380=AXIS2_PLACEMENT_3D('',#90148,#58061,#58062);
#48381=AXIS2_PLACEMENT_3D('',#90150,#58063,#58064);
#48382=AXIS2_PLACEMENT_3D('',#90151,#58065,#58066);
#48383=AXIS2_PLACEMENT_3D('',#90183,#58067,#58068);
#48384=AXIS2_PLACEMENT_3D('',#90258,#58069,#58070);
#48385=AXIS2_PLACEMENT_3D('',#90299,#58071,#58072);
#48386=AXIS2_PLACEMENT_3D('',#90301,#58073,#58074);
#48387=AXIS2_PLACEMENT_3D('',#90303,#58076,#58077);
#48388=AXIS2_PLACEMENT_3D('',#90306,#58078,#58079);
#48389=AXIS2_PLACEMENT_3D('',#90309,#58082,#58083);
#48390=AXIS2_PLACEMENT_3D('',#90312,#58084,#58085);
#48391=AXIS2_PLACEMENT_3D('',#90315,#58088,#58089);
#48392=AXIS2_PLACEMENT_3D('',#90317,#58090,#58091);
#48393=AXIS2_PLACEMENT_3D('',#90350,#58093,#58094);
#48394=AXIS2_PLACEMENT_3D('',#90391,#58095,#58096);
#48395=AXIS2_PLACEMENT_3D('',#90392,#58097,#58098);
#48396=AXIS2_PLACEMENT_3D('',#90393,#58099,#58100);
#48397=AXIS2_PLACEMENT_3D('',#90425,#58101,#58102);
#48398=AXIS2_PLACEMENT_3D('',#90481,#58103,#58104);
#48399=AXIS2_PLACEMENT_3D('',#90484,#58107,#58108);
#48400=AXIS2_PLACEMENT_3D('',#90487,#58111,#58112);
#48401=AXIS2_PLACEMENT_3D('',#90488,#58113,#58114);
#48402=AXIS2_PLACEMENT_3D('',#90489,#58115,#58116);
#48403=AXIS2_PLACEMENT_3D('',#90492,#58119,#58120);
#48404=AXIS2_PLACEMENT_3D('',#90493,#58121,#58122);
#48405=AXIS2_PLACEMENT_3D('',#90494,#58123,#58124);
#48406=AXIS2_PLACEMENT_3D('',#90495,#58125,#58126);
#48407=AXIS2_PLACEMENT_3D('',#90498,#58127,#58128);
#48408=AXIS2_PLACEMENT_3D('',#90501,#58131,#58132);
#48409=AXIS2_PLACEMENT_3D('',#90504,#58133,#58134);
#48410=AXIS2_PLACEMENT_3D('',#90505,#58135,#58136);
#48411=AXIS2_PLACEMENT_3D('',#90506,#58137,#58138);
#48412=AXIS2_PLACEMENT_3D('',#90507,#58139,#58140);
#48413=AXIS2_PLACEMENT_3D('',#90510,#58143,#58144);
#48414=AXIS2_PLACEMENT_3D('',#90512,#58145,#58146);
#48415=AXIS2_PLACEMENT_3D('',#90514,#58147,#58148);
#48416=AXIS2_PLACEMENT_3D('',#90515,#58149,#58150);
#48417=AXIS2_PLACEMENT_3D('',#90547,#58151,#58152);
#48418=AXIS2_PLACEMENT_3D('',#90622,#58153,#58154);
#48419=AXIS2_PLACEMENT_3D('',#90663,#58155,#58156);
#48420=AXIS2_PLACEMENT_3D('',#90665,#58157,#58158);
#48421=AXIS2_PLACEMENT_3D('',#90667,#58160,#58161);
#48422=AXIS2_PLACEMENT_3D('',#90670,#58162,#58163);
#48423=AXIS2_PLACEMENT_3D('',#90673,#58166,#58167);
#48424=AXIS2_PLACEMENT_3D('',#90676,#58168,#58169);
#48425=AXIS2_PLACEMENT_3D('',#90679,#58172,#58173);
#48426=AXIS2_PLACEMENT_3D('',#90681,#58174,#58175);
#48427=AXIS2_PLACEMENT_3D('',#90714,#58177,#58178);
#48428=AXIS2_PLACEMENT_3D('',#90755,#58179,#58180);
#48429=AXIS2_PLACEMENT_3D('',#90756,#58181,#58182);
#48430=AXIS2_PLACEMENT_3D('',#90757,#58183,#58184);
#48431=AXIS2_PLACEMENT_3D('',#90789,#58185,#58186);
#48432=AXIS2_PLACEMENT_3D('',#90845,#58187,#58188);
#48433=AXIS2_PLACEMENT_3D('',#90848,#58191,#58192);
#48434=AXIS2_PLACEMENT_3D('',#90851,#58195,#58196);
#48435=AXIS2_PLACEMENT_3D('',#90852,#58197,#58198);
#48436=AXIS2_PLACEMENT_3D('',#90853,#58199,#58200);
#48437=AXIS2_PLACEMENT_3D('',#90856,#58203,#58204);
#48438=AXIS2_PLACEMENT_3D('',#90857,#58205,#58206);
#48439=AXIS2_PLACEMENT_3D('',#90858,#58207,#58208);
#48440=AXIS2_PLACEMENT_3D('',#90859,#58209,#58210);
#48441=AXIS2_PLACEMENT_3D('',#90862,#58211,#58212);
#48442=AXIS2_PLACEMENT_3D('',#90865,#58215,#58216);
#48443=AXIS2_PLACEMENT_3D('',#90868,#58217,#58218);
#48444=AXIS2_PLACEMENT_3D('',#90869,#58219,#58220);
#48445=AXIS2_PLACEMENT_3D('',#90870,#58221,#58222);
#48446=AXIS2_PLACEMENT_3D('',#90871,#58223,#58224);
#48447=AXIS2_PLACEMENT_3D('',#90874,#58227,#58228);
#48448=AXIS2_PLACEMENT_3D('',#90876,#58229,#58230);
#48449=AXIS2_PLACEMENT_3D('',#90878,#58231,#58232);
#48450=AXIS2_PLACEMENT_3D('',#90879,#58233,#58234);
#48451=AXIS2_PLACEMENT_3D('',#90911,#58235,#58236);
#48452=AXIS2_PLACEMENT_3D('',#90986,#58237,#58238);
#48453=AXIS2_PLACEMENT_3D('',#91027,#58239,#58240);
#48454=AXIS2_PLACEMENT_3D('',#91029,#58241,#58242);
#48455=AXIS2_PLACEMENT_3D('',#91031,#58244,#58245);
#48456=AXIS2_PLACEMENT_3D('',#91034,#58246,#58247);
#48457=AXIS2_PLACEMENT_3D('',#91037,#58250,#58251);
#48458=AXIS2_PLACEMENT_3D('',#91040,#58252,#58253);
#48459=AXIS2_PLACEMENT_3D('',#91043,#58256,#58257);
#48460=AXIS2_PLACEMENT_3D('',#91045,#58258,#58259);
#48461=AXIS2_PLACEMENT_3D('',#91078,#58261,#58262);
#48462=AXIS2_PLACEMENT_3D('',#91119,#58263,#58264);
#48463=AXIS2_PLACEMENT_3D('',#91120,#58265,#58266);
#48464=AXIS2_PLACEMENT_3D('',#91121,#58267,#58268);
#48465=AXIS2_PLACEMENT_3D('',#91153,#58269,#58270);
#48466=AXIS2_PLACEMENT_3D('',#91209,#58271,#58272);
#48467=AXIS2_PLACEMENT_3D('',#91212,#58275,#58276);
#48468=AXIS2_PLACEMENT_3D('',#91215,#58279,#58280);
#48469=AXIS2_PLACEMENT_3D('',#91216,#58281,#58282);
#48470=AXIS2_PLACEMENT_3D('',#91217,#58283,#58284);
#48471=AXIS2_PLACEMENT_3D('',#91220,#58287,#58288);
#48472=AXIS2_PLACEMENT_3D('',#91221,#58289,#58290);
#48473=AXIS2_PLACEMENT_3D('',#91222,#58291,#58292);
#48474=AXIS2_PLACEMENT_3D('',#91223,#58293,#58294);
#48475=AXIS2_PLACEMENT_3D('',#91225,#58296,#58297);
#48476=AXIS2_PLACEMENT_3D('',#91227,#58299,#58300);
#48477=AXIS2_PLACEMENT_3D('',#91229,#58302,#58303);
#48478=AXIS2_PLACEMENT_3D('',#91231,#58304,#58305);
#48479=AXIS2_PLACEMENT_3D('',#91233,#58306,#58307);
#48480=AXIS2_PLACEMENT_3D('',#91235,#58309,#58310);
#48481=AXIS2_PLACEMENT_3D('',#91237,#58311,#58312);
#48482=AXIS2_PLACEMENT_3D('',#91238,#58313,#58314);
#48483=AXIS2_PLACEMENT_3D('',#91249,#58315,#58316);
#48484=AXIS2_PLACEMENT_3D('',#91250,#58317,#58318);
#48485=AXIS2_PLACEMENT_3D('',#91390,#58319,#58320);
#48486=AXIS2_PLACEMENT_3D('',#91395,#58321,#58322);
#48487=AXIS2_PLACEMENT_3D('',#91397,#58323,#58324);
#48488=AXIS2_PLACEMENT_3D('',#91418,#58326,#58327);
#48489=AXIS2_PLACEMENT_3D('',#91442,#58328,#58329);
#48490=AXIS2_PLACEMENT_3D('',#91443,#58330,#58331);
#48491=AXIS2_PLACEMENT_3D('',#91463,#58332,#58333);
#48492=AXIS2_PLACEMENT_3D('',#91470,#58334,#58335);
#48493=AXIS2_PLACEMENT_3D('',#91472,#58336,#58337);
#48494=AXIS2_PLACEMENT_3D('',#91493,#58339,#58340);
#48495=AXIS2_PLACEMENT_3D('',#91507,#58341,#58342);
#48496=AXIS2_PLACEMENT_3D('',#91509,#58343,#58344);
#48497=AXIS2_PLACEMENT_3D('',#91510,#58345,#58346);
#48498=AXIS2_PLACEMENT_3D('',#91554,#58347,#58348);
#48499=AXIS2_PLACEMENT_3D('',#91959,#58349,#58350);
#48500=AXIS2_PLACEMENT_3D('',#91964,#58353,#58354);
#48501=AXIS2_PLACEMENT_3D('',#92093,#58355,#58356);
#48502=AXIS2_PLACEMENT_3D('',#92446,#58357,#58358);
#48503=AXIS2_PLACEMENT_3D('',#92524,#58359,#58360);
#48504=AXIS2_PLACEMENT_3D('',#92526,#58361,#58362);
#48505=AXIS2_PLACEMENT_3D('',#92527,#58363,#58364);
#48506=AXIS2_PLACEMENT_3D('',#92528,#58365,#58366);
#48507=AXIS2_PLACEMENT_3D('',#92529,#58367,#58368);
#48508=AXIS2_PLACEMENT_3D('',#92531,#58369,#58370);
#48509=AXIS2_PLACEMENT_3D('',#92532,#58371,#58372);
#48510=AXIS2_PLACEMENT_3D('',#92533,#58373,#58374);
#48511=AXIS2_PLACEMENT_3D('',#92535,#58375,#58376);
#48512=AXIS2_PLACEMENT_3D('',#92537,#58378,#58379);
#48513=AXIS2_PLACEMENT_3D('',#92540,#58380,#58381);
#48514=AXIS2_PLACEMENT_3D('',#92541,#58382,#58383);
#48515=AXIS2_PLACEMENT_3D('',#92542,#58384,#58385);
#48516=AXIS2_PLACEMENT_3D('',#92586,#58386,#58387);
#48517=AXIS2_PLACEMENT_3D('',#92749,#58388,#58389);
#48518=AXIS2_PLACEMENT_3D('',#92872,#58390,#58391);
#48519=AXIS2_PLACEMENT_3D('',#92874,#58392,#58393);
#48520=AXIS2_PLACEMENT_3D('',#92876,#58395,#58396);
#48521=AXIS2_PLACEMENT_3D('',#92878,#58397,#58398);
#48522=AXIS2_PLACEMENT_3D('',#92879,#58399,#58400);
#48523=AXIS2_PLACEMENT_3D('',#92880,#58401,#58402);
#48524=AXIS2_PLACEMENT_3D('',#92920,#58405,#58406);
#48525=AXIS2_PLACEMENT_3D('',#92994,#58407,#58408);
#48526=AXIS2_PLACEMENT_3D('',#92996,#58409,#58410);
#48527=AXIS2_PLACEMENT_3D('',#92997,#58411,#58412);
#48528=AXIS2_PLACEMENT_3D('',#92998,#58413,#58414);
#48529=AXIS2_PLACEMENT_3D('',#93000,#58415,#58416);
#48530=AXIS2_PLACEMENT_3D('',#93001,#58417,#58418);
#48531=AXIS2_PLACEMENT_3D('',#93002,#58419,#58420);
#48532=AXIS2_PLACEMENT_3D('',#93004,#58421,#58422);
#48533=AXIS2_PLACEMENT_3D('',#93006,#58424,#58425);
#48534=AXIS2_PLACEMENT_3D('',#93008,#58426,#58427);
#48535=AXIS2_PLACEMENT_3D('',#93009,#58428,#58429);
#48536=AXIS2_PLACEMENT_3D('',#93053,#58430,#58431);
#48537=AXIS2_PLACEMENT_3D('',#93091,#58432,#58433);
#48538=AXIS2_PLACEMENT_3D('',#93093,#58434,#58435);
#48539=AXIS2_PLACEMENT_3D('',#93108,#58437,#58438);
#48540=AXIS2_PLACEMENT_3D('',#93141,#58439,#58440);
#48541=AXIS2_PLACEMENT_3D('',#93272,#58441,#58442);
#48542=AXIS2_PLACEMENT_3D('',#93395,#58443,#58444);
#48543=AXIS2_PLACEMENT_3D('',#93445,#58445,#58446);
#48544=AXIS2_PLACEMENT_3D('',#93591,#58447,#58448);
#48545=AXIS2_PLACEMENT_3D('',#93750,#58449,#58450);
#48546=AXIS2_PLACEMENT_3D('',#93967,#58451,#58452);
#48547=AXIS2_PLACEMENT_3D('',#94187,#58453,#58454);
#48548=AXIS2_PLACEMENT_3D('',#94371,#58455,#58456);
#48549=AXIS2_PLACEMENT_3D('',#94372,#58457,#58458);
#48550=AXIS2_PLACEMENT_3D('',#94373,#58459,#58460);
#48551=AXIS2_PLACEMENT_3D('',#94424,#58461,#58462);
#48552=AXIS2_PLACEMENT_3D('',#94509,#58463,#58464);
#48553=AXIS2_PLACEMENT_3D('',#94669,#58465,#58466);
#48554=AXIS2_PLACEMENT_3D('',#94760,#58467,#58468);
#48555=AXIS2_PLACEMENT_3D('',#94761,#58469,#58470);
#48556=AXIS2_PLACEMENT_3D('',#94762,#58471,#58472);
#48557=AXIS2_PLACEMENT_3D('',#94831,#58473,#58474);
#48558=AXIS2_PLACEMENT_3D('',#94867,#58479,#58480);
#48559=AXIS2_PLACEMENT_3D('',#94872,#58483,#58484);
#48560=AXIS2_PLACEMENT_3D('',#95222,#58485,#58486);
#48561=AXIS2_PLACEMENT_3D('',#96545,#58487,#58488);
#48562=AXIS2_PLACEMENT_3D('',#96546,#58489,#58490);
#48563=AXIS2_PLACEMENT_3D('',#96566,#58494,#58495);
#48564=AXIS2_PLACEMENT_3D('',#96567,#58496,#58497);
#48565=AXIS2_PLACEMENT_3D('',#96569,#58499,#58500);
#48566=AXIS2_PLACEMENT_3D('',#96748,#58503,#58504);
#48567=AXIS2_PLACEMENT_3D('',#96799,#58507,#58508);
#48568=AXIS2_PLACEMENT_3D('',#96800,#58509,#58510);
#48569=AXIS2_PLACEMENT_3D('',#96917,#58511,#58512);
#48570=AXIS2_PLACEMENT_3D('',#96919,#58514,#58515);
#48571=AXIS2_PLACEMENT_3D('',#96921,#58517,#58518);
#48572=AXIS2_PLACEMENT_3D('',#96923,#58520,#58521);
#48573=AXIS2_PLACEMENT_3D('',#96925,#58523,#58524);
#57537=DIRECTION('axis',(0.,0.,1.));
#57538=DIRECTION('refdir',(1.,0.,0.));
#57539=DIRECTION('center_axis',(0.,1.,0.));
#57540=DIRECTION('ref_axis',(0.,0.,1.));
#57541=DIRECTION('',(0.,1.,0.));
#57542=DIRECTION('center_axis',(0.,1.,0.));
#57543=DIRECTION('ref_axis',(0.,0.,1.));
#57544=DIRECTION('',(0.,1.,0.));
#57545=DIRECTION('center_axis',(0.,1.,0.));
#57546=DIRECTION('ref_axis',(0.,0.,-1.));
#57547=DIRECTION('center_axis',(-3.75424127281594E-15,0.,1.));
#57548=DIRECTION('ref_axis',(1.,0.,3.75424127281594E-15));
#57549=DIRECTION('',(0.,1.,0.));
#57550=DIRECTION('',(1.,0.,3.75424127281594E-15));
#57551=DIRECTION('',(1.,0.,3.75424127281594E-15));
#57552=DIRECTION('center_axis',(0.,1.,0.));
#57553=DIRECTION('ref_axis',(0.,0.,1.));
#57554=DIRECTION('',(0.,1.,0.));
#57555=DIRECTION('center_axis',(0.,1.,0.));
#57556=DIRECTION('ref_axis',(0.,0.,1.));
#57557=DIRECTION('center_axis',(0.,1.,0.));
#57558=DIRECTION('ref_axis',(0.,0.,-1.));
#57559=DIRECTION('center_axis',(-3.75424127281594E-15,0.,-1.));
#57560=DIRECTION('ref_axis',(-1.,0.,3.75424127281594E-15));
#57561=DIRECTION('',(-1.,0.,3.75424127281594E-15));
#57562=DIRECTION('',(-1.,0.,3.75424127281594E-15));
#57563=DIRECTION('center_axis',(0.,-1.,0.));
#57564=DIRECTION('ref_axis',(0.,0.,-1.));
#57565=DIRECTION('center_axis',(0.,1.,0.));
#57566=DIRECTION('ref_axis',(0.,0.,1.));
#57567=DIRECTION('center_axis',(0.,1.,0.));
#57568=DIRECTION('ref_axis',(0.,0.,1.));
#57569=DIRECTION('center_axis',(0.,1.,0.));
#57570=DIRECTION('ref_axis',(0.,0.,1.));
#57571=DIRECTION('',(1.,0.,-3.75424127281594E-15));
#57572=DIRECTION('center_axis',(0.,1.,0.));
#57573=DIRECTION('ref_axis',(0.,0.,1.));
#57574=DIRECTION('',(-1.,0.,-3.75424127281594E-15));
#57575=DIRECTION('center_axis',(3.75424127281594E-15,0.,1.));
#57576=DIRECTION('ref_axis',(1.,0.,-3.75424127281594E-15));
#57577=DIRECTION('',(0.,1.,0.));
#57578=DIRECTION('',(1.,0.,-3.75424127281594E-15));
#57579=DIRECTION('',(0.,1.,0.));
#57580=DIRECTION('center_axis',(0.,1.,0.));
#57581=DIRECTION('ref_axis',(0.,0.,1.));
#57582=DIRECTION('center_axis',(0.,1.,0.));
#57583=DIRECTION('ref_axis',(0.,0.,1.));
#57584=DIRECTION('',(0.,1.,0.));
#57585=DIRECTION('center_axis',(3.75424127281594E-15,0.,-1.));
#57586=DIRECTION('ref_axis',(-1.,0.,-3.75424127281594E-15));
#57587=DIRECTION('',(-1.,0.,-3.75424127281594E-15));
#57588=DIRECTION('',(0.,1.,0.));
#57589=DIRECTION('center_axis',(0.,1.,0.));
#57590=DIRECTION('ref_axis',(0.,0.,1.));
#57591=DIRECTION('center_axis',(0.,1.,0.));
#57592=DIRECTION('ref_axis',(0.,0.,1.));
#57593=DIRECTION('center_axis',(0.,1.,0.));
#57594=DIRECTION('ref_axis',(0.,0.,1.));
#57595=DIRECTION('center_axis',(0.,0.,-1.));
#57596=DIRECTION('ref_axis',(-1.,0.,0.));
#57597=DIRECTION('',(0.,0.,-1.));
#57598=DIRECTION('center_axis',(0.,0.,1.));
#57599=DIRECTION('ref_axis',(-1.,0.,0.));
#57600=DIRECTION('',(0.,0.,-1.));
#57601=DIRECTION('center_axis',(0.,0.,1.));
#57602=DIRECTION('ref_axis',(-1.,0.,0.));
#57603=DIRECTION('',(0.,0.,1.));
#57604=DIRECTION('center_axis',(0.,0.,1.));
#57605=DIRECTION('ref_axis',(-1.,-2.6760472293316E-15,0.));
#57606=DIRECTION('',(0.,0.,1.));
#57607=DIRECTION('center_axis',(-0.674290861195454,-0.353082477337477,0.648586616193645));
#57608=DIRECTION('ref_axis',(0.738465865105631,-0.322427194837445,0.592206779852315));
#57609=DIRECTION('',(0.,0.,1.));
#57610=DIRECTION('center_axis',(0.,0.,-1.));
#57611=DIRECTION('ref_axis',(-1.,0.,0.));
#57612=DIRECTION('center_axis',(0.997947005577613,-0.0140531647494822,0.0624842589713604));
#57613=DIRECTION('ref_axis',(-0.0640450849043188,-0.219494029111198,0.973509423829133));
#57614=DIRECTION('center_axis',(0.,0.,-1.));
#57615=DIRECTION('ref_axis',(-1.,0.,0.));
#57616=DIRECTION('center_axis',(-1.55697293342929E-16,-1.,0.));
#57617=DIRECTION('ref_axis',(1.,-1.55697293342929E-16,0.));
#57618=DIRECTION('center_axis',(0.,0.,1.));
#57619=DIRECTION('ref_axis',(-1.,0.,0.));
#57620=DIRECTION('center_axis',(0.,0.,-1.));
#57621=DIRECTION('ref_axis',(-6.12323399573677E-17,1.,0.));
#57622=DIRECTION('center_axis',(0.,0.,1.));
#57623=DIRECTION('ref_axis',(1.,0.,0.));
#57624=DIRECTION('',(0.,0.,-1.));
#57625=DIRECTION('center_axis',(0.,0.,1.));
#57626=DIRECTION('ref_axis',(1.,0.,0.));
#57627=DIRECTION('',(0.,0.,1.));
#57628=DIRECTION('center_axis',(0.,0.,-1.));
#57629=DIRECTION('ref_axis',(-2.83276944882399E-16,1.,0.));
#57630=DIRECTION('center_axis',(0.,0.,1.));
#57631=DIRECTION('ref_axis',(1.,0.,0.));
#57632=DIRECTION('',(0.,0.,-1.));
#57633=DIRECTION('center_axis',(0.,0.,1.));
#57634=DIRECTION('ref_axis',(1.,0.,0.));
#57635=DIRECTION('',(0.,0.,1.));
#57636=DIRECTION('center_axis',(0.,0.,-1.));
#57637=DIRECTION('ref_axis',(-6.12323399573677E-17,1.,0.));
#57638=DIRECTION('center_axis',(0.,0.,1.));
#57639=DIRECTION('ref_axis',(1.,0.,0.));
#57640=DIRECTION('',(0.,0.,-1.));
#57641=DIRECTION('center_axis',(0.,0.,1.));
#57642=DIRECTION('ref_axis',(1.,0.,0.));
#57643=DIRECTION('',(0.,0.,1.));
#57644=DIRECTION('center_axis',(0.,0.,-1.));
#57645=DIRECTION('ref_axis',(-1.,0.,0.));
#57646=DIRECTION('center_axis',(0.,0.,1.));
#57647=DIRECTION('ref_axis',(1.,0.,0.));
#57648=DIRECTION('',(0.,0.,1.));
#57649=DIRECTION('center_axis',(0.,0.,-1.));
#57650=DIRECTION('ref_axis',(1.,0.,0.));
#57651=DIRECTION('',(0.,0.,-1.));
#57652=DIRECTION('center_axis',(0.,0.,-1.));
#57653=DIRECTION('ref_axis',(1.,-1.73472347597681E-15,0.));
#57654=DIRECTION('',(0.,0.,1.));
#57655=DIRECTION('center_axis',(0.,0.,-1.));
#57656=DIRECTION('ref_axis',(1.,0.,0.));
#57657=DIRECTION('center_axis',(0.,0.,1.));
#57658=DIRECTION('ref_axis',(1.,0.,0.));
#57659=DIRECTION('center_axis',(0.,0.,1.));
#57660=DIRECTION('ref_axis',(1.,0.,0.));
#57661=DIRECTION('center_axis',(0.,0.,1.));
#57662=DIRECTION('ref_axis',(1.,0.,0.));
#57663=DIRECTION('',(0.,0.,1.));
#57664=DIRECTION('center_axis',(0.,0.,-1.));
#57665=DIRECTION('ref_axis',(1.,0.,0.));
#57666=DIRECTION('',(0.,0.,1.));
#57667=DIRECTION('center_axis',(0.,0.,1.));
#57668=DIRECTION('ref_axis',(1.,0.,0.));
#57669=DIRECTION('center_axis',(0.710660584319699,0.703535026771507,0.));
#57670=DIRECTION('ref_axis',(-0.703535026771507,0.710660584319699,0.));
#57671=DIRECTION('center_axis',(0.,0.,-1.));
#57672=DIRECTION('ref_axis',(1.,-7.7650619940415E-16,0.));
#57673=DIRECTION('center_axis',(0.710660584319702,0.703535026771503,-4.88175490844999E-15));
#57674=DIRECTION('ref_axis',(-0.703535026771503,0.710660584319702,-2.41028291557853E-29));
#57675=DIRECTION('center_axis',(0.,0.,1.));
#57676=DIRECTION('ref_axis',(0.710660584319704,0.703535026771501,0.));
#57677=DIRECTION('center_axis',(0.,0.,1.));
#57678=DIRECTION('ref_axis',(1.,0.,0.));
#57679=DIRECTION('center_axis',(0.,0.,1.));
#57680=DIRECTION('ref_axis',(1.,0.,0.));
#57681=DIRECTION('center_axis',(0.710660584319702,0.703535026771503,4.88175490844999E-15));
#57682=DIRECTION('ref_axis',(-0.703535026771503,0.710660584319702,2.41028291557853E-29));
#57683=DIRECTION('center_axis',(0.,0.,1.));
#57684=DIRECTION('ref_axis',(1.,0.,0.));
#57685=DIRECTION('center_axis',(-0.710660584319702,-0.703535026771503,0.));
#57686=DIRECTION('ref_axis',(0.703535026771503,-0.710660584319702,0.));
#57687=DIRECTION('center_axis',(0.,0.,1.));
#57688=DIRECTION('ref_axis',(1.,0.,0.));
#57689=DIRECTION('center_axis',(0.,-1.,0.));
#57690=DIRECTION('ref_axis',(-1.,0.,0.));
#57691=DIRECTION('center_axis',(0.,0.,1.));
#57692=DIRECTION('ref_axis',(1.,0.,0.));
#57693=DIRECTION('center_axis',(0.,0.,-1.));
#57694=DIRECTION('ref_axis',(-1.,0.,0.));
#57695=DIRECTION('center_axis',(0.,0.,1.));
#57696=DIRECTION('ref_axis',(1.,0.,0.));
#57697=DIRECTION('',(0.,0.,1.));
#57698=DIRECTION('center_axis',(0.,0.,-1.));
#57699=DIRECTION('ref_axis',(1.,0.,0.));
#57700=DIRECTION('',(0.,0.,-1.));
#57701=DIRECTION('center_axis',(0.,0.,-1.));
#57702=DIRECTION('ref_axis',(1.,-1.73472347597681E-15,0.));
#57703=DIRECTION('',(0.,0.,1.));
#57704=DIRECTION('center_axis',(0.,0.,-1.));
#57705=DIRECTION('ref_axis',(1.,0.,0.));
#57706=DIRECTION('center_axis',(0.,0.,1.));
#57707=DIRECTION('ref_axis',(1.,0.,0.));
#57708=DIRECTION('center_axis',(0.,0.,1.));
#57709=DIRECTION('ref_axis',(1.,0.,0.));
#57710=DIRECTION('center_axis',(0.,0.,1.));
#57711=DIRECTION('ref_axis',(1.,0.,0.));
#57712=DIRECTION('',(0.,0.,1.));
#57713=DIRECTION('center_axis',(0.,0.,-1.));
#57714=DIRECTION('ref_axis',(1.,0.,0.));
#57715=DIRECTION('',(0.,0.,1.));
#57716=DIRECTION('center_axis',(0.,0.,1.));
#57717=DIRECTION('ref_axis',(1.,0.,0.));
#57718=DIRECTION('center_axis',(0.710660584319699,0.703535026771507,0.));
#57719=DIRECTION('ref_axis',(-0.703535026771507,0.710660584319699,0.));
#57720=DIRECTION('center_axis',(0.,0.,-1.));
#57721=DIRECTION('ref_axis',(1.,-2.32951859821245E-15,0.));
#57722=DIRECTION('center_axis',(0.710660584319702,0.703535026771503,-4.88175490844999E-15));
#57723=DIRECTION('ref_axis',(-0.703535026771503,0.710660584319702,-2.41028291557853E-29));
#57724=DIRECTION('center_axis',(0.,0.,1.));
#57725=DIRECTION('ref_axis',(0.710660584319704,0.703535026771501,0.));
#57726=DIRECTION('center_axis',(0.,0.,1.));
#57727=DIRECTION('ref_axis',(1.,0.,0.));
#57728=DIRECTION('center_axis',(0.,0.,1.));
#57729=DIRECTION('ref_axis',(1.,0.,0.));
#57730=DIRECTION('center_axis',(0.710660584319702,0.703535026771503,4.88175490844999E-15));
#57731=DIRECTION('ref_axis',(-0.703535026771503,0.710660584319702,2.41028291557853E-29));
#57732=DIRECTION('center_axis',(0.,0.,1.));
#57733=DIRECTION('ref_axis',(1.,0.,0.));
#57734=DIRECTION('center_axis',(-0.710660584319702,-0.703535026771503,0.));
#57735=DIRECTION('ref_axis',(0.703535026771503,-0.710660584319702,0.));
#57736=DIRECTION('center_axis',(0.,0.,1.));
#57737=DIRECTION('ref_axis',(1.,0.,0.));
#57738=DIRECTION('center_axis',(0.,-1.,0.));
#57739=DIRECTION('ref_axis',(-1.,0.,0.));
#57740=DIRECTION('center_axis',(0.,0.,1.));
#57741=DIRECTION('ref_axis',(1.,0.,0.));
#57742=DIRECTION('center_axis',(0.,0.,-1.));
#57743=DIRECTION('ref_axis',(-1.,0.,0.));
#57744=DIRECTION('center_axis',(0.,0.,1.));
#57745=DIRECTION('ref_axis',(1.,0.,0.));
#57746=DIRECTION('',(0.,0.,1.));
#57747=DIRECTION('center_axis',(0.,0.,-1.));
#57748=DIRECTION('ref_axis',(1.,0.,0.));
#57749=DIRECTION('',(0.,0.,-1.));
#57750=DIRECTION('center_axis',(0.,0.,-1.));
#57751=DIRECTION('ref_axis',(1.,0.,0.));
#57752=DIRECTION('',(0.,0.,1.));
#57753=DIRECTION('center_axis',(0.,0.,-1.));
#57754=DIRECTION('ref_axis',(1.,0.,0.));
#57755=DIRECTION('center_axis',(0.,0.,1.));
#57756=DIRECTION('ref_axis',(1.,0.,0.));
#57757=DIRECTION('center_axis',(0.,0.,1.));
#57758=DIRECTION('ref_axis',(1.,0.,0.));
#57759=DIRECTION('center_axis',(0.,0.,1.));
#57760=DIRECTION('ref_axis',(1.,0.,0.));
#57761=DIRECTION('',(0.,0.,1.));
#57762=DIRECTION('center_axis',(0.,0.,-1.));
#57763=DIRECTION('ref_axis',(1.,0.,0.));
#57764=DIRECTION('',(0.,0.,1.));
#57765=DIRECTION('center_axis',(0.,0.,1.));
#57766=DIRECTION('ref_axis',(1.,0.,0.));
#57767=DIRECTION('center_axis',(0.710660584319699,0.703535026771507,0.));
#57768=DIRECTION('ref_axis',(-0.703535026771507,0.710660584319699,0.));
#57769=DIRECTION('center_axis',(0.,0.,-1.));
#57770=DIRECTION('ref_axis',(1.,-2.32951859821245E-15,0.));
#57771=DIRECTION('center_axis',(0.710660584319702,0.703535026771503,-4.88175490844999E-15));
#57772=DIRECTION('ref_axis',(-0.703535026771503,0.710660584319702,-2.41028291557853E-29));
#57773=DIRECTION('center_axis',(0.,0.,1.));
#57774=DIRECTION('ref_axis',(0.710660584319704,0.703535026771501,0.));
#57775=DIRECTION('center_axis',(0.,0.,1.));
#57776=DIRECTION('ref_axis',(1.,0.,0.));
#57777=DIRECTION('center_axis',(0.,0.,1.));
#57778=DIRECTION('ref_axis',(1.,0.,0.));
#57779=DIRECTION('center_axis',(0.710660584319702,0.703535026771503,4.88175490844999E-15));
#57780=DIRECTION('ref_axis',(-0.703535026771503,0.710660584319702,2.41028291557853E-29));
#57781=DIRECTION('center_axis',(0.,0.,1.));
#57782=DIRECTION('ref_axis',(1.,0.,0.));
#57783=DIRECTION('center_axis',(-0.710660584319702,-0.703535026771503,0.));
#57784=DIRECTION('ref_axis',(0.703535026771503,-0.710660584319702,0.));
#57785=DIRECTION('center_axis',(0.,0.,1.));
#57786=DIRECTION('ref_axis',(1.,0.,0.));
#57787=DIRECTION('center_axis',(0.,-1.,0.));
#57788=DIRECTION('ref_axis',(-1.,0.,0.));
#57789=DIRECTION('center_axis',(0.,0.,1.));
#57790=DIRECTION('ref_axis',(1.,0.,0.));
#57791=DIRECTION('center_axis',(0.,0.,-1.));
#57792=DIRECTION('ref_axis',(-1.,0.,0.));
#57793=DIRECTION('center_axis',(0.,0.,1.));
#57794=DIRECTION('ref_axis',(-1.,0.,0.));
#57795=DIRECTION('',(0.,0.,1.));
#57796=DIRECTION('center_axis',(0.,0.,-1.));
#57797=DIRECTION('ref_axis',(1.,-1.73321670543144E-15,0.));
#57798=DIRECTION('',(0.,0.,-1.));
#57799=DIRECTION('center_axis',(0.,0.,-1.));
#57800=DIRECTION('ref_axis',(1.,-3.59975777281914E-15,0.));
#57801=DIRECTION('',(0.,0.,1.));
#57802=DIRECTION('center_axis',(0.,0.,-1.));
#57803=DIRECTION('ref_axis',(1.,-1.73321670543144E-15,0.));
#57804=DIRECTION('center_axis',(0.,0.,1.));
#57805=DIRECTION('ref_axis',(0.,-1.,0.));
#57806=DIRECTION('center_axis',(0.,0.,1.));
#57807=DIRECTION('ref_axis',(1.,0.,0.));
#57808=DIRECTION('center_axis',(1.27486239704332E-16,-1.,0.));
#57809=DIRECTION('ref_axis',(1.,1.27486239704332E-16,0.));
#57810=DIRECTION('center_axis',(-1.27486239704332E-16,1.,0.));
#57811=DIRECTION('ref_axis',(1.,1.27486239704332E-16,0.));
#57812=DIRECTION('center_axis',(-1.27486239704332E-16,1.,0.));
#57813=DIRECTION('ref_axis',(1.,1.27486239704332E-16,-1.88173394004264E-13));
#57814=DIRECTION('',(0.,0.,-1.));
#57815=DIRECTION('',(-1.,-1.27486239704332E-16,0.));
#57816=DIRECTION('',(0.,0.,1.));
#57817=DIRECTION('center_axis',(-1.27486239704332E-16,1.,0.));
#57818=DIRECTION('ref_axis',(-1.,-1.27486239704332E-16,0.));
#57819=DIRECTION('',(1.27486239704332E-16,-1.,0.));
#57820=DIRECTION('center_axis',(1.27486239704332E-16,-1.,0.));
#57821=DIRECTION('ref_axis',(1.,1.27486239704332E-16,0.));
#57822=DIRECTION('',(0.,1.,0.));
#57823=DIRECTION('center_axis',(0.,1.,0.));
#57824=DIRECTION('ref_axis',(0.,0.,1.));
#57825=DIRECTION('',(-1.27486239704332E-16,1.,0.));
#57826=DIRECTION('center_axis',(-1.27486239704332E-16,1.,0.));
#57827=DIRECTION('ref_axis',(-1.,-1.27486239704332E-16,0.));
#57828=DIRECTION('',(0.,-1.,0.));
#57829=DIRECTION('center_axis',(1.27486239704332E-16,-1.,0.));
#57830=DIRECTION('ref_axis',(1.,1.27486239704332E-16,0.));
#57831=DIRECTION('',(-1.27486239704332E-16,1.,0.));
#57832=DIRECTION('center_axis',(0.,1.,0.));
#57833=DIRECTION('ref_axis',(0.,0.,1.));
#57834=DIRECTION('center_axis',(0.,0.,-1.));
#57835=DIRECTION('ref_axis',(-1.,0.,0.));
#57836=DIRECTION('',(-1.,0.,0.));
#57837=DIRECTION('',(0.,1.,0.));
#57838=DIRECTION('',(1.,1.27486239704332E-16,0.));
#57839=DIRECTION('',(0.,-1.,0.));
#57840=DIRECTION('center_axis',(1.,0.,0.));
#57841=DIRECTION('ref_axis',(0.,0.,-1.));
#57842=DIRECTION('',(0.,0.,-1.));
#57843=DIRECTION('',(0.,-1.,0.));
#57844=DIRECTION('',(0.,0.,1.));
#57845=DIRECTION('center_axis',(-1.,0.,0.));
#57846=DIRECTION('ref_axis',(0.,0.,1.));
#57847=DIRECTION('',(0.,1.,0.));
#57848=DIRECTION('',(0.,0.,1.));
#57849=DIRECTION('',(0.,0.,-1.));
#57850=DIRECTION('center_axis',(0.00367439112755605,0.,-0.999993249402136));
#57851=DIRECTION('ref_axis',(-0.999993249402136,0.,-0.00367439112755605));
#57852=DIRECTION('center_axis',(-1.,0.,-1.23259516440783E-29));
#57853=DIRECTION('ref_axis',(-1.23259516440783E-29,0.,1.));
#57854=DIRECTION('center_axis',(-0.0036743911275285,0.,-0.999993249402136));
#57855=DIRECTION('ref_axis',(-0.999993249402136,0.,0.0036743911275285));
#57856=DIRECTION('center_axis',(0.,1.,0.));
#57857=DIRECTION('ref_axis',(0.,0.,1.));
#57858=DIRECTION('center_axis',(0.,-1.,0.));
#57859=DIRECTION('ref_axis',(0.,0.,-1.));
#57860=DIRECTION('center_axis',(0.,0.,-1.));
#57861=DIRECTION('ref_axis',(-1.,0.,0.));
#57862=DIRECTION('center_axis',(0.,1.,0.));
#57863=DIRECTION('ref_axis',(0.,0.,1.));
#57864=DIRECTION('center_axis',(0.,-1.,0.));
#57865=DIRECTION('ref_axis',(0.,0.,-1.));
#57866=DIRECTION('center_axis',(0.,0.,-1.));
#57867=DIRECTION('ref_axis',(-1.,0.,0.));
#57868=DIRECTION('center_axis',(0.,0.,-1.));
#57869=DIRECTION('ref_axis',(-1.,0.,0.));
#57870=DIRECTION('center_axis',(0.,0.,-1.));
#57871=DIRECTION('ref_axis',(-1.,0.,0.));
#57872=DIRECTION('',(0.,0.,1.));
#57873=DIRECTION('center_axis',(0.,0.,1.));
#57874=DIRECTION('ref_axis',(1.,0.,0.));
#57875=DIRECTION('',(0.,0.,-1.));
#57876=DIRECTION('center_axis',(0.,0.,-1.));
#57877=DIRECTION('ref_axis',(-1.,0.,0.));
#57878=DIRECTION('center_axis',(-1.,0.,0.));
#57879=DIRECTION('ref_axis',(0.,0.,1.));
#57880=DIRECTION('center_axis',(-1.,0.,0.));
#57881=DIRECTION('ref_axis',(0.,0.,1.));
#57882=DIRECTION('center_axis',(1.,0.,0.));
#57883=DIRECTION('ref_axis',(0.,0.,-1.));
#57884=DIRECTION('',(1.,0.,0.));
#57885=DIRECTION('center_axis',(0.,1.,0.));
#57886=DIRECTION('ref_axis',(1.,0.,0.));
#57887=DIRECTION('center_axis',(0.,1.,0.));
#57888=DIRECTION('ref_axis',(0.,0.,-1.));
#57889=DIRECTION('center_axis',(0.,1.,0.));
#57890=DIRECTION('ref_axis',(1.,0.,0.));
#57891=DIRECTION('center_axis',(0.,1.,0.));
#57892=DIRECTION('ref_axis',(0.,0.,-1.));
#57893=DIRECTION('center_axis',(0.,-1.,0.));
#57894=DIRECTION('ref_axis',(0.,0.,-1.));
#57895=DIRECTION('center_axis',(0.,1.,0.));
#57896=DIRECTION('ref_axis',(0.,0.,1.));
#57897=DIRECTION('center_axis',(0.,1.,0.));
#57898=DIRECTION('ref_axis',(0.,0.,1.));
#57899=DIRECTION('center_axis',(0.,1.,0.));
#57900=DIRECTION('ref_axis',(0.,0.,1.));
#57901=DIRECTION('center_axis',(1.,1.27486239704332E-16,0.));
#57902=DIRECTION('ref_axis',(-1.27486239704332E-16,1.,0.));
#57903=DIRECTION('center_axis',(1.,0.,0.));
#57904=DIRECTION('ref_axis',(0.,0.,-1.));
#57905=DIRECTION('center_axis',(-1.,0.,0.));
#57906=DIRECTION('ref_axis',(0.,0.,1.));
#57907=DIRECTION('center_axis',(0.,1.,0.));
#57908=DIRECTION('ref_axis',(1.,0.,0.));
#57909=DIRECTION('center_axis',(0.,0.,1.));
#57910=DIRECTION('ref_axis',(-1.,0.,0.));
#57911=DIRECTION('center_axis',(0.,1.,0.));
#57912=DIRECTION('ref_axis',(1.,0.,0.));
#57913=DIRECTION('center_axis',(0.,0.,1.));
#57914=DIRECTION('ref_axis',(-1.,0.,0.));
#57915=DIRECTION('center_axis',(0.,0.,-1.));
#57916=DIRECTION('ref_axis',(-1.,0.,0.));
#57917=DIRECTION('center_axis',(0.,0.,1.));
#57918=DIRECTION('ref_axis',(1.,0.,0.));
#57919=DIRECTION('center_axis',(0.,0.,-1.));
#57920=DIRECTION('ref_axis',(-1.,0.,0.));
#57921=DIRECTION('center_axis',(0.,0.,1.));
#57922=DIRECTION('ref_axis',(1.,0.,0.));
#57923=DIRECTION('center_axis',(1.27486239704332E-16,-1.,0.));
#57924=DIRECTION('ref_axis',(1.,2.368475785867E-16,0.));
#57925=DIRECTION('center_axis',(-0.00367439112755605,2.03969681564559E-16,
0.999993249402136));
#57926=DIRECTION('ref_axis',(0.999993249402136,6.24671789190351E-35,0.00367439112755605));
#57927=DIRECTION('center_axis',(1.27486239704332E-16,-1.,0.));
#57928=DIRECTION('ref_axis',(1.,2.368475785867E-16,0.));
#57929=DIRECTION('center_axis',(0.0036743911275283,0.,0.999993249402136));
#57930=DIRECTION('ref_axis',(0.999993249402136,0.,-0.0036743911275283));
#57931=DIRECTION('center_axis',(-1.,1.56267011062633E-16,2.83753250766951E-16));
#57932=DIRECTION('ref_axis',(2.83753250766951E-16,1.09476442525376E-47,
1.));
#57933=DIRECTION('center_axis',(0.,0.,1.));
#57934=DIRECTION('ref_axis',(1.,0.,0.));
#57935=DIRECTION('center_axis',(0.,-1.,0.));
#57936=DIRECTION('ref_axis',(0.,0.,-1.));
#57937=DIRECTION('center_axis',(0.,0.,-1.));
#57938=DIRECTION('ref_axis',(1.,0.,0.));
#57939=DIRECTION('center_axis',(0.,-1.,0.));
#57940=DIRECTION('ref_axis',(0.,0.,-1.));
#57941=DIRECTION('center_axis',(0.,0.,1.));
#57942=DIRECTION('ref_axis',(1.,0.,0.));
#57943=DIRECTION('center_axis',(0.,1.,0.));
#57944=DIRECTION('ref_axis',(0.,0.,1.));
#57945=DIRECTION('center_axis',(0.,-1.,0.));
#57946=DIRECTION('ref_axis',(0.,0.,-1.));
#57947=DIRECTION('',(0.,1.,0.));
#57948=DIRECTION('',(0.,-1.,0.));
#57949=DIRECTION('center_axis',(0.,-1.,0.));
#57950=DIRECTION('ref_axis',(0.,0.,-1.));
#57951=DIRECTION('center_axis',(0.,-1.,0.));
#57952=DIRECTION('ref_axis',(0.,0.,-1.));
#57953=DIRECTION('',(0.,1.,0.));
#57954=DIRECTION('',(0.,-1.,0.));
#57955=DIRECTION('center_axis',(0.,0.,1.));
#57956=DIRECTION('ref_axis',(1.,0.,0.));
#57957=DIRECTION('center_axis',(0.,0.,-1.));
#57958=DIRECTION('ref_axis',(1.,0.,0.));
#57959=DIRECTION('center_axis',(0.,0.,1.));
#57960=DIRECTION('ref_axis',(1.,0.,0.));
#57961=DIRECTION('center_axis',(0.,0.,-1.));
#57962=DIRECTION('ref_axis',(-1.,0.,0.));
#57963=DIRECTION('center_axis',(0.,0.,1.));
#57964=DIRECTION('ref_axis',(-1.,9.91270557701024E-15,0.));
#57965=DIRECTION('',(0.,0.,1.));
#57966=DIRECTION('center_axis',(0.,0.,-1.));
#57967=DIRECTION('ref_axis',(1.,0.,0.));
#57968=DIRECTION('center_axis',(0.988416151653142,0.151767951660399,0.));
#57969=DIRECTION('ref_axis',(-0.151767951660399,0.988416151653142,0.));
#57970=DIRECTION('center_axis',(0.,-1.,0.));
#57971=DIRECTION('ref_axis',(0.,0.,-1.));
#57972=DIRECTION('center_axis',(0.,1.,0.));
#57973=DIRECTION('ref_axis',(0.,0.,1.));
#57974=DIRECTION('center_axis',(0.,-1.,0.));
#57975=DIRECTION('ref_axis',(0.,0.,-1.));
#57976=DIRECTION('',(0.,1.,0.));
#57977=DIRECTION('',(0.,-1.,0.));
#57978=DIRECTION('center_axis',(0.,0.,1.));
#57979=DIRECTION('ref_axis',(1.,0.,0.));
#57980=DIRECTION('center_axis',(0.988416151653139,-0.151767951660418,0.));
#57981=DIRECTION('ref_axis',(-0.151767951660418,-0.988416151653139,0.));
#57982=DIRECTION('center_axis',(0.,0.,1.));
#57983=DIRECTION('ref_axis',(1.,0.,0.));
#57984=DIRECTION('center_axis',(0.,1.,0.));
#57985=DIRECTION('ref_axis',(0.,0.,1.));
#57986=DIRECTION('center_axis',(0.,-1.,0.));
#57987=DIRECTION('ref_axis',(0.,0.,-1.));
#57988=DIRECTION('',(0.,-1.,0.));
#57989=DIRECTION('',(0.,1.,0.));
#57990=DIRECTION('center_axis',(0.,0.,1.));
#57991=DIRECTION('ref_axis',(1.,0.,0.));
#57992=DIRECTION('center_axis',(0.,1.,0.));
#57993=DIRECTION('ref_axis',(0.,0.,1.));
#57994=DIRECTION('center_axis',(0.,0.,-1.));
#57995=DIRECTION('ref_axis',(1.,0.,0.));
#57996=DIRECTION('center_axis',(0.,0.,1.));
#57997=DIRECTION('ref_axis',(1.,0.,0.));
#57998=DIRECTION('center_axis',(0.,0.,1.));
#57999=DIRECTION('ref_axis',(1.,0.,0.));
#58000=DIRECTION('center_axis',(0.,-1.,0.));
#58001=DIRECTION('ref_axis',(0.,0.,-1.));
#58002=DIRECTION('center_axis',(0.,0.,-1.));
#58003=DIRECTION('ref_axis',(-1.,0.,0.));
#58004=DIRECTION('center_axis',(0.,0.,1.));
#58005=DIRECTION('ref_axis',(1.,0.,0.));
#58006=DIRECTION('center_axis',(0.,1.,0.));
#58007=DIRECTION('ref_axis',(0.,0.,1.));
#58008=DIRECTION('center_axis',(0.,0.,1.));
#58009=DIRECTION('ref_axis',(1.,0.,0.));
#58010=DIRECTION('center_axis',(0.,0.,-1.));
#58011=DIRECTION('ref_axis',(1.,0.,0.));
#58012=DIRECTION('center_axis',(0.,-1.,0.));
#58013=DIRECTION('ref_axis',(0.,0.,-1.));
#58014=DIRECTION('',(0.,1.,0.));
#58015=DIRECTION('',(0.,-1.,0.));
#58016=DIRECTION('center_axis',(0.,0.,-1.));
#58017=DIRECTION('ref_axis',(-1.,0.,0.));
#58018=DIRECTION('',(0.,0.,-1.));
#58019=DIRECTION('center_axis',(0.,-1.,0.));
#58020=DIRECTION('ref_axis',(0.,0.,-1.));
#58021=DIRECTION('',(0.,1.,0.));
#58022=DIRECTION('',(0.,-1.,0.));
#58023=DIRECTION('center_axis',(0.,0.,1.));
#58024=DIRECTION('ref_axis',(1.,0.,0.));
#58025=DIRECTION('center_axis',(0.,0.,1.));
#58026=DIRECTION('ref_axis',(1.,0.,0.));
#58027=DIRECTION('center_axis',(0.,0.,1.));
#58028=DIRECTION('ref_axis',(1.,0.,0.));
#58029=DIRECTION('',(0.,0.,1.));
#58030=DIRECTION('',(0.,0.,1.));
#58031=DIRECTION('center_axis',(0.,0.,1.));
#58032=DIRECTION('ref_axis',(1.,0.,0.));
#58033=DIRECTION('',(0.,0.,1.));
#58034=DIRECTION('',(0.,0.,1.));
#58035=DIRECTION('center_axis',(1.,0.,0.));
#58036=DIRECTION('ref_axis',(0.,0.,-1.));
#58037=DIRECTION('center_axis',(-1.,0.,0.));
#58038=DIRECTION('ref_axis',(0.,0.,1.));
#58039=DIRECTION('center_axis',(0.,0.,1.));
#58040=DIRECTION('ref_axis',(1.,0.,0.));
#58041=DIRECTION('center_axis',(0.710660584319708,0.703535026771498,0.));
#58042=DIRECTION('ref_axis',(-0.703535026771498,0.710660584319708,0.));
#58043=DIRECTION('center_axis',(0.710660584319702,0.703535026771503,0.));
#58044=DIRECTION('ref_axis',(-0.703535026771503,0.710660584319702,0.));
#58045=DIRECTION('',(-0.710660584319708,-0.703535026771497,0.));
#58046=DIRECTION('',(0.710660584319708,0.703535026771497,0.));
#58047=DIRECTION('center_axis',(0.,0.,1.));
#58048=DIRECTION('ref_axis',(-0.710660584319708,-0.703535026771497,0.));
#58049=DIRECTION('center_axis',(-0.710660584319705,-0.7035350267715,0.));
#58050=DIRECTION('ref_axis',(0.7035350267715,-0.710660584319705,0.));
#58051=DIRECTION('center_axis',(0.,0.,-1.));
#58052=DIRECTION('ref_axis',(1.,0.,0.));
#58053=DIRECTION('center_axis',(0.,0.,1.));
#58054=DIRECTION('ref_axis',(1.,0.,0.));
#58055=DIRECTION('center_axis',(-0.710660584319708,-0.703535026771498,0.));
#58056=DIRECTION('ref_axis',(0.703535026771498,-0.710660584319708,0.));
#58057=DIRECTION('',(0.710660584319708,0.703535026771497,0.));
#58058=DIRECTION('',(-0.710660584319708,-0.703535026771497,0.));
#58059=DIRECTION('center_axis',(0.,0.,1.));
#58060=DIRECTION('ref_axis',(1.,0.,0.));
#58061=DIRECTION('center_axis',(-0.538450589001472,0.842657085179949,1.16942162228788E-14));
#58062=DIRECTION('ref_axis',(0.842657085179949,0.538450589001472,-2.58948405569131E-29));
#58063=DIRECTION('center_axis',(0.837188370386661,-0.546914648267284,0.));
#58064=DIRECTION('ref_axis',(-0.546914648267284,-0.837188370386661,0.));
#58065=DIRECTION('center_axis',(0.,0.,1.));
#58066=DIRECTION('ref_axis',(1.,0.,0.));
#58067=DIRECTION('center_axis',(0.,0.,1.));
#58068=DIRECTION('ref_axis',(1.,0.,0.));
#58069=DIRECTION('center_axis',(0.,0.,1.));
#58070=DIRECTION('ref_axis',(1.,0.,0.));
#58071=DIRECTION('center_axis',(0.,0.,-1.));
#58072=DIRECTION('ref_axis',(-1.,0.,0.));
#58073=DIRECTION('center_axis',(0.,0.,1.));
#58074=DIRECTION('ref_axis',(-1.,-6.93889390390722E-15,0.));
#58075=DIRECTION('',(0.,0.,1.));
#58076=DIRECTION('center_axis',(-0.710660584319708,-0.703535026771498,0.));
#58077=DIRECTION('ref_axis',(0.703535026771498,-0.710660584319708,0.));
#58078=DIRECTION('center_axis',(0.710660584319703,0.703535026771502,-3.66131618133748E-15));
#58079=DIRECTION('ref_axis',(-0.703535026771502,0.710660584319703,4.48656828425865E-30));
#58080=DIRECTION('',(-0.710660584319708,-0.703535026771497,0.));
#58081=DIRECTION('',(0.710660584319708,0.703535026771497,0.));
#58082=DIRECTION('center_axis',(0.710660584319708,0.703535026771498,0.));
#58083=DIRECTION('ref_axis',(-0.703535026771498,0.710660584319708,0.));
#58084=DIRECTION('center_axis',(0.7106605843197,0.703535026771505,0.));
#58085=DIRECTION('ref_axis',(-0.703535026771505,0.7106605843197,0.));
#58086=DIRECTION('',(-0.710660584319708,-0.703535026771497,0.));
#58087=DIRECTION('',(0.710660584319708,0.703535026771497,0.));
#58088=DIRECTION('center_axis',(0.,0.,-1.));
#58089=DIRECTION('ref_axis',(0.989914405816618,-0.141666753886477,0.));
#58090=DIRECTION('center_axis',(0.,0.,1.));
#58091=DIRECTION('ref_axis',(-1.,6.93889390390722E-15,0.));
#58092=DIRECTION('',(0.,0.,-1.));
#58093=DIRECTION('center_axis',(0.710660584319718,0.703535026771487,0.));
#58094=DIRECTION('ref_axis',(-0.703535026771487,0.710660584319718,0.));
#58095=DIRECTION('center_axis',(0.,0.,1.));
#58096=DIRECTION('ref_axis',(-0.710660584319708,-0.703535026771497,0.));
#58097=DIRECTION('center_axis',(0.,0.,1.));
#58098=DIRECTION('ref_axis',(1.,0.,0.));
#58099=DIRECTION('center_axis',(0.,0.,-1.));
#58100=DIRECTION('ref_axis',(1.,0.,0.));
#58101=DIRECTION('center_axis',(0.710660584319702,0.703535026771503,9.76350981689998E-15));
#58102=DIRECTION('ref_axis',(-0.703535026771503,0.710660584319702,-1.13654707447903E-31));
#58103=DIRECTION('center_axis',(-0.710660584319708,-0.703535026771498,0.));
#58104=DIRECTION('ref_axis',(0.703535026771498,-0.710660584319708,0.));
#58105=DIRECTION('',(0.710660584319708,0.703535026771497,0.));
#58106=DIRECTION('',(-0.710660584319708,-0.703535026771497,0.));
#58107=DIRECTION('center_axis',(0.710660584319708,0.703535026771498,0.));
#58108=DIRECTION('ref_axis',(-0.703535026771498,0.710660584319708,0.));
#58109=DIRECTION('',(0.710660584319708,0.703535026771497,0.));
#58110=DIRECTION('',(-0.710660584319708,-0.703535026771497,0.));
#58111=DIRECTION('center_axis',(0.,0.,1.));
#58112=DIRECTION('ref_axis',(1.,0.,0.));
#58113=DIRECTION('center_axis',(0.,0.,1.));
#58114=DIRECTION('ref_axis',(1.,0.,0.));
#58115=DIRECTION('center_axis',(0.,0.,1.));
#58116=DIRECTION('ref_axis',(-0.710660584319707,-0.703535026771498,0.));
#58117=DIRECTION('',(0.,0.,1.));
#58118=DIRECTION('',(0.,0.,1.));
#58119=DIRECTION('center_axis',(-0.703535026771498,0.710660584319708,0.));
#58120=DIRECTION('ref_axis',(-0.710660584319708,-0.703535026771498,0.));
#58121=DIRECTION('center_axis',(0.703535026771498,-0.710660584319708,0.));
#58122=DIRECTION('ref_axis',(0.710660584319708,0.703535026771498,0.));
#58123=DIRECTION('center_axis',(0.,0.,1.));
#58124=DIRECTION('ref_axis',(1.,0.,0.));
#58125=DIRECTION('center_axis',(0.710660584319708,0.703535026771498,0.));
#58126=DIRECTION('ref_axis',(-0.703535026771498,0.710660584319708,0.));
#58127=DIRECTION('center_axis',(0.710660584319702,0.703535026771503,0.));
#58128=DIRECTION('ref_axis',(-0.703535026771503,0.710660584319702,0.));
#58129=DIRECTION('',(-0.710660584319708,-0.703535026771497,0.));
#58130=DIRECTION('',(0.710660584319708,0.703535026771497,0.));
#58131=DIRECTION('center_axis',(0.,0.,1.));
#58132=DIRECTION('ref_axis',(-0.710660584319708,-0.703535026771497,0.));
#58133=DIRECTION('center_axis',(-0.710660584319705,-0.7035350267715,0.));
#58134=DIRECTION('ref_axis',(0.7035350267715,-0.710660584319705,0.));
#58135=DIRECTION('center_axis',(0.,0.,-1.));
#58136=DIRECTION('ref_axis',(1.,0.,0.));
#58137=DIRECTION('center_axis',(0.,0.,1.));
#58138=DIRECTION('ref_axis',(1.,0.,0.));
#58139=DIRECTION('center_axis',(-0.710660584319708,-0.703535026771498,0.));
#58140=DIRECTION('ref_axis',(0.703535026771498,-0.710660584319708,0.));
#58141=DIRECTION('',(0.710660584319708,0.703535026771497,0.));
#58142=DIRECTION('',(-0.710660584319708,-0.703535026771497,0.));
#58143=DIRECTION('center_axis',(0.,0.,1.));
#58144=DIRECTION('ref_axis',(1.,0.,0.));
#58145=DIRECTION('center_axis',(-0.538450589001472,0.842657085179949,1.16942162228788E-14));
#58146=DIRECTION('ref_axis',(0.842657085179949,0.538450589001472,-6.90946196667231E-29));
#58147=DIRECTION('center_axis',(0.837188370386661,-0.546914648267284,0.));
#58148=DIRECTION('ref_axis',(-0.546914648267284,-0.837188370386661,0.));
#58149=DIRECTION('center_axis',(0.,0.,1.));
#58150=DIRECTION('ref_axis',(1.,0.,0.));
#58151=DIRECTION('center_axis',(0.,0.,1.));
#58152=DIRECTION('ref_axis',(1.,0.,0.));
#58153=DIRECTION('center_axis',(0.,0.,1.));
#58154=DIRECTION('ref_axis',(1.,0.,0.));
#58155=DIRECTION('center_axis',(0.,0.,-1.));
#58156=DIRECTION('ref_axis',(-1.,0.,0.));
#58157=DIRECTION('center_axis',(0.,0.,1.));
#58158=DIRECTION('ref_axis',(-1.,-2.77555756156289E-14,0.));
#58159=DIRECTION('',(0.,0.,1.));
#58160=DIRECTION('center_axis',(-0.710660584319708,-0.703535026771498,0.));
#58161=DIRECTION('ref_axis',(0.703535026771498,-0.710660584319708,0.));
#58162=DIRECTION('center_axis',(0.710660584319703,0.703535026771502,-3.66131618133748E-15));
#58163=DIRECTION('ref_axis',(-0.703535026771502,0.710660584319703,-1.3070762122351E-29));
#58164=DIRECTION('',(-0.710660584319708,-0.703535026771497,0.));
#58165=DIRECTION('',(0.710660584319708,0.703535026771497,0.));
#58166=DIRECTION('center_axis',(0.710660584319708,0.703535026771498,0.));
#58167=DIRECTION('ref_axis',(-0.703535026771498,0.710660584319708,0.));
#58168=DIRECTION('center_axis',(0.7106605843197,0.703535026771505,0.));
#58169=DIRECTION('ref_axis',(-0.703535026771505,0.7106605843197,0.));
#58170=DIRECTION('',(-0.710660584319708,-0.703535026771497,0.));
#58171=DIRECTION('',(0.710660584319708,0.703535026771497,0.));
#58172=DIRECTION('center_axis',(0.,0.,-1.));
#58173=DIRECTION('ref_axis',(0.989914405816619,-0.141666753886473,0.));
#58174=DIRECTION('center_axis',(0.,0.,1.));
#58175=DIRECTION('ref_axis',(-1.,2.77555756156289E-14,0.));
#58176=DIRECTION('',(0.,0.,-1.));
#58177=DIRECTION('center_axis',(0.710660584319718,0.703535026771487,0.));
#58178=DIRECTION('ref_axis',(-0.703535026771488,0.710660584319718,0.));
#58179=DIRECTION('center_axis',(0.,0.,1.));
#58180=DIRECTION('ref_axis',(-0.710660584319709,-0.703535026771496,0.));
#58181=DIRECTION('center_axis',(0.,0.,1.));
#58182=DIRECTION('ref_axis',(1.,0.,0.));
#58183=DIRECTION('center_axis',(0.,0.,-1.));
#58184=DIRECTION('ref_axis',(1.,0.,0.));
#58185=DIRECTION('center_axis',(0.710660584319702,0.703535026771503,9.76350981689998E-15));
#58186=DIRECTION('ref_axis',(-0.703535026771503,0.710660584319702,4.82056583115707E-29));
#58187=DIRECTION('center_axis',(-0.710660584319708,-0.703535026771498,0.));
#58188=DIRECTION('ref_axis',(0.703535026771498,-0.710660584319708,0.));
#58189=DIRECTION('',(0.710660584319708,0.703535026771497,0.));
#58190=DIRECTION('',(-0.710660584319708,-0.703535026771497,0.));
#58191=DIRECTION('center_axis',(0.710660584319708,0.703535026771498,0.));
#58192=DIRECTION('ref_axis',(-0.703535026771498,0.710660584319708,0.));
#58193=DIRECTION('',(0.710660584319708,0.703535026771497,0.));
#58194=DIRECTION('',(-0.710660584319708,-0.703535026771497,0.));
#58195=DIRECTION('center_axis',(0.,0.,1.));
#58196=DIRECTION('ref_axis',(1.,0.,0.));
#58197=DIRECTION('center_axis',(0.,0.,1.));
#58198=DIRECTION('ref_axis',(1.,0.,0.));
#58199=DIRECTION('center_axis',(0.,0.,1.));
#58200=DIRECTION('ref_axis',(-0.710660584319709,-0.703535026771496,0.));
#58201=DIRECTION('',(0.,0.,1.));
#58202=DIRECTION('',(0.,0.,1.));
#58203=DIRECTION('center_axis',(-0.703535026771498,0.710660584319708,0.));
#58204=DIRECTION('ref_axis',(-0.710660584319708,-0.703535026771498,0.));
#58205=DIRECTION('center_axis',(0.703535026771498,-0.710660584319708,0.));
#58206=DIRECTION('ref_axis',(0.710660584319708,0.703535026771498,0.));
#58207=DIRECTION('center_axis',(0.,0.,1.));
#58208=DIRECTION('ref_axis',(1.,0.,0.));
#58209=DIRECTION('center_axis',(0.710660584319708,0.703535026771498,0.));
#58210=DIRECTION('ref_axis',(-0.703535026771498,0.710660584319708,0.));
#58211=DIRECTION('center_axis',(0.710660584319702,0.703535026771503,0.));
#58212=DIRECTION('ref_axis',(-0.703535026771503,0.710660584319702,0.));
#58213=DIRECTION('',(-0.710660584319708,-0.703535026771497,0.));
#58214=DIRECTION('',(0.710660584319708,0.703535026771497,0.));
#58215=DIRECTION('center_axis',(0.,0.,1.));
#58216=DIRECTION('ref_axis',(-0.710660584319709,-0.703535026771496,0.));
#58217=DIRECTION('center_axis',(-0.710660584319705,-0.7035350267715,0.));
#58218=DIRECTION('ref_axis',(0.7035350267715,-0.710660584319705,0.));
#58219=DIRECTION('center_axis',(0.,0.,-1.));
#58220=DIRECTION('ref_axis',(1.,0.,0.));
#58221=DIRECTION('center_axis',(0.,0.,1.));
#58222=DIRECTION('ref_axis',(1.,0.,0.));
#58223=DIRECTION('center_axis',(-0.710660584319708,-0.703535026771498,0.));
#58224=DIRECTION('ref_axis',(0.703535026771498,-0.710660584319708,0.));
#58225=DIRECTION('',(0.710660584319708,0.703535026771497,0.));
#58226=DIRECTION('',(-0.710660584319708,-0.703535026771497,0.));
#58227=DIRECTION('center_axis',(0.,0.,1.));
#58228=DIRECTION('ref_axis',(1.,0.,0.));
#58229=DIRECTION('center_axis',(-0.538450589001472,0.842657085179949,1.16942162228788E-14));
#58230=DIRECTION('ref_axis',(0.842657085179949,0.538450589001472,-6.90946196667231E-29));
#58231=DIRECTION('center_axis',(0.837188370386661,-0.546914648267284,0.));
#58232=DIRECTION('ref_axis',(-0.546914648267284,-0.837188370386661,0.));
#58233=DIRECTION('center_axis',(0.,0.,1.));
#58234=DIRECTION('ref_axis',(1.,0.,0.));
#58235=DIRECTION('center_axis',(0.,0.,1.));
#58236=DIRECTION('ref_axis',(1.,0.,0.));
#58237=DIRECTION('center_axis',(0.,0.,1.));
#58238=DIRECTION('ref_axis',(1.,0.,0.));
#58239=DIRECTION('center_axis',(0.,0.,-1.));
#58240=DIRECTION('ref_axis',(-1.,0.,0.));
#58241=DIRECTION('center_axis',(0.,0.,1.));
#58242=DIRECTION('ref_axis',(-1.,-2.77555756156289E-14,0.));
#58243=DIRECTION('',(0.,0.,1.));
#58244=DIRECTION('center_axis',(-0.710660584319708,-0.703535026771498,0.));
#58245=DIRECTION('ref_axis',(0.703535026771498,-0.710660584319708,0.));
#58246=DIRECTION('center_axis',(0.710660584319703,0.703535026771502,-3.66131618133748E-15));
#58247=DIRECTION('ref_axis',(-0.703535026771502,0.710660584319703,-1.3070762122351E-29));
#58248=DIRECTION('',(-0.710660584319708,-0.703535026771497,0.));
#58249=DIRECTION('',(0.710660584319708,0.703535026771497,0.));
#58250=DIRECTION('center_axis',(0.710660584319708,0.703535026771498,0.));
#58251=DIRECTION('ref_axis',(-0.703535026771498,0.710660584319708,0.));
#58252=DIRECTION('center_axis',(0.7106605843197,0.703535026771505,0.));
#58253=DIRECTION('ref_axis',(-0.703535026771505,0.7106605843197,0.));
#58254=DIRECTION('',(-0.710660584319708,-0.703535026771497,0.));
#58255=DIRECTION('',(0.710660584319708,0.703535026771497,0.));
#58256=DIRECTION('center_axis',(0.,0.,-1.));
#58257=DIRECTION('ref_axis',(0.989914405816618,-0.141666753886482,0.));
#58258=DIRECTION('center_axis',(0.,0.,1.));
#58259=DIRECTION('ref_axis',(-1.,4.85722573273506E-14,0.));
#58260=DIRECTION('',(0.,0.,-1.));
#58261=DIRECTION('center_axis',(0.710660584319718,0.703535026771487,0.));
#58262=DIRECTION('ref_axis',(-0.703535026771487,0.710660584319718,0.));
#58263=DIRECTION('center_axis',(0.,0.,1.));
#58264=DIRECTION('ref_axis',(-0.710660584319709,-0.703535026771496,0.));
#58265=DIRECTION('center_axis',(0.,0.,1.));
#58266=DIRECTION('ref_axis',(1.,0.,0.));
#58267=DIRECTION('center_axis',(0.,0.,-1.));
#58268=DIRECTION('ref_axis',(1.,0.,0.));
#58269=DIRECTION('center_axis',(0.710660584319702,0.703535026771503,9.76350981689998E-15));
#58270=DIRECTION('ref_axis',(-0.703535026771503,0.710660584319702,4.82056583115707E-29));
#58271=DIRECTION('center_axis',(-0.710660584319708,-0.703535026771498,0.));
#58272=DIRECTION('ref_axis',(0.703535026771498,-0.710660584319708,0.));
#58273=DIRECTION('',(0.710660584319708,0.703535026771497,0.));
#58274=DIRECTION('',(-0.710660584319708,-0.703535026771497,0.));
#58275=DIRECTION('center_axis',(0.710660584319708,0.703535026771498,0.));
#58276=DIRECTION('ref_axis',(-0.703535026771498,0.710660584319708,0.));
#58277=DIRECTION('',(0.710660584319708,0.703535026771497,0.));
#58278=DIRECTION('',(-0.710660584319708,-0.703535026771497,0.));
#58279=DIRECTION('center_axis',(0.,0.,1.));
#58280=DIRECTION('ref_axis',(1.,0.,0.));
#58281=DIRECTION('center_axis',(0.,0.,1.));
#58282=DIRECTION('ref_axis',(1.,0.,0.));
#58283=DIRECTION('center_axis',(0.,0.,1.));
#58284=DIRECTION('ref_axis',(-0.710660584319707,-0.703535026771498,0.));
#58285=DIRECTION('',(0.,0.,1.));
#58286=DIRECTION('',(0.,0.,1.));
#58287=DIRECTION('center_axis',(-0.703535026771498,0.710660584319708,0.));
#58288=DIRECTION('ref_axis',(-0.710660584319708,-0.703535026771498,0.));
#58289=DIRECTION('center_axis',(0.703535026771498,-0.710660584319708,0.));
#58290=DIRECTION('ref_axis',(0.710660584319708,0.703535026771498,0.));
#58291=DIRECTION('center_axis',(0.,0.,1.));
#58292=DIRECTION('ref_axis',(1.,0.,0.));
#58293=DIRECTION('center_axis',(0.,0.,1.));
#58294=DIRECTION('ref_axis',(1.,0.,0.));
#58295=DIRECTION('',(1.,0.,0.));
#58296=DIRECTION('center_axis',(0.,0.,1.));
#58297=DIRECTION('ref_axis',(1.,0.,0.));
#58298=DIRECTION('',(1.,0.,0.));
#58299=DIRECTION('center_axis',(0.,0.,1.));
#58300=DIRECTION('ref_axis',(1.,0.,0.));
#58301=DIRECTION('',(1.,0.,0.));
#58302=DIRECTION('center_axis',(0.,0.,1.));
#58303=DIRECTION('ref_axis',(1.,0.,0.));
#58304=DIRECTION('center_axis',(0.,0.,1.));
#58305=DIRECTION('ref_axis',(1.,0.,0.));
#58306=DIRECTION('center_axis',(0.,0.,-1.));
#58307=DIRECTION('ref_axis',(-1.,0.,0.));
#58308=DIRECTION('',(0.,0.,1.));
#58309=DIRECTION('center_axis',(0.,-1.,0.));
#58310=DIRECTION('ref_axis',(0.,0.,-1.));
#58311=DIRECTION('center_axis',(0.00367439112755605,0.,-0.999993249402136));
#58312=DIRECTION('ref_axis',(-0.999993249402136,0.,-0.00367439112755605));
#58313=DIRECTION('center_axis',(0.,-1.,0.));
#58314=DIRECTION('ref_axis',(0.,0.,-1.));
#58315=DIRECTION('center_axis',(0.,-1.,0.));
#58316=DIRECTION('ref_axis',(0.,0.,-1.));
#58317=DIRECTION('center_axis',(1.,0.,0.));
#58318=DIRECTION('ref_axis',(0.,0.,-1.));
#58319=DIRECTION('center_axis',(0.993664622325388,0.,-0.112386023770502));
#58320=DIRECTION('ref_axis',(-0.112386023770502,0.,-0.993664622325388));
#58321=DIRECTION('center_axis',(1.,0.,0.));
#58322=DIRECTION('ref_axis',(0.,0.,-1.));
#58323=DIRECTION('center_axis',(1.,0.,0.));
#58324=DIRECTION('ref_axis',(0.,0.,-1.));
#58325=DIRECTION('',(1.,0.,0.));
#58326=DIRECTION('center_axis',(0.992466262760427,0.,-0.12251823244869));
#58327=DIRECTION('ref_axis',(-0.12251823244869,0.,-0.992466262760427));
#58328=DIRECTION('center_axis',(0.,0.,-1.));
#58329=DIRECTION('ref_axis',(-1.,0.,0.));
#58330=DIRECTION('center_axis',(0.,-1.,0.));
#58331=DIRECTION('ref_axis',(0.,0.,-1.));
#58332=DIRECTION('center_axis',(0.998253744921096,0.,-0.0590716577641654));
#58333=DIRECTION('ref_axis',(-0.0590716577641654,0.,-0.998253744921096));
#58334=DIRECTION('center_axis',(0.,0.,-1.));
#58335=DIRECTION('ref_axis',(-1.,0.,0.));
#58336=DIRECTION('center_axis',(0.,0.,-1.));
#58337=DIRECTION('ref_axis',(-1.,0.,0.));
#58338=DIRECTION('',(0.,0.,-1.));
#58339=DIRECTION('center_axis',(0.997326999817373,0.,-0.073067471800225));
#58340=DIRECTION('ref_axis',(-0.073067471800225,0.,-0.997326999817374));
#58341=DIRECTION('center_axis',(0.,-1.,0.));
#58342=DIRECTION('ref_axis',(0.,0.,-1.));
#58343=DIRECTION('center_axis',(-0.00367439112755605,2.77553882489006E-14,
-0.999993249402136));
#58344=DIRECTION('ref_axis',(-0.999993249402136,2.07077330159731E-32,0.00367439112755605));
#58345=DIRECTION('center_axis',(0.,-1.,0.));
#58346=DIRECTION('ref_axis',(0.,0.,-1.));
#58347=DIRECTION('center_axis',(1.,0.,-2.83753250766945E-16));
#58348=DIRECTION('ref_axis',(-2.83753250766945E-16,0.,-1.));
#58349=DIRECTION('center_axis',(0.,1.,0.));
#58350=DIRECTION('ref_axis',(0.,0.,1.));
#58351=DIRECTION('',(0.,-1.,0.));
#58352=DIRECTION('',(0.,1.,0.));
#58353=DIRECTION('center_axis',(4.16333634234433E-14,1.,0.));
#58354=DIRECTION('ref_axis',(-1.,4.16333634234433E-14,0.));
#58355=DIRECTION('center_axis',(-1.,-1.30289899094001E-16,0.));
#58356=DIRECTION('ref_axis',(1.30289899094001E-16,-1.,0.));
#58357=DIRECTION('center_axis',(-0.99083605930949,-0.135069995084183,-4.3932954632363E-16));
#58358=DIRECTION('ref_axis',(-0.135069995084183,0.99083605930949,-1.6477538710012E-33));
#58359=DIRECTION('center_axis',(0.,0.,-1.));
#58360=DIRECTION('ref_axis',(-1.,0.,0.));
#58361=DIRECTION('center_axis',(-0.870187309198622,0.492721064000376,0.));
#58362=DIRECTION('ref_axis',(-0.492721064000376,-0.870187309198622,0.));
#58363=DIRECTION('center_axis',(0.,0.,1.));
#58364=DIRECTION('ref_axis',(-1.,2.13045726893401E-14,0.));
#58365=DIRECTION('center_axis',(0.,0.,-1.));
#58366=DIRECTION('ref_axis',(-1.,0.,0.));
#58367=DIRECTION('center_axis',(0.,0.,-1.));
#58368=DIRECTION('ref_axis',(-1.,0.,0.));
#58369=DIRECTION('center_axis',(-0.589792031258401,-0.807555174501464,0.));
#58370=DIRECTION('ref_axis',(-0.807555174501464,0.589792031258401,0.));
#58371=DIRECTION('center_axis',(0.,0.,-1.));
#58372=DIRECTION('ref_axis',(-1.,0.,0.));
#58373=DIRECTION('center_axis',(0.,0.,-1.));
#58374=DIRECTION('ref_axis',(-1.,0.,0.));
#58375=DIRECTION('center_axis',(0.,0.,1.));
#58376=DIRECTION('ref_axis',(1.,0.,0.));
#58377=DIRECTION('',(0.,0.,1.));
#58378=DIRECTION('center_axis',(0.,0.,-1.));
#58379=DIRECTION('ref_axis',(-1.,0.,0.));
#58380=DIRECTION('center_axis',(-0.950587351628009,-0.310457222375076,0.));
#58381=DIRECTION('ref_axis',(0.310457222375076,-0.950587351628009,0.));
#58382=DIRECTION('center_axis',(0.,0.,1.));
#58383=DIRECTION('ref_axis',(-1.,-2.42861286636753E-14,0.));
#58384=DIRECTION('center_axis',(0.,0.,-1.));
#58385=DIRECTION('ref_axis',(-1.,0.,0.));
#58386=DIRECTION('center_axis',(-0.813624755504625,0.581390365615083,-1.49473109573578E-14));
#58387=DIRECTION('ref_axis',(-0.581390365615083,-0.813624755504625,-2.20695383221015E-29));
#58388=DIRECTION('center_axis',(0.,-1.,0.));
#58389=DIRECTION('ref_axis',(0.,0.,-1.));
#58390=DIRECTION('center_axis',(0.,0.,-1.));
#58391=DIRECTION('ref_axis',(-1.,0.,0.));
#58392=DIRECTION('center_axis',(-1.40023216580064E-13,-1.91722619337689E-13,
1.));
#58393=DIRECTION('ref_axis',(-3.59356979302414E-28,-1.,-1.91722619337689E-13));
#58394=DIRECTION('',(0.,0.,-1.));
#58395=DIRECTION('center_axis',(0.,0.,-1.));
#58396=DIRECTION('ref_axis',(-1.,0.,0.));
#58397=DIRECTION('center_axis',(-0.0533420240673326,0.998576300774458,-2.72423821176928E-15));
#58398=DIRECTION('ref_axis',(-0.998576300774458,-0.0533420240673326,-4.56897457660181E-33));
#58399=DIRECTION('center_axis',(0.,0.,-1.));
#58400=DIRECTION('ref_axis',(-1.,0.,0.));
#58401=DIRECTION('center_axis',(0.,-1.,0.));
#58402=DIRECTION('ref_axis',(0.,0.,-1.));
#58403=DIRECTION('',(0.,-1.,0.));
#58404=DIRECTION('',(0.,1.,0.));
#58405=DIRECTION('center_axis',(0.498280113808025,0.867016106069237,0.));
#58406=DIRECTION('ref_axis',(-0.867016106069237,0.498280113808025,0.));
#58407=DIRECTION('center_axis',(0.,0.,1.));
#58408=DIRECTION('ref_axis',(0.0533420240673336,-0.998576300774458,0.));
#58409=DIRECTION('center_axis',(0.,0.,1.));
#58410=DIRECTION('ref_axis',(1.,0.,0.));
#58411=DIRECTION('center_axis',(1.,0.,0.));
#58412=DIRECTION('ref_axis',(0.,0.,1.));
#58413=DIRECTION('center_axis',(0.,0.,-1.));
#58414=DIRECTION('ref_axis',(-1.,0.,0.));
#58415=DIRECTION('center_axis',(0.0533420240673341,0.998576300774458,0.));
#58416=DIRECTION('ref_axis',(-0.998576300774458,0.0533420240673341,0.));
#58417=DIRECTION('center_axis',(0.,0.,-1.));
#58418=DIRECTION('ref_axis',(-1.,0.,0.));
#58419=DIRECTION('center_axis',(0.,0.,-1.));
#58420=DIRECTION('ref_axis',(-1.,0.,0.));
#58421=DIRECTION('center_axis',(0.,0.,1.));
#58422=DIRECTION('ref_axis',(1.,0.,0.));
#58423=DIRECTION('',(0.,0.,1.));
#58424=DIRECTION('center_axis',(0.,0.,1.));
#58425=DIRECTION('ref_axis',(0.0533420240673479,0.998576300774457,0.));
#58426=DIRECTION('center_axis',(-1.,0.,0.));
#58427=DIRECTION('ref_axis',(0.,0.,1.));
#58428=DIRECTION('center_axis',(0.,0.,1.));
#58429=DIRECTION('ref_axis',(1.,0.,0.));
#58430=DIRECTION('center_axis',(0.00693238621491237,0.993966797804128,0.109462079664029));
#58431=DIRECTION('ref_axis',(-1.22354345465345E-17,-0.109464710021979,0.993990682682591));
#58432=DIRECTION('center_axis',(0.,0.,-1.));
#58433=DIRECTION('ref_axis',(-1.,0.,0.));
#58434=DIRECTION('center_axis',(2.96529885867188E-15,5.55111512312578E-14,
1.));
#58435=DIRECTION('ref_axis',(0.,-1.,5.55111512312578E-14));
#58436=DIRECTION('',(0.,0.,-1.));
#58437=DIRECTION('center_axis',(0.124001141217911,0.992275239756939,-0.00368314294652425));
#58438=DIRECTION('ref_axis',(-0.992281970201119,0.12400198229781,6.2356654373776E-21));
#58439=DIRECTION('center_axis',(0.0139772935711188,0.879101978084599,0.47642874324727));
#58440=DIRECTION('ref_axis',(2.72212200690293E-17,-0.476475288755116,0.879187863431775));
#58441=DIRECTION('center_axis',(0.994025548953269,0.0701103237587535,-0.0836525584222893));
#58442=DIRECTION('ref_axis',(0.0838589147843666,1.84650881221684E-17,0.996477637687464));
#58443=DIRECTION('center_axis',(-0.456401891282935,0.882037283977672,0.117079218081824));
#58444=DIRECTION('ref_axis',(-0.888145434138644,-0.459562496096754,1.03214570261012E-16));
#58445=DIRECTION('center_axis',(0.992758434166036,-0.0700209519858698,-0.0976102334552734));
#58446=DIRECTION('ref_axis',(-0.0978504052290823,-1.24014805477136E-16,
-0.995201134543417));
#58447=DIRECTION('center_axis',(0.,0.,-1.));
#58448=DIRECTION('ref_axis',(-1.,0.,0.));
#58449=DIRECTION('center_axis',(-1.,0.,4.00096335390287E-16));
#58450=DIRECTION('ref_axis',(4.00096335390287E-16,0.,1.));
#58451=DIRECTION('center_axis',(0.0764633074491056,0.,0.997072395874013));
#58452=DIRECTION('ref_axis',(-0.997072395874013,-2.08166817117216E-14,0.0764633074491056));
#58453=DIRECTION('center_axis',(-0.763137786294476,0.64623580768135,-4.48416170640668E-15));
#58454=DIRECTION('ref_axis',(-0.64623580768135,-0.763137786294476,3.55662332953577E-29));
#58455=DIRECTION('center_axis',(-0.780043230375354,0.625725625770259,1.2139561508471E-13));
#58456=DIRECTION('ref_axis',(-0.625725625770259,-0.780043230375354,-2.63473956355127E-28));
#58457=DIRECTION('center_axis',(5.89460815835388E-12,7.1840930855476E-12,
1.));
#58458=DIRECTION('ref_axis',(-0.625713604765022,-0.780052873087435,9.29240284524464E-12));
#58459=DIRECTION('center_axis',(-0.0132304380228111,-0.00122043043743016,
-0.999911729133763));
#58460=DIRECTION('ref_axis',(-0.646190117710228,-0.763117574189617,0.00948154716257832));
#58461=DIRECTION('center_axis',(-0.0764633074494057,-3.38289393019627E-13,
0.99707239587399));
#58462=DIRECTION('ref_axis',(-0.99707239587399,3.46944695195615E-15,-0.0764633074494057));
#58463=DIRECTION('center_axis',(0.76313778629449,0.646235807681333,0.));
#58464=DIRECTION('ref_axis',(-0.646235807681333,0.76313778629449,0.));
#58465=DIRECTION('center_axis',(-1.,-1.18445362812728E-16,0.));
#58466=DIRECTION('ref_axis',(1.18445362812728E-16,-1.,0.));
#58467=DIRECTION('center_axis',(0.780043230375353,0.625725625770261,0.));
#58468=DIRECTION('ref_axis',(-0.62572562577026,0.780043230375353,0.));
#58469=DIRECTION('center_axis',(0.0135861973191934,-0.00164484670762636,
-0.99990635047574));
#58470=DIRECTION('ref_axis',(0.625603637149145,-0.780079720485556,0.00978360224753608));
#58471=DIRECTION('center_axis',(-7.88065731198386E-12,9.56133411252272E-12,
1.));
#58472=DIRECTION('ref_axis',(0.646224932541722,-0.763146995382572,1.23893231864011E-11));
#58473=DIRECTION('center_axis',(0.,0.,-1.));
#58474=DIRECTION('ref_axis',(-1.,0.,0.));
#58475=DIRECTION('',(-1.,0.,0.));
#58476=DIRECTION('',(-1.,0.,0.));
#58477=DIRECTION('',(-1.,0.,0.));
#58478=DIRECTION('',(-1.,0.,0.));
#58479=DIRECTION('center_axis',(-1.27486239704332E-16,1.,0.));
#58480=DIRECTION('ref_axis',(-1.,-1.27486239704332E-16,0.));
#58481=DIRECTION('',(1.27486239704332E-16,-1.,0.));
#58482=DIRECTION('',(0.,1.,0.));
#58483=DIRECTION('center_axis',(4.62592926927149E-16,1.,3.77688604714562E-13));
#58484=DIRECTION('ref_axis',(8.56727719098818E-33,-3.77688604714562E-13,
1.));
#58485=DIRECTION('center_axis',(-1.,-1.18445362812727E-16,3.8759154073836E-16));
#58486=DIRECTION('ref_axis',(3.8759154073836E-16,5.47382212626882E-48,1.));
#58487=DIRECTION('center_axis',(0.,-1.,1.88844727276056E-13));
#58488=DIRECTION('ref_axis',(0.,-1.88844727276056E-13,-1.));
#58489=DIRECTION('center_axis',(-1.27486239704332E-16,1.,0.));
#58490=DIRECTION('ref_axis',(-1.,-1.27486239704332E-16,0.));
#58491=DIRECTION('',(0.,-1.,0.));
#58492=DIRECTION('',(-1.27486239704332E-16,1.,0.));
#58493=DIRECTION('',(-1.27486239704332E-16,1.,0.));
#58494=DIRECTION('center_axis',(0.,0.,-1.));
#58495=DIRECTION('ref_axis',(-1.,0.,0.));
#58496=DIRECTION('center_axis',(1.,0.,0.));
#58497=DIRECTION('ref_axis',(0.,0.,-1.));
#58498=DIRECTION('',(0.,0.,-1.));
#58499=DIRECTION('center_axis',(-1.,0.,0.));
#58500=DIRECTION('ref_axis',(0.,0.,1.));
#58501=DIRECTION('',(0.,0.,-1.));
#58502=DIRECTION('',(0.,0.,-1.));
#58503=DIRECTION('center_axis',(-1.,0.,0.));
#58504=DIRECTION('ref_axis',(0.,0.,1.));
#58505=DIRECTION('',(1.,0.,0.));
#58506=DIRECTION('',(-1.,0.,0.));
#58507=DIRECTION('center_axis',(0.,0.,-1.));
#58508=DIRECTION('ref_axis',(-1.,0.,0.));
#58509=DIRECTION('center_axis',(0.,1.,0.));
#58510=DIRECTION('ref_axis',(0.,0.,1.));
#58511=DIRECTION('center_axis',(-1.,0.,0.));
#58512=DIRECTION('ref_axis',(0.,0.,1.));
#58513=DIRECTION('',(1.,0.,0.));
#58514=DIRECTION('center_axis',(-1.,0.,0.));
#58515=DIRECTION('ref_axis',(0.,0.,1.));
#58516=DIRECTION('',(1.,0.,0.));
#58517=DIRECTION('center_axis',(-1.,0.,0.));
#58518=DIRECTION('ref_axis',(0.,0.,1.));
#58519=DIRECTION('',(1.,0.,0.));
#58520=DIRECTION('center_axis',(-1.,0.,0.));
#58521=DIRECTION('ref_axis',(0.,0.,1.));
#58522=DIRECTION('',(1.,0.,0.));
#58523=DIRECTION('center_axis',(0.,1.,0.));
#58524=DIRECTION('ref_axis',(0.,0.,1.));
#85906=CARTESIAN_POINT('',(0.,0.,0.));
#85907=CARTESIAN_POINT('Origin',(121.691000639221,53.9,183.212899484195));
#85908=CARTESIAN_POINT('',(121.691000639221,53.9,183.712899484196));
#85909=CARTESIAN_POINT('',(121.691000639221,54.8,183.712899484196));
#85910=CARTESIAN_POINT('',(121.691000639221,53.9,183.712899484196));
#85911=CARTESIAN_POINT('',(121.691000639221,54.8,182.712899484195));
#85912=CARTESIAN_POINT('Origin',(121.691000639221,54.8,183.212899484195));
#85913=CARTESIAN_POINT('',(121.691000639221,53.9,182.712899484195));
#85914=CARTESIAN_POINT('',(121.691000639221,53.9,182.712899484195));
#85915=CARTESIAN_POINT('Origin',(121.691000639221,53.9,183.212899484195));
#85916=CARTESIAN_POINT('Origin',(121.691000639221,53.9,183.712899484196));
#85917=CARTESIAN_POINT('',(106.90475031663,53.9,183.712899484195));
#85918=CARTESIAN_POINT('',(106.90475031663,54.8,183.712899484195));
#85919=CARTESIAN_POINT('',(106.90475031663,53.9,183.712899484195));
#85920=CARTESIAN_POINT('',(-205.7,54.8,183.712899484194));
#85921=CARTESIAN_POINT('',(121.691000639221,53.9,183.712899484196));
#85922=CARTESIAN_POINT('Origin',(106.90475031663,53.9,183.212899484195));
#85923=CARTESIAN_POINT('',(106.90475031663,53.9,182.712899484196));
#85924=CARTESIAN_POINT('',(106.90475031663,54.8,182.712899484196));
#85925=CARTESIAN_POINT('',(106.90475031663,53.9,182.712899484196));
#85926=CARTESIAN_POINT('Origin',(106.90475031663,54.8,183.212899484195));
#85927=CARTESIAN_POINT('Origin',(106.90475031663,53.9,183.212899484195));
#85928=CARTESIAN_POINT('Origin',(121.691000639221,53.9,182.712899484195));
#85929=CARTESIAN_POINT('',(-205.7,54.8,182.712899484197));
#85930=CARTESIAN_POINT('',(121.691000639221,53.9,182.712899484195));
#85931=CARTESIAN_POINT('Origin',(121.691000639221,53.9,183.212899484195));
#85932=CARTESIAN_POINT('Origin',(-205.7,54.8,197.697003183159));
#85933=CARTESIAN_POINT('Origin',(128.895960652199,53.9,183.212899484195));
#85934=CARTESIAN_POINT('',(128.895960652199,53.9,182.712899484195));
#85935=CARTESIAN_POINT('',(128.895960652199,53.9,183.712899484196));
#85936=CARTESIAN_POINT('Origin',(128.895960652199,53.9,183.212899484195));
#85937=CARTESIAN_POINT('',(143.682210974789,53.9,183.712899484195));
#85938=CARTESIAN_POINT('',(128.895960652199,53.9,183.712899484196));
#85939=CARTESIAN_POINT('',(143.682210974789,53.9,182.712899484196));
#85940=CARTESIAN_POINT('Origin',(143.682210974789,53.9,183.212899484195));
#85941=CARTESIAN_POINT('',(128.895960652199,53.9,182.712899484195));
#85942=CARTESIAN_POINT('Origin',(128.895960652199,53.9,183.712899484196));
#85943=CARTESIAN_POINT('',(128.895960652199,54.8,183.712899484196));
#85944=CARTESIAN_POINT('',(128.895960652199,53.9,183.712899484196));
#85945=CARTESIAN_POINT('',(143.682210974789,54.8,183.712899484195));
#85946=CARTESIAN_POINT('',(-205.7,54.8,183.712899484197));
#85947=CARTESIAN_POINT('',(143.682210974789,53.9,183.712899484195));
#85948=CARTESIAN_POINT('Origin',(143.682210974789,53.9,183.212899484195));
#85949=CARTESIAN_POINT('',(143.682210974789,54.8,182.712899484196));
#85950=CARTESIAN_POINT('Origin',(143.682210974789,54.8,183.212899484195));
#85951=CARTESIAN_POINT('',(143.682210974789,53.9,182.712899484196));
#85952=CARTESIAN_POINT('Origin',(128.895960652199,53.9,182.712899484195));
#85953=CARTESIAN_POINT('',(128.895960652199,54.8,182.712899484195));
#85954=CARTESIAN_POINT('',(-205.7,54.8,182.712899484194));
#85955=CARTESIAN_POINT('',(128.895960652199,53.9,182.712899484195));
#85956=CARTESIAN_POINT('Origin',(128.895960652199,53.9,183.212899484195));
#85957=CARTESIAN_POINT('Origin',(128.895960652199,54.8,183.212899484195));
#85958=CARTESIAN_POINT('Origin',(-205.7,54.8,197.697003183159));
#85959=CARTESIAN_POINT('Origin',(125.29348064571,25.4505574462982,200.));
#85960=CARTESIAN_POINT('',(96.7708826633735,25.4505574465334,196.229576409449));
#85961=CARTESIAN_POINT('',(96.8114851745877,23.9291040663932,194.272013743528));
#85962=CARTESIAN_POINT('Ctrl Pts',(96.7708826633735,25.4505574465334,196.229576409449));
#85963=CARTESIAN_POINT('Ctrl Pts',(96.770884572667,25.3888168379312,196.215660891132));
#85964=CARTESIAN_POINT('Ctrl Pts',(96.7710859278689,25.328300044412,196.198742499774));
#85965=CARTESIAN_POINT('Ctrl Pts',(96.7714629075156,25.2689905570161,196.178935869129));
#85966=CARTESIAN_POINT('Ctrl Pts',(96.7718468277933,25.2085891133962,196.158764575518));
#85967=CARTESIAN_POINT('Ctrl Pts',(96.7724129528313,25.1494394923947,196.135597518842));
#85968=CARTESIAN_POINT('Ctrl Pts',(96.7731397544311,25.0915407352726,196.109504170528));
#85969=CARTESIAN_POINT('Ctrl Pts',(96.7736290811383,25.0525597971678,196.091936553429));
#85970=CARTESIAN_POINT('Ctrl Pts',(96.7741913136005,25.0141461969243,196.073041442187));
#85971=CARTESIAN_POINT('Ctrl Pts',(96.7748205968608,24.9763049437873,196.052827902151));
#85972=CARTESIAN_POINT('Ctrl Pts',(96.775605887767,24.9290823433476,196.02760315811));
#85973=CARTESIAN_POINT('Ctrl Pts',(96.7764993817748,24.8825802014245,196.000147388779));
#85974=CARTESIAN_POINT('Ctrl Pts',(96.7774766184748,24.8371623486203,195.970690132415));
#85975=CARTESIAN_POINT('Ctrl Pts',(96.7785956662022,24.7851537155424,195.936958206682));
#85976=CARTESIAN_POINT('Ctrl Pts',(96.7798169585537,24.7349116033477,195.900837873986));
#85977=CARTESIAN_POINT('Ctrl Pts',(96.7811015898682,24.686931282354,195.862746601214));
#85978=CARTESIAN_POINT('Ctrl Pts',(96.78117851315,24.6840582372147,195.860465708885));
#85979=CARTESIAN_POINT('Ctrl Pts',(96.7812556644065,24.6811933013905,195.85817773446));
#85980=CARTESIAN_POINT('Ctrl Pts',(96.7813330355974,24.6783365813196,195.855882761992));
#85981=CARTESIAN_POINT('Ctrl Pts',(96.7827143680617,24.6273346498515,195.814909889032));
#85982=CARTESIAN_POINT('Ctrl Pts',(96.7841695078232,24.5786282396643,195.771582834397));
#85983=CARTESIAN_POINT('Ctrl Pts',(96.7856684582633,24.5321043729733,195.725832497918));
#85984=CARTESIAN_POINT('Ctrl Pts',(96.786903293901,24.4937780033667,195.688143362636));
#85985=CARTESIAN_POINT('Ctrl Pts',(96.7881679285545,24.4569334037587,195.648808966062));
#85986=CARTESIAN_POINT('Ctrl Pts',(96.7894462372192,24.4215244761583,195.607770307954));
#85987=CARTESIAN_POINT('Ctrl Pts',(96.7903511917988,24.3964573917586,195.578717761713));
#85988=CARTESIAN_POINT('Ctrl Pts',(96.7912621271681,24.3721489380842,195.548811846036));
#85989=CARTESIAN_POINT('Ctrl Pts',(96.7921699928626,24.3486689952047,195.518156906328));
#85990=CARTESIAN_POINT('Ctrl Pts',(96.7935847249944,24.3120800703772,195.470387144268));
#85991=CARTESIAN_POINT('Ctrl Pts',(96.7949823397169,24.2777486344132,195.421117146607));
#85992=CARTESIAN_POINT('Ctrl Pts',(96.7963302088508,24.2458601081044,195.37075500768));
#85993=CARTESIAN_POINT('Ctrl Pts',(96.7968332917952,24.2339579335512,195.351957683446));
#85994=CARTESIAN_POINT('Ctrl Pts',(96.7973294572306,24.2223963168555,195.333007722924));
#85995=CARTESIAN_POINT('Ctrl Pts',(96.7978170366339,24.2111858784597,195.3139248247));
#85996=CARTESIAN_POINT('Ctrl Pts',(96.7991683406123,24.1801166620386,195.261037446533));
#85997=CARTESIAN_POINT('Ctrl Pts',(96.8004619805254,24.151517163759,195.20689229819));
#85998=CARTESIAN_POINT('Ctrl Pts',(96.8016796026155,24.1253390270934,195.151352643979));
#85999=CARTESIAN_POINT('Ctrl Pts',(96.8028512729684,24.1001488249169,195.097908996089));
#86000=CARTESIAN_POINT('Ctrl Pts',(96.8039526057457,24.0772008393268,195.043174016525));
#86001=CARTESIAN_POINT('Ctrl Pts',(96.8049660037159,24.0564914865203,194.987003196263));
#86002=CARTESIAN_POINT('Ctrl Pts',(96.8053085104808,24.0494921697253,194.968018664525));
#86003=CARTESIAN_POINT('Ctrl Pts',(96.8056393130589,24.0427722122427,194.948929948601));
#86004=CARTESIAN_POINT('Ctrl Pts',(96.8059580529338,24.0363324515711,194.929737855852));
#86005=CARTESIAN_POINT('Ctrl Pts',(96.8068918795025,24.0174655946617,194.873509917246));
#86006=CARTESIAN_POINT('Ctrl Pts',(96.8077148336768,24.0011508604124,194.816857349836));
#86007=CARTESIAN_POINT('Ctrl Pts',(96.8084222566688,23.9873133973046,194.759798812559));
#86008=CARTESIAN_POINT('Ctrl Pts',(96.8091332048146,23.9734069808486,194.702455947356));
#86009=CARTESIAN_POINT('Ctrl Pts',(96.8097274986935,23.9620025122422,194.644702547731));
#86010=CARTESIAN_POINT('Ctrl Pts',(96.8101983286926,23.9530743260575,194.586541266325));
#86011=CARTESIAN_POINT('Ctrl Pts',(96.8106680291585,23.9441675588171,194.528519515303));
#86012=CARTESIAN_POINT('Ctrl Pts',(96.8110148873442,23.9377251529057,194.470091329796));
#86013=CARTESIAN_POINT('Ctrl Pts',(96.8112296232299,23.9337724353167,194.41125080931));
#86014=CARTESIAN_POINT('Ctrl Pts',(96.8113980719359,23.9306717418256,194.365093598536));
#86015=CARTESIAN_POINT('Ctrl Pts',(96.8114851744842,23.9291040683311,194.31868240643));
#86016=CARTESIAN_POINT('Ctrl Pts',(96.8114851745877,23.9291040663932,194.272013743528));
#86017=CARTESIAN_POINT('',(96.8114851745877,23.9291040663932,152.608250755187));
#86018=CARTESIAN_POINT('',(96.8114851745877,23.9291040663932,200.));
#86019=CARTESIAN_POINT('',(108.710714013295,2.24386148976204,152.608250755187));
#86020=CARTESIAN_POINT('Origin',(125.29348064571,25.4505574462982,152.608250755187));
#86021=CARTESIAN_POINT('',(111.239793308547,0.630550221611421,150.608250755187));
#86022=CARTESIAN_POINT('Ctrl Pts',(108.710714013295,2.24386148976203,152.608250755187));
#86023=CARTESIAN_POINT('Ctrl Pts',(108.853554035459,2.14179255423786,152.608250752516));
#86024=CARTESIAN_POINT('Ctrl Pts',(108.996115566955,2.04191344387966,152.597109166573));
#86025=CARTESIAN_POINT('Ctrl Pts',(109.138428228549,1.94410762303756,152.574931667418));
#86026=CARTESIAN_POINT('Ctrl Pts',(109.261361350294,1.85962058761654,152.555774206844));
#86027=CARTESIAN_POINT('Ctrl Pts',(109.384108759692,1.77668082196495,152.528380974701));
#86028=CARTESIAN_POINT('Ctrl Pts',(109.506688753907,1.69521934777192,152.492789418762));
#86029=CARTESIAN_POINT('Ctrl Pts',(109.509657719578,1.69324629889127,152.491927368569));
#86030=CARTESIAN_POINT('Ctrl Pts',(109.512625826965,1.6912746327679,152.491060749244));
#86031=CARTESIAN_POINT('Ctrl Pts',(109.515593066985,1.689304352752,152.490189550154));
#86032=CARTESIAN_POINT('Ctrl Pts',(109.648551129122,1.60101873682548,152.451152282539));
#86033=CARTESIAN_POINT('Ctrl Pts',(109.779549079908,1.51566120719707,152.402991156227));
#86034=CARTESIAN_POINT('Ctrl Pts',(109.907692820099,1.43356899326917,152.344885850416));
#86035=CARTESIAN_POINT('Ctrl Pts',(110.032432777243,1.35365733131867,152.288323950896));
#86036=CARTESIAN_POINT('Ctrl Pts',(110.154467914824,1.27683990420537,152.222338990309));
#86037=CARTESIAN_POINT('Ctrl Pts',(110.272995112549,1.20341533113175,152.146214709741));
#86038=CARTESIAN_POINT('Ctrl Pts',(110.277494300693,1.20062819893815,152.143325099026));
#86039=CARTESIAN_POINT('Ctrl Pts',(110.281989807978,1.19784513176216,152.14041918704));
#86040=CARTESIAN_POINT('Ctrl Pts',(110.286481320508,1.19506630191825,152.137497018263));
#86041=CARTESIAN_POINT('Ctrl Pts',(110.35623096888,1.15191326533487,152.092118041067));
#86042=CARTESIAN_POINT('Ctrl Pts',(110.425074014063,1.10974719909899,152.042776226069));
#86043=CARTESIAN_POINT('Ctrl Pts',(110.491771329291,1.06925349349879,151.989678218464));
#86044=CARTESIAN_POINT('Ctrl Pts',(110.537415615272,1.04154163924302,151.953340614231));
#86045=CARTESIAN_POINT('Ctrl Pts',(110.58205524589,1.01461277564984,151.915244580614));
#86046=CARTESIAN_POINT('Ctrl Pts',(110.62530262364,0.988680169120933,151.875465066187));
#86047=CARTESIAN_POINT('Ctrl Pts',(110.629563036415,0.986125479938043,151.871546281737));
#86048=CARTESIAN_POINT('Ctrl Pts',(110.633811274977,0.983579621774255,151.867610985757));
#86049=CARTESIAN_POINT('Ctrl Pts',(110.638047119709,0.981042694525639,151.863658939861));
#86050=CARTESIAN_POINT('Ctrl Pts',(110.70070725821,0.943514356544463,151.805196989804));
#86051=CARTESIAN_POINT('Ctrl Pts',(110.760624068134,0.907958530544358,151.743130385674));
#86052=CARTESIAN_POINT('Ctrl Pts',(110.817254839353,0.874600052649044,151.676514300529));
#86053=CARTESIAN_POINT('Ctrl Pts',(110.85673195265,0.851345973939509,151.630076459685));
#86054=CARTESIAN_POINT('Ctrl Pts',(110.894611970937,0.82915999987308,151.581427616684));
#86055=CARTESIAN_POINT('Ctrl Pts',(110.93070160126,0.808125250386176,151.53023744095));
#86056=CARTESIAN_POINT('Ctrl Pts',(110.933778433361,0.806331926601132,151.525873207387));
#86057=CARTESIAN_POINT('Ctrl Pts',(110.936838861941,0.804548941091073,151.521495117895));
#86058=CARTESIAN_POINT('Ctrl Pts',(110.939882620671,0.802776422030424,151.517103032953));
#86059=CARTESIAN_POINT('Ctrl Pts',(110.980020267636,0.779402445768727,151.459185185155));
#86060=CARTESIAN_POINT('Ctrl Pts',(111.017089051938,0.757947186283859,151.39911365981));
#86061=CARTESIAN_POINT('Ctrl Pts',(111.050594740143,0.738635777139546,151.336542541543));
#86062=CARTESIAN_POINT('Ctrl Pts',(111.080229497341,0.72155542595697,151.281200299767));
#86063=CARTESIAN_POINT('Ctrl Pts',(111.107077475512,0.706152002360059,151.223902600443));
#86064=CARTESIAN_POINT('Ctrl Pts',(111.1307673688,0.692600311320128,151.164386072023));
#86065=CARTESIAN_POINT('Ctrl Pts',(111.139079110306,0.687845619033563,151.143504340159));
#86066=CARTESIAN_POINT('Ctrl Pts',(111.147001767321,0.683319072810068,151.122349238626));
#86067=CARTESIAN_POINT('Ctrl Pts',(111.154518126295,0.679028925038091,151.100908592914));
#86068=CARTESIAN_POINT('Ctrl Pts',(111.155644514676,0.678386011012504,151.097695535328));
#86069=CARTESIAN_POINT('Ctrl Pts',(111.156760455762,0.677749140970417,151.094479455626));
#86070=CARTESIAN_POINT('Ctrl Pts',(111.157865910725,0.677118333770718,151.091260344968));
#86071=CARTESIAN_POINT('Ctrl Pts',(111.178503113567,0.665342099939013,151.031164328541));
#86072=CARTESIAN_POINT('Ctrl Pts',(111.195422514671,0.655714867320027,150.970227054675));
#86073=CARTESIAN_POINT('Ctrl Pts',(111.208427711382,0.648327212263957,150.908408142258));
#86074=CARTESIAN_POINT('Ctrl Pts',(111.220857230375,0.641266573284417,150.849325656765));
#86075=CARTESIAN_POINT('Ctrl Pts',(111.229711584529,0.636251567041951,150.78943767752));
#86076=CARTESIAN_POINT('Ctrl Pts',(111.234779728312,0.633384247886193,150.728697997016));
#86077=CARTESIAN_POINT('Ctrl Pts',(111.238098863481,0.63150643615474,150.688919486701));
#86078=CARTESIAN_POINT('Ctrl Pts',(111.239793303854,0.630550224268599,150.648775470141));
#86079=CARTESIAN_POINT('Ctrl Pts',(111.239793308547,0.630550221611425,150.608250755187));
#86080=CARTESIAN_POINT('',(111.239793308547,0.630550221611421,41.));
#86081=CARTESIAN_POINT('',(111.239793308547,0.630550221611421,200.));
#86082=CARTESIAN_POINT('',(148.327056352437,8.62815343953651,41.));
#86083=CARTESIAN_POINT('Origin',(125.29348064571,25.4505574462982,41.));
#86084=CARTESIAN_POINT('',(148.327056352437,8.62815343953651,150.608250755186));
#86085=CARTESIAN_POINT('',(148.327056352437,8.62815343953651,200.));
#86086=CARTESIAN_POINT('',(150.023036902254,11.238311537975,152.608250755187));
#86087=CARTESIAN_POINT('Ctrl Pts',(148.327056352437,8.62815343953653,150.608250755186));
#86088=CARTESIAN_POINT('Ctrl Pts',(148.327056355648,8.62815344393261,150.653182845415));
#86089=CARTESIAN_POINT('Ctrl Pts',(148.328597783066,8.63025784593123,150.697882422423));
#86090=CARTESIAN_POINT('Ctrl Pts',(148.331544689823,8.63429111208799,150.742200419329));
#86091=CARTESIAN_POINT('Ctrl Pts',(148.334586530884,8.63845430950751,150.787946116039));
#86092=CARTESIAN_POINT('Ctrl Pts',(148.339126089743,8.6446729210104,150.833286146418));
#86093=CARTESIAN_POINT('Ctrl Pts',(148.345047922207,8.65280026655287,150.878059836472));
#86094=CARTESIAN_POINT('Ctrl Pts',(148.351129064247,8.66114625454908,150.924038031663));
#86095=CARTESIAN_POINT('Ctrl Pts',(148.358668143408,8.67150540995371,150.969420095879));
#86096=CARTESIAN_POINT('Ctrl Pts',(148.367571470274,8.68376212324061,151.014020080674));
#86097=CARTESIAN_POINT('Ctrl Pts',(148.373624358134,8.69209479620402,151.044341185425));
#86098=CARTESIAN_POINT('Ctrl Pts',(148.380308440668,8.70130540278121,151.074300568726));
#86099=CARTESIAN_POINT('Ctrl Pts',(148.387601113806,8.7113672249093,151.103832740569));
#86100=CARTESIAN_POINT('Ctrl Pts',(148.388415597221,8.71249098119087,151.107131046104));
#86101=CARTESIAN_POINT('Ctrl Pts',(148.389237458434,8.71362506083807,151.110423262381));
#86102=CARTESIAN_POINT('Ctrl Pts',(148.390066647454,8.71476940103632,151.113709253066));
#86103=CARTESIAN_POINT('Ctrl Pts',(148.410348874067,8.74276032549509,151.194085628184));
#86104=CARTESIAN_POINT('Ctrl Pts',(148.434884633381,8.77673358153417,151.271196363152));
#86105=CARTESIAN_POINT('Ctrl Pts',(148.462667315314,8.81542934375246,151.344668023511));
#86106=CARTESIAN_POINT('Ctrl Pts',(148.487557673704,8.85009667328186,151.410490896992));
#86107=CARTESIAN_POINT('Ctrl Pts',(148.515054073122,8.88855439426902,151.473392480735));
#86108=CARTESIAN_POINT('Ctrl Pts',(148.544415056844,8.92987551455189,151.533081539737));
#86109=CARTESIAN_POINT('Ctrl Pts',(148.546552570807,8.93288374044883,151.537426973061));
#86110=CARTESIAN_POINT('Ctrl Pts',(148.548699885631,8.93590702948339,151.541755336793));
#86111=CARTESIAN_POINT('Ctrl Pts',(148.55085670104,8.93894500455668,151.546066510681));
#86112=CARTESIAN_POINT('Ctrl Pts',(148.587783204918,8.9909577071013,151.619877453696));
#86113=CARTESIAN_POINT('Ctrl Pts',(148.627416081672,9.04719548373904,151.689016296417));
#86114=CARTESIAN_POINT('Ctrl Pts',(148.669115490153,9.10686606773614,151.753729104497));
#86115=CARTESIAN_POINT('Ctrl Pts',(148.712668400571,9.16918895657458,151.821318339832));
#86116=CARTESIAN_POINT('Ctrl Pts',(148.758475300866,9.23525621682179,151.884079380573));
#86117=CARTESIAN_POINT('Ctrl Pts',(148.805779372373,9.30412622234888,151.94232646711));
#86118=CARTESIAN_POINT('Ctrl Pts',(148.857157944997,9.37892829472724,152.00559062325));
#86119=CARTESIAN_POINT('Ctrl Pts',(148.91030228072,9.45703626517374,152.06352962054));
#86120=CARTESIAN_POINT('Ctrl Pts',(148.964216374769,9.53720504806013,152.116585972851));
#86121=CARTESIAN_POINT('Ctrl Pts',(148.975223846884,9.55357285795584,152.127418322515));
#86122=CARTESIAN_POINT('Ctrl Pts',(148.986263339059,9.57002646799165,152.138047268404));
#86123=CARTESIAN_POINT('Ctrl Pts',(148.997326284789,9.58655513910883,152.148476762181));
#86124=CARTESIAN_POINT('Ctrl Pts',(149.00027597909,9.59096215042319,152.151257560271));
#86125=CARTESIAN_POINT('Ctrl Pts',(149.003227532453,9.59537478430998,152.154024316336));
#86126=CARTESIAN_POINT('Ctrl Pts',(149.006180782728,9.59979283861002,152.156777099669));
#86127=CARTESIAN_POINT('Ctrl Pts',(149.065723470318,9.68886853571161,152.212278023329));
#86128=CARTESIAN_POINT('Ctrl Pts',(149.12656226372,9.78102167254516,152.262422515793));
#86129=CARTESIAN_POINT('Ctrl Pts',(149.188058090848,9.87538467355686,152.307308751997));
#86130=CARTESIAN_POINT('Ctrl Pts',(149.254297541489,9.97702658390632,152.355657392324));
#86131=CARTESIAN_POINT('Ctrl Pts',(149.321298638721,10.0812316646319,152.397904945431));
#86132=CARTESIAN_POINT('Ctrl Pts',(149.388246614364,10.1868826220101,152.434224145398));
#86133=CARTESIAN_POINT('Ctrl Pts',(149.429229226741,10.2515575011517,152.456457165587));
#86134=CARTESIAN_POINT('Ctrl Pts',(149.470191659495,10.3167736033849,152.476469621483));
#86135=CARTESIAN_POINT('Ctrl Pts',(149.510946200718,10.3822714058908,152.494309993715));
#86136=CARTESIAN_POINT('Ctrl Pts',(149.512747991317,10.3851671157005,152.495098730724));
#86137=CARTESIAN_POINT('Ctrl Pts',(149.51454941295,10.3880634359148,152.495883238571));
#86138=CARTESIAN_POINT('Ctrl Pts',(149.516350450608,10.3909603461317,152.496663521671));
#86139=CARTESIAN_POINT('Ctrl Pts',(149.686680714973,10.6649310101692,152.570457551552));
#86140=CARTESIAN_POINT('Ctrl Pts',(149.855757811428,10.9472429965344,152.608250749998));
#86141=CARTESIAN_POINT('Ctrl Pts',(150.023036902254,11.238311537975,152.608250755187));
#86142=CARTESIAN_POINT('',(153.775476116832,23.9291040663932,152.608250755187));
#86143=CARTESIAN_POINT('Origin',(125.29348064571,25.4505574462982,152.608250755187));
#86144=CARTESIAN_POINT('',(153.775476116832,23.9291040663932,184.081718857688));
#86145=CARTESIAN_POINT('',(153.775476116832,23.9291040663932,200.));
#86146=CARTESIAN_POINT('',(153.812479229218,24.9971192497139,186.033932954965));
#86147=CARTESIAN_POINT('Ctrl Pts',(153.775476116832,23.9291040663932,184.081718857688));
#86148=CARTESIAN_POINT('Ctrl Pts',(153.775476116833,23.9291040664218,184.18683784592));
#86149=CARTESIAN_POINT('Ctrl Pts',(153.775835918749,23.9356932216278,184.291821685737));
#86150=CARTESIAN_POINT('Ctrl Pts',(153.776527304571,23.9488156066092,184.395645925698));
#86151=CARTESIAN_POINT('Ctrl Pts',(153.777122987151,23.9601215603797,184.48509857161));
#86152=CARTESIAN_POINT('Ctrl Pts',(153.777964738683,23.9762763343269,184.573689668976));
#86153=CARTESIAN_POINT('Ctrl Pts',(153.779032729615,23.9972132828232,184.660762130601));
#86154=CARTESIAN_POINT('Ctrl Pts',(153.77905396866,23.9976296541279,184.662493733201));
#86155=CARTESIAN_POINT('Ctrl Pts',(153.779075297335,23.9980479198028,184.664224752928));
#86156=CARTESIAN_POINT('Ctrl Pts',(153.779096715495,23.9984680795417,184.665955185441));
#86157=CARTESIAN_POINT('Ctrl Pts',(153.780335726001,24.0227737306845,184.76605827737));
#86158=CARTESIAN_POINT('Ctrl Pts',(153.781891347461,24.0537766428393,184.86522683398));
#86159=CARTESIAN_POINT('Ctrl Pts',(153.783676643627,24.0912021740848,184.961913456917));
#86160=CARTESIAN_POINT('Ctrl Pts',(153.785213510754,24.1234198362054,185.04514586126));
#86161=CARTESIAN_POINT('Ctrl Pts',(153.786920623228,24.1603976715318,185.126539185878));
#86162=CARTESIAN_POINT('Ctrl Pts',(153.788742263954,24.2019772886183,185.205080004687));
#86163=CARTESIAN_POINT('Ctrl Pts',(153.788798993319,24.2032721571579,185.207525915508));
#86164=CARTESIAN_POINT('Ctrl Pts',(153.788855834083,24.204571498343,185.209969085199));
#86165=CARTESIAN_POINT('Ctrl Pts',(153.78891278456,24.2058753078926,185.212409482336));
#86166=CARTESIAN_POINT('Ctrl Pts',(153.790943205448,24.2523592400329,185.299415483266));
#86167=CARTESIAN_POINT('Ctrl Pts',(153.793125302327,24.3048539183938,185.383361160768));
#86168=CARTESIAN_POINT('Ctrl Pts',(153.795342394988,24.3629513380175,185.463342843834));
#86169=CARTESIAN_POINT('Ctrl Pts',(153.79741974315,24.4173868472074,185.538283240013));
#86170=CARTESIAN_POINT('Ctrl Pts',(153.799527849837,24.4767414351666,185.609743667113));
#86171=CARTESIAN_POINT('Ctrl Pts',(153.801567334367,24.540682359021,185.676939406521));
#86172=CARTESIAN_POINT('Ctrl Pts',(153.802750453586,24.5777749355041,185.715920124237));
#86173=CARTESIAN_POINT('Ctrl Pts',(153.803904141896,24.6162117466583,185.753262592201));
#86174=CARTESIAN_POINT('Ctrl Pts',(153.805012744829,24.6560073896456,185.788953519961));
#86175=CARTESIAN_POINT('Ctrl Pts',(153.806106344776,24.6952644687927,185.824161433962));
#86176=CARTESIAN_POINT('Ctrl Pts',(153.807156145169,24.7358442672836,185.857762680895));
#86177=CARTESIAN_POINT('Ctrl Pts',(153.808146151009,24.7777933705704,185.889706633511));
#86178=CARTESIAN_POINT('Ctrl Pts',(153.809105866949,24.8184590126162,185.920673239251));
#86179=CARTESIAN_POINT('Ctrl Pts',(153.81000945025,24.8604118596032,185.950082728695));
#86180=CARTESIAN_POINT('Ctrl Pts',(153.81084045852,24.9037190593713,185.97784759324));
#86181=CARTESIAN_POINT('Ctrl Pts',(153.811424818388,24.9341724139999,185.997371674011));
#86182=CARTESIAN_POINT('Ctrl Pts',(153.811973254734,24.965295980978,186.016081687442));
#86183=CARTESIAN_POINT('Ctrl Pts',(153.812479229218,24.9971192497139,186.033932954965));
#86184=CARTESIAN_POINT('',(153.816083724746,25.4505574462842,186.284526408638));
#86185=CARTESIAN_POINT('Origin',(133.440794228452,34.3467674767392,169.944726356503));
#86186=CARTESIAN_POINT('',(153.816083724746,25.4505574462982,199.));
#86187=CARTESIAN_POINT('',(153.816083724746,25.4505574462982,200.));
#86188=CARTESIAN_POINT('Origin',(125.29348064571,25.4505574462982,199.));
#86189=CARTESIAN_POINT('',(150.625700340104,38.5584761124776,190.698119455572));
#86190=CARTESIAN_POINT('Ctrl Pts',(153.816083724746,25.4505574462982,186.284526408646));
#86191=CARTESIAN_POINT('Ctrl Pts',(153.816083724746,26.5106419398841,186.861657876856));
#86192=CARTESIAN_POINT('Ctrl Pts',(153.757166391213,27.588785058979,187.388187067696));
#86193=CARTESIAN_POINT('Ctrl Pts',(153.569780012624,29.2312207216284,188.104076474668));
#86194=CARTESIAN_POINT('Ctrl Pts',(153.490782930083,29.7829196479227,188.330345814086));
#86195=CARTESIAN_POINT('Ctrl Pts',(153.297393809188,30.8946428510959,188.757964813333));
#86196=CARTESIAN_POINT('Ctrl Pts',(153.182766552402,31.4549710261938,188.959285999996));
#86197=CARTESIAN_POINT('Ctrl Pts',(152.788570289629,33.1228706277751,189.517224242465));
#86198=CARTESIAN_POINT('Ctrl Pts',(152.457618579669,34.2256840028288,189.831355971386));
#86199=CARTESIAN_POINT('Ctrl Pts',(151.652438549957,36.4095069388551,190.348448095162));
#86200=CARTESIAN_POINT('Ctrl Pts',(151.178289930999,37.4905475363332,190.551395655298));
#86201=CARTESIAN_POINT('Ctrl Pts',(150.625700340104,38.5584761124776,190.698119455572));
#86202=CARTESIAN_POINT('',(127.30024332107,53.9024781190581,194.634660522392));
#86203=CARTESIAN_POINT('Ctrl Pts',(150.625700340104,38.5584761124776,190.698119455572));
#86204=CARTESIAN_POINT('Ctrl Pts',(150.061469174662,39.6489030677709,190.847934331189));
#86205=CARTESIAN_POINT('Ctrl Pts',(149.431181026365,40.695257042216,191.009583714252));
#86206=CARTESIAN_POINT('Ctrl Pts',(148.735694662152,41.6986800582058,191.179338039736));
#86207=CARTESIAN_POINT('Ctrl Pts',(148.735673295998,41.6987108845328,191.179343254787));
#86208=CARTESIAN_POINT('Ctrl Pts',(148.73565192978,41.698741710823,191.179348469846));
#86209=CARTESIAN_POINT('Ctrl Pts',(148.735630563497,41.6987725370764,191.179353684914));
#86210=CARTESIAN_POINT('Ctrl Pts',(148.387874587815,42.20049826009,191.2642337292));
#86211=CARTESIAN_POINT('Ctrl Pts',(148.022946011743,42.6924701456368,191.35134309563));
#86212=CARTESIAN_POINT('Ctrl Pts',(147.643370795097,43.1712035043443,191.439657777885));
#86213=CARTESIAN_POINT('Ctrl Pts',(147.643369837125,43.1712047125725,191.439658000774));
#86214=CARTESIAN_POINT('Ctrl Pts',(147.643368879152,43.1712059208007,191.439658223663));
#86215=CARTESIAN_POINT('Ctrl Pts',(147.643367921179,43.1712071290287,191.439658446552));
#86216=CARTESIAN_POINT('Ctrl Pts',(147.263793588568,43.6499392126947,191.527972912004));
#86217=CARTESIAN_POINT('Ctrl Pts',(146.870881838364,44.1139344808582,191.617196054609));
#86218=CARTESIAN_POINT('Ctrl Pts',(146.464931838332,44.5636037969635,191.70694380284));
#86219=CARTESIAN_POINT('Ctrl Pts',(146.464890465031,44.5636496260163,191.706952949682));
#86220=CARTESIAN_POINT('Ctrl Pts',(146.464849091595,44.5636954549204,191.70696209653));
#86221=CARTESIAN_POINT('Ctrl Pts',(146.464807718023,44.5637412836756,191.706971243383));
#86222=CARTESIAN_POINT('Ctrl Pts',(145.652941727099,45.4630305166459,191.886458259871));
#86223=CARTESIAN_POINT('Ctrl Pts',(144.789083501741,46.3052025359163,192.067991850579));
#86224=CARTESIAN_POINT('Ctrl Pts',(143.873620601989,47.0911971228637,192.249227483336));
#86225=CARTESIAN_POINT('Ctrl Pts',(143.873463960051,47.0913316118918,192.249258493987));
#86226=CARTESIAN_POINT('Ctrl Pts',(143.873307316601,47.0914660992751,192.24928950463));
#86227=CARTESIAN_POINT('Ctrl Pts',(143.873150671641,47.0916005850136,192.249320515264));
#86228=CARTESIAN_POINT('Ctrl Pts',(142.957780102958,47.8774815154557,192.430534271331));
#86229=CARTESIAN_POINT('Ctrl Pts',(141.990826816845,48.6072058722179,192.611464291541));
#86230=CARTESIAN_POINT('Ctrl Pts',(140.970103221489,49.2787422497132,192.790511107359));
#86231=CARTESIAN_POINT('Ctrl Pts',(140.969808649731,49.2789360491434,192.790562778679));
#86232=CARTESIAN_POINT('Ctrl Pts',(140.969514073494,49.2791298437284,192.790614449842));
#86233=CARTESIAN_POINT('Ctrl Pts',(140.969219492776,49.2793236334683,192.790666120848));
#86234=CARTESIAN_POINT('Ctrl Pts',(140.459049412573,49.6149386998141,192.880152635069));
#86235=CARTESIAN_POINT('Ctrl Pts',(139.938175750855,49.9340294827454,192.968677353463));
#86236=CARTESIAN_POINT('Ctrl Pts',(139.410618693711,50.2345300845201,193.055482746109));
#86237=CARTESIAN_POINT('Ctrl Pts',(139.410267290937,50.2347302462726,193.055540566691));
#86238=CARTESIAN_POINT('Ctrl Pts',(139.409915885195,50.2349303997783,193.05559838651));
#86239=CARTESIAN_POINT('Ctrl Pts',(139.409564476487,50.2351305450365,193.055656205566));
#86240=CARTESIAN_POINT('Ctrl Pts',(138.882045294331,50.5355797384922,193.142451611038));
#86241=CARTESIAN_POINT('Ctrl Pts',(138.346664242735,50.8182249900564,193.227736381437));
#86242=CARTESIAN_POINT('Ctrl Pts',(137.803522272346,51.0833049561888,193.311458624612));
#86243=CARTESIAN_POINT('Ctrl Pts',(137.803136062597,51.0834934455209,193.311518156646));
#86244=CARTESIAN_POINT('Ctrl Pts',(137.802749848923,51.0836819259721,193.311577687891));
#86245=CARTESIAN_POINT('Ctrl Pts',(137.802363631325,51.0838703975427,193.311637218346));
#86246=CARTESIAN_POINT('Ctrl Pts',(136.715720182944,51.6141450354221,193.479129271527));
#86247=CARTESIAN_POINT('Ctrl Pts',(135.598096689337,52.0743333349272,193.640350049973));
#86248=CARTESIAN_POINT('Ctrl Pts',(134.449176632172,52.4637415868922,193.795169694551));
#86249=CARTESIAN_POINT('Ctrl Pts',(134.448795563475,52.4638707440901,193.795221044443));
#86250=CARTESIAN_POINT('Ctrl Pts',(134.448414491335,52.4639998935016,193.79527239363));
#86251=CARTESIAN_POINT('Ctrl Pts',(134.448033415752,52.4641290351266,193.795323742113));
#86252=CARTESIAN_POINT('Ctrl Pts',(133.873739902698,52.6587497372968,193.872707605266));
#86253=CARTESIAN_POINT('Ctrl Pts',(133.291604977981,52.8356331717541,193.948497219751));
#86254=CARTESIAN_POINT('Ctrl Pts',(132.701448837108,52.9943569968444,194.022701543398));
#86255=CARTESIAN_POINT('Ctrl Pts',(132.701112354813,52.9944474945164,194.022743851593));
#86256=CARTESIAN_POINT('Ctrl Pts',(132.700775869911,52.9945379862852,194.022786159272));
#86257=CARTESIAN_POINT('Ctrl Pts',(132.7004393824,52.9946284721507,194.022828466437));
#86258=CARTESIAN_POINT('Ctrl Pts',(132.110218972949,53.1533464123654,194.097037912924));
#86259=CARTESIAN_POINT('Ctrl Pts',(131.511183281109,53.2939014558829,194.169734986987));
#86260=CARTESIAN_POINT('Ctrl Pts',(130.912612387922,53.4141810466492,194.239880283632));
#86261=CARTESIAN_POINT('Ctrl Pts',(130.912355373884,53.4142326922331,194.23991040258));
#86262=CARTESIAN_POINT('Ctrl Pts',(130.912098359931,53.4142843340791,194.239940521058));
#86263=CARTESIAN_POINT('Ctrl Pts',(130.911841346064,53.414335972187,194.239970639066));
#86264=CARTESIAN_POINT('Ctrl Pts',(129.714274871677,53.6549458171522,194.380306710062));
#86265=CARTESIAN_POINT('Ctrl Pts',(128.510331618815,53.8171285197205,194.51151055066));
#86266=CARTESIAN_POINT('Ctrl Pts',(127.30024332107,53.9024781190581,194.634660522392));
#86267=CARTESIAN_POINT('',(123.286717970418,53.9024781190629,195.01289889797));
#86268=CARTESIAN_POINT('Ctrl Pts',(127.30024332107,53.9024781190581,194.634660522392));
#86269=CARTESIAN_POINT('Ctrl Pts',(126.632621052928,53.949566660614,194.702604046515));
#86270=CARTESIAN_POINT('Ctrl Pts',(125.963635221528,53.9731507806434,194.765349588697));
#86271=CARTESIAN_POINT('Ctrl Pts',(124.624155818791,53.9731702639907,194.891453422566));
#86272=CARTESIAN_POINT('Ctrl Pts',(123.955253370733,53.9496310653927,194.954665574162));
#86273=CARTESIAN_POINT('Ctrl Pts',(123.286717970418,53.9024781190629,195.01289889797));
#86274=CARTESIAN_POINT('',(96.9910158671794,28.9874167683923,196.445393189885));
#86275=CARTESIAN_POINT('Ctrl Pts',(123.286717970418,53.9024781190629,195.01289889797));
#86276=CARTESIAN_POINT('Ctrl Pts',(123.051828692201,53.8859109761352,195.033359121005));
#86277=CARTESIAN_POINT('Ctrl Pts',(122.816379187764,53.8663568090316,195.05358701849));
#86278=CARTESIAN_POINT('Ctrl Pts',(122.581140823996,53.8438729171098,195.073525055871));
#86279=CARTESIAN_POINT('Ctrl Pts',(122.407062679345,53.827234669302,195.08827935232));
#86280=CARTESIAN_POINT('Ctrl Pts',(122.233100354408,53.8089931799125,195.102875013651));
#86281=CARTESIAN_POINT('Ctrl Pts',(122.059565244225,53.7891899052099,195.117290547141));
#86282=CARTESIAN_POINT('Ctrl Pts',(121.77966601252,53.757248695338,195.140541730975));
#86283=CARTESIAN_POINT('Ctrl Pts',(121.500846574299,53.7212485547933,195.1633276292));
#86284=CARTESIAN_POINT('Ctrl Pts',(121.223097074563,53.6812169890033,195.1856676816));
#86285=CARTESIAN_POINT('Ctrl Pts',(121.095940822165,53.6628901733355,195.195895161197));
#86286=CARTESIAN_POINT('Ctrl Pts',(120.969008930784,53.6437177097922,195.206029122082));
#86287=CARTESIAN_POINT('Ctrl Pts',(120.842301392603,53.6236987276649,195.216071038628));
#86288=CARTESIAN_POINT('Ctrl Pts',(120.842169588707,53.6236779034908,195.216081484445));
#86289=CARTESIAN_POINT('Ctrl Pts',(120.842037785115,53.6236570784102,195.216091930157));
#86290=CARTESIAN_POINT('Ctrl Pts',(120.841905981827,53.6236362524229,195.216102375765));
#86291=CARTESIAN_POINT('Ctrl Pts',(120.03508769286,53.4961524272351,195.280043932537));
#86292=CARTESIAN_POINT('Ctrl Pts',(119.237312586138,53.3346392699969,195.340284676336));
#86293=CARTESIAN_POINT('Ctrl Pts',(118.448469507687,53.139629459016,195.397278038018));
#86294=CARTESIAN_POINT('Ctrl Pts',(118.448244786133,53.1395739056253,195.397294273993));
#86295=CARTESIAN_POINT('Ctrl Pts',(118.448020065304,53.1395183495163,195.397310509705));
#86296=CARTESIAN_POINT('Ctrl Pts',(118.4477953452,53.1394627906889,195.397326745153));
#86297=CARTESIAN_POINT('Ctrl Pts',(116.870086353624,52.7493968376374,195.511312153296));
#86298=CARTESIAN_POINT('Ctrl Pts',(115.327903406651,52.2260862500057,195.612365054023));
#86299=CARTESIAN_POINT('Ctrl Pts',(113.822703841679,51.5649244867685,195.703261304229));
#86300=CARTESIAN_POINT('Ctrl Pts',(113.822385722138,51.5647847521568,195.703280514886));
#86301=CARTESIAN_POINT('Ctrl Pts',(113.822067604247,51.5646450113871,195.70329972509));
#86302=CARTESIAN_POINT('Ctrl Pts',(113.821749488008,51.5645052644595,195.703318934841));
#86303=CARTESIAN_POINT('Ctrl Pts',(113.44571802119,51.3993164571522,195.726025951065));
#86304=CARTESIAN_POINT('Ctrl Pts',(113.071361950894,51.2251071050355,195.748130225883));
#86305=CARTESIAN_POINT('Ctrl Pts',(112.702797713323,51.0437907256687,195.769437135944));
#86306=CARTESIAN_POINT('Ctrl Pts',(112.702474366697,51.0436316542412,195.769455828798));
#86307=CARTESIAN_POINT('Ctrl Pts',(112.702151024526,51.0434725773416,195.769474521039));
#86308=CARTESIAN_POINT('Ctrl Pts',(112.701827686811,51.0433134949714,195.769493212665));
#86309=CARTESIAN_POINT('Ctrl Pts',(112.333285153187,50.8619903238695,195.790798056524));
#86310=CARTESIAN_POINT('Ctrl Pts',(111.969800119671,50.6732726224591,195.811351687744));
#86311=CARTESIAN_POINT('Ctrl Pts',(111.611298768909,50.4772788755021,195.831212048309));
#86312=CARTESIAN_POINT('Ctrl Pts',(111.610976846822,50.4771028797467,195.831229882241));
#86313=CARTESIAN_POINT('Ctrl Pts',(111.610654928752,50.4769268781238,195.831247715614));
#86314=CARTESIAN_POINT('Ctrl Pts',(111.610333014701,50.4767508706336,195.831265548428));
#86315=CARTESIAN_POINT('Ctrl Pts',(110.893041082789,50.0845693177917,195.871000793435));
#86316=CARTESIAN_POINT('Ctrl Pts',(110.195668715804,49.6632963076804,195.907966652454));
#86317=CARTESIAN_POINT('Ctrl Pts',(109.517936153566,49.2133662529799,195.942552628765));
#86318=CARTESIAN_POINT('Ctrl Pts',(109.517627457568,49.213161317265,195.942568382106));
#86319=CARTESIAN_POINT('Ctrl Pts',(109.517318765645,49.2129563756048,195.942584134954));
#86320=CARTESIAN_POINT('Ctrl Pts',(109.517010077796,49.2127514279993,195.942599887308));
#86321=CARTESIAN_POINT('Ctrl Pts',(108.161281119207,48.3126401828122,196.011782793513));
#86322=CARTESIAN_POINT('Ctrl Pts',(106.883700856073,47.2985001737882,196.071502648147));
#86323=CARTESIAN_POINT('Ctrl Pts',(105.687270783624,46.1661414654911,196.123962833256));
#86324=CARTESIAN_POINT('Ctrl Pts',(105.687018511028,46.1659027026272,196.123973894719));
#86325=CARTESIAN_POINT('Ctrl Pts',(105.68676624204,46.1656639345064,196.123984955859));
#86326=CARTESIAN_POINT('Ctrl Pts',(105.686513976658,46.1654251611288,196.123996016677));
#86327=CARTESIAN_POINT('Ctrl Pts',(105.387599175031,45.8824973320413,196.13710222288));
#86328=CARTESIAN_POINT('Ctrl Pts',(105.093849245306,45.5921177194927,196.149746269813));
#86329=CARTESIAN_POINT('Ctrl Pts',(104.808073524937,45.2971435883637,196.161843863493));
#86330=CARTESIAN_POINT('Ctrl Pts',(104.807841819524,45.2969044249286,196.161853672157));
#86331=CARTESIAN_POINT('Ctrl Pts',(104.80761011935,45.29666525847,196.161863480461));
#86332=CARTESIAN_POINT('Ctrl Pts',(104.807378424416,45.2964260889894,196.161873288407));
#86333=CARTESIAN_POINT('Ctrl Pts',(104.521606158111,45.0014347250463,196.17397039717));
#86334=CARTESIAN_POINT('Ctrl Pts',(104.243057792459,44.7011568357949,196.185554290362));
#86335=CARTESIAN_POINT('Ctrl Pts',(103.971628652771,44.3956759203509,196.196665129066));
#86336=CARTESIAN_POINT('Ctrl Pts',(103.971418658918,44.3954395820027,196.196673725077));
#86337=CARTESIAN_POINT('Ctrl Pts',(103.971208669325,44.3952032405395,196.196682320804));
#86338=CARTESIAN_POINT('Ctrl Pts',(103.970998683993,44.3949668959614,196.196690916249));
#86339=CARTESIAN_POINT('Ctrl Pts',(103.427932303613,43.7837299434221,196.218920549917));
#86340=CARTESIAN_POINT('Ctrl Pts',(102.913323228656,43.1516872362662,196.239261316819));
#86341=CARTESIAN_POINT('Ctrl Pts',(102.426794049151,42.4991213301067,196.257972789619));
#86342=CARTESIAN_POINT('Ctrl Pts',(102.426626494949,42.4988965950563,196.257979233602));
#86343=CARTESIAN_POINT('Ctrl Pts',(102.426458944077,42.4986718575718,196.257985677392));
#86344=CARTESIAN_POINT('Ctrl Pts',(102.426291396536,42.4984471176532,196.257992120989));
#86345=CARTESIAN_POINT('Ctrl Pts',(101.453063032674,41.1930071125781,196.295420847925));
#86346=CARTESIAN_POINT('Ctrl Pts',(100.591557999332,39.8059105229358,196.326383225952));
#86347=CARTESIAN_POINT('Ctrl Pts',(99.8463073435662,38.3338899863526,196.352178614945));
#86348=CARTESIAN_POINT('Ctrl Pts',(99.8462171346804,38.333711805587,196.352181737349));
#86349=CARTESIAN_POINT('Ctrl Pts',(99.846126927498,38.333533623577,196.352184859677));
#86350=CARTESIAN_POINT('Ctrl Pts',(99.8460367220189,38.3333554403228,196.352187981929));
#86351=CARTESIAN_POINT('Ctrl Pts',(99.4734515242212,37.5973863649595,196.365084149053));
#86352=CARTESIAN_POINT('Ctrl Pts',(99.1340435629579,36.8475297378679,196.376538124842));
#86353=CARTESIAN_POINT('Ctrl Pts',(98.8291431339836,36.0890595245597,196.386657820445));
#86354=CARTESIAN_POINT('Ctrl Pts',(98.8290868940062,36.0889196220092,196.38665968706));
#86355=CARTESIAN_POINT('Ctrl Pts',(98.8290306552028,36.0887797191656,196.386661553628));
#86356=CARTESIAN_POINT('Ctrl Pts',(98.8289744175735,36.0886398160288,196.386663420152));
#86357=CARTESIAN_POINT('Ctrl Pts',(98.5240691405042,35.3301226957862,196.396783206952));
#86358=CARTESIAN_POINT('Ctrl Pts',(98.252880212789,34.5614226416425,196.405595343169));
#86359=CARTESIAN_POINT('Ctrl Pts',(98.0150109184552,33.7826625670746,196.413227915146));
#86360=CARTESIAN_POINT('Ctrl Pts',(98.0149812430995,33.7825654129534,196.413228867347));
#86361=CARTESIAN_POINT('Ctrl Pts',(98.0149515682624,33.7824682586759,196.413229819529));
#86362=CARTESIAN_POINT('Ctrl Pts',(98.0149218939439,33.7823711042421,196.413230771693));
#86363=CARTESIAN_POINT('Ctrl Pts',(97.6450275225364,32.5713280160703,196.425099622736));
#86364=CARTESIAN_POINT('Ctrl Pts',(97.3552447935968,31.3360957625847,196.434146130749));
#86365=CARTESIAN_POINT('Ctrl Pts',(97.1483025685318,30.0758530500492,196.440544914249));
#86366=CARTESIAN_POINT('Ctrl Pts',(97.0890634582333,29.715097012816,196.442376624725));
#86367=CARTESIAN_POINT('Ctrl Pts',(97.036612966678,29.3522914170678,196.44399135908));
#86368=CARTESIAN_POINT('Ctrl Pts',(96.9910158671796,28.9874167683946,196.445393189885));
#86369=CARTESIAN_POINT('',(96.7715712560824,25.6494824928011,196.263237066376));
#86370=CARTESIAN_POINT('Ctrl Pts',(96.9910158671794,28.9874167683923,196.445393189885));
#86371=CARTESIAN_POINT('Ctrl Pts',(96.8801655539068,28.1003763742528,196.448801156303));
#86372=CARTESIAN_POINT('Ctrl Pts',(96.81145956153,27.2127811520719,196.411604298023));
#86373=CARTESIAN_POINT('Ctrl Pts',(96.7842616286642,26.3247722192935,196.33198398003));
#86374=CARTESIAN_POINT('Ctrl Pts',(96.777368162748,26.0997014633065,196.311803771812));
#86375=CARTESIAN_POINT('Ctrl Pts',(96.7731413589317,25.8746041252277,196.288898122989));
#86376=CARTESIAN_POINT('Ctrl Pts',(96.7715712560824,25.6494824928014,196.263237066376));
#86377=CARTESIAN_POINT('Origin',(96.8900428237467,25.8589582227839,194.418219598777));
#86378=CARTESIAN_POINT('Origin',(125.29348064571,25.4505574462982,199.));
#86379=CARTESIAN_POINT('',(152.816083724746,25.4505574462982,200.));
#86380=CARTESIAN_POINT('Origin',(152.816083724746,25.4505574462982,199.));
#86381=CARTESIAN_POINT('Origin',(125.29348064571,25.4505574462982,200.));
#86382=CARTESIAN_POINT('Origin',(-34.5950649486897,26.6830679909832,173.608250755187));
#86383=CARTESIAN_POINT('',(-18.1943440740468,24.8757620423259,173.608250755187));
#86384=CARTESIAN_POINT('',(-50.9957858233326,24.8757620423259,173.608250755187));
#86385=CARTESIAN_POINT('Origin',(-34.5950649486897,26.6830679909832,173.608250755187));
#86386=CARTESIAN_POINT('',(-50.9957858233326,24.8757620423259,152.608250755187));
#86387=CARTESIAN_POINT('',(-50.9957858233326,24.8757620423259,173.608250755187));
#86388=CARTESIAN_POINT('',(-50.8544940072586,23.8757620423259,151.608250755187));
#86389=CARTESIAN_POINT('Ctrl Pts',(-50.9957858233326,24.8757620423259,152.608250755187));
#86390=CARTESIAN_POINT('Ctrl Pts',(-50.9957858233326,24.8757620423259,152.482802647827));
#86391=CARTESIAN_POINT('Ctrl Pts',(-50.9930852122888,24.8507057023964,152.349039676494));
#86392=CARTESIAN_POINT('Ctrl Pts',(-50.9814007950441,24.7490003445042,152.103116732228));
#86393=CARTESIAN_POINT('Ctrl Pts',(-50.9723338669737,24.6723550602491,151.990959171534));
#86394=CARTESIAN_POINT('Ctrl Pts',(-50.9495732713337,24.4948810766518,151.812827976054));
#86395=CARTESIAN_POINT('Ctrl Pts',(-50.9342825703181,24.3818609440281,151.735479916628));
#86396=CARTESIAN_POINT('Ctrl Pts',(-50.897590189515,24.1348809622359,151.633200800084));
#86397=CARTESIAN_POINT('Ctrl Pts',(-50.8761070582787,24.0009410845208,151.608250755187));
#86398=CARTESIAN_POINT('Ctrl Pts',(-50.8544940072586,23.8757620423259,151.608250755187));
#86399=CARTESIAN_POINT('',(-18.3356358901209,23.8757620423259,151.608250755187));
#86400=CARTESIAN_POINT('Origin',(-34.5950649486897,26.6830679909832,151.608250755187));
#86401=CARTESIAN_POINT('',(-18.1943440740468,24.8757620423259,152.608250755187));
#86402=CARTESIAN_POINT('Ctrl Pts',(-18.3356358901209,23.8757620423259,151.608250755187));
#86403=CARTESIAN_POINT('Ctrl Pts',(-18.3140228391008,24.0009410845208,151.608250755187));
#86404=CARTESIAN_POINT('Ctrl Pts',(-18.2925397078645,24.1348809622359,151.633200800084));
#86405=CARTESIAN_POINT('Ctrl Pts',(-18.2558473270613,24.3818609440281,151.735479916628));
#86406=CARTESIAN_POINT('Ctrl Pts',(-18.2405566260457,24.4948810766518,151.812827976054));
#86407=CARTESIAN_POINT('Ctrl Pts',(-18.2177960304058,24.6723550602491,151.990959171534));
#86408=CARTESIAN_POINT('Ctrl Pts',(-18.2087291023353,24.7490003445041,152.103116732228));
#86409=CARTESIAN_POINT('Ctrl Pts',(-18.1970446850907,24.8507057023964,152.349039676494));
#86410=CARTESIAN_POINT('Ctrl Pts',(-18.1943440740468,24.8757620423259,152.482802647827));
#86411=CARTESIAN_POINT('Ctrl Pts',(-18.1943440740468,24.8757620423259,152.608250755187));
#86412=CARTESIAN_POINT('',(-18.1943440740468,24.8757620423259,173.608250755187));
#86413=CARTESIAN_POINT('Origin',(35.4049350513103,26.6830679909832,173.608250755187));
#86414=CARTESIAN_POINT('',(51.8056559259532,24.8757620423259,173.608250755187));
#86415=CARTESIAN_POINT('',(19.0042141766674,24.8757620423259,173.608250755187));
#86416=CARTESIAN_POINT('Origin',(35.4049350513103,26.6830679909832,173.608250755187));
#86417=CARTESIAN_POINT('',(19.0042141766674,24.8757620423259,152.608250755187));
#86418=CARTESIAN_POINT('',(19.0042141766674,24.8757620423259,173.608250755187));
#86419=CARTESIAN_POINT('',(19.1455059927414,23.8757620423259,151.608250755187));
#86420=CARTESIAN_POINT('Ctrl Pts',(19.0042141766674,24.8757620423259,152.608250755187));
#86421=CARTESIAN_POINT('Ctrl Pts',(19.0042141766674,24.8757620423259,152.482802647827));
#86422=CARTESIAN_POINT('Ctrl Pts',(19.0069147877113,24.8507057023964,152.349039676494));
#86423=CARTESIAN_POINT('Ctrl Pts',(19.0185992049559,24.7490003445042,152.103116732228));
#86424=CARTESIAN_POINT('Ctrl Pts',(19.0276661330263,24.6723550602491,151.990959171534));
#86425=CARTESIAN_POINT('Ctrl Pts',(19.0504267286663,24.4948810766518,151.812827976054));
#86426=CARTESIAN_POINT('Ctrl Pts',(19.0657174296819,24.3818609440281,151.735479916628));
#86427=CARTESIAN_POINT('Ctrl Pts',(19.102409810485,24.1348809622359,151.633200800084));
#86428=CARTESIAN_POINT('Ctrl Pts',(19.1238929417213,24.0009410845208,151.608250755187));
#86429=CARTESIAN_POINT('Ctrl Pts',(19.1455059927414,23.8757620423259,151.608250755187));
#86430=CARTESIAN_POINT('',(51.6643641098791,23.8757620423259,151.608250755187));
#86431=CARTESIAN_POINT('Origin',(35.4049350513103,26.6830679909832,151.608250755187));
#86432=CARTESIAN_POINT('',(51.8056559259533,24.8757620423259,152.608250755187));
#86433=CARTESIAN_POINT('Ctrl Pts',(51.6643641098791,23.8757620423259,151.608250755187));
#86434=CARTESIAN_POINT('Ctrl Pts',(51.6859771608993,24.0009410845208,151.608250755187));
#86435=CARTESIAN_POINT('Ctrl Pts',(51.7074602921355,24.1348809622359,151.633200800084));
#86436=CARTESIAN_POINT('Ctrl Pts',(51.7441526729387,24.3818609440281,151.735479916628));
#86437=CARTESIAN_POINT('Ctrl Pts',(51.7594433739543,24.4948810766518,151.812827976054));
#86438=CARTESIAN_POINT('Ctrl Pts',(51.7822039695942,24.6723550602491,151.990959171534));
#86439=CARTESIAN_POINT('Ctrl Pts',(51.7912708976647,24.7490003445041,152.103116732228));
#86440=CARTESIAN_POINT('Ctrl Pts',(51.8029553149093,24.8507057023964,152.349039676494));
#86441=CARTESIAN_POINT('Ctrl Pts',(51.8056559259532,24.8757620423259,152.482802647827));
#86442=CARTESIAN_POINT('Ctrl Pts',(51.8056559259532,24.8757620423259,152.608250755187));
#86443=CARTESIAN_POINT('',(51.8056559259532,24.8757620423259,173.608250755187));
#86444=CARTESIAN_POINT('Origin',(-104.59506494869,26.6830679909832,173.608250755187));
#86445=CARTESIAN_POINT('',(-88.1943440740468,24.8757620423259,173.608250755187));
#86446=CARTESIAN_POINT('',(-120.995785823333,24.8757620423259,173.608250755187));
#86447=CARTESIAN_POINT('Origin',(-104.59506494869,26.6830679909832,173.608250755187));
#86448=CARTESIAN_POINT('',(-120.995785823333,24.8757620423259,152.608250755187));
#86449=CARTESIAN_POINT('',(-120.995785823333,24.8757620423259,173.608250755187));
#86450=CARTESIAN_POINT('',(-120.854494007259,23.8757620423259,151.608250755187));
#86451=CARTESIAN_POINT('Ctrl Pts',(-120.995785823333,24.8757620423259,152.608250755187));
#86452=CARTESIAN_POINT('Ctrl Pts',(-120.995785823333,24.8757620423259,152.482802647827));
#86453=CARTESIAN_POINT('Ctrl Pts',(-120.993085212289,24.8507057023964,152.349039676494));
#86454=CARTESIAN_POINT('Ctrl Pts',(-120.981400795044,24.7490003445042,152.103116732228));
#86455=CARTESIAN_POINT('Ctrl Pts',(-120.972333866974,24.6723550602491,151.990959171534));
#86456=CARTESIAN_POINT('Ctrl Pts',(-120.949573271334,24.4948810766518,151.812827976054));
#86457=CARTESIAN_POINT('Ctrl Pts',(-120.934282570318,24.3818609440281,151.735479916628));
#86458=CARTESIAN_POINT('Ctrl Pts',(-120.897590189515,24.1348809622359,151.633200800084));
#86459=CARTESIAN_POINT('Ctrl Pts',(-120.876107058279,24.0009410845208,151.608250755187));
#86460=CARTESIAN_POINT('Ctrl Pts',(-120.854494007259,23.8757620423259,151.608250755187));
#86461=CARTESIAN_POINT('',(-88.3356358901209,23.8757620423259,151.608250755187));
#86462=CARTESIAN_POINT('Origin',(-104.59506494869,26.6830679909832,151.608250755187));
#86463=CARTESIAN_POINT('',(-88.1943440740468,24.8757620423259,152.608250755187));
#86464=CARTESIAN_POINT('Ctrl Pts',(-88.3356358901209,23.8757620423259,151.608250755187));
#86465=CARTESIAN_POINT('Ctrl Pts',(-88.3140228391008,24.0009410845208,151.608250755187));
#86466=CARTESIAN_POINT('Ctrl Pts',(-88.2925397078645,24.1348809622359,151.633200800084));
#86467=CARTESIAN_POINT('Ctrl Pts',(-88.2558473270613,24.3818609440281,151.735479916628));
#86468=CARTESIAN_POINT('Ctrl Pts',(-88.2405566260458,24.4948810766518,151.812827976054));
#86469=CARTESIAN_POINT('Ctrl Pts',(-88.2177960304058,24.6723550602491,151.990959171534));
#86470=CARTESIAN_POINT('Ctrl Pts',(-88.2087291023354,24.7490003445041,152.103116732228));
#86471=CARTESIAN_POINT('Ctrl Pts',(-88.1970446850907,24.8507057023964,152.349039676494));
#86472=CARTESIAN_POINT('Ctrl Pts',(-88.1943440740468,24.8757620423259,152.482802647827));
#86473=CARTESIAN_POINT('Ctrl Pts',(-88.1943440740468,24.8757620423259,152.608250755187));
#86474=CARTESIAN_POINT('',(-88.1943440740468,24.8757620423259,173.608250755187));
#86475=CARTESIAN_POINT('Origin',(-104.59506494869,26.6830679909832,171.608250755187));
#86476=CARTESIAN_POINT('',(-120.59506494869,26.6830679909832,152.108250755187));
#86477=CARTESIAN_POINT('',(-88.5950649486898,26.6830679909832,152.108250755187));
#86478=CARTESIAN_POINT('Origin',(-104.59506494869,26.6830679909832,152.108250755187));
#86479=CARTESIAN_POINT('',(-88.5950649486898,26.6830679909832,171.108250755187));
#86480=CARTESIAN_POINT('',(-88.5950649486898,26.6830679909832,171.608250755187));
#86481=CARTESIAN_POINT('',(-112.492659345135,12.768040044578,171.108250755187));
#86482=CARTESIAN_POINT('Origin',(-104.59506494869,26.6830679909832,171.108250755187));
#86483=CARTESIAN_POINT('',(-112.492659345135,12.768040044578,153.608250755187));
#86484=CARTESIAN_POINT('',(-112.492659345135,12.768040044578,171.608250755187));
#86485=CARTESIAN_POINT('',(-113.345699320966,13.2880540647967,152.608250755187));
#86486=CARTESIAN_POINT('Ctrl Pts',(-113.345699320966,13.2880540647967,152.608250755187));
#86487=CARTESIAN_POINT('Ctrl Pts',(-113.314805388695,13.2678718158554,152.60825075831));
#86488=CARTESIAN_POINT('Ctrl Pts',(-113.283882083917,13.247833572522,152.610400982822));
#86489=CARTESIAN_POINT('Ctrl Pts',(-113.253143854674,13.2280604794924,152.614563215046));
#86490=CARTESIAN_POINT('Ctrl Pts',(-113.221265174007,13.207553764109,152.618879874633));
#86491=CARTESIAN_POINT('Ctrl Pts',(-113.189584552444,13.1873316127548,152.625360599392));
#86492=CARTESIAN_POINT('Ctrl Pts',(-113.158319731925,13.1675195649457,152.633903745459));
#86493=CARTESIAN_POINT('Ctrl Pts',(-113.126367003894,13.147271600464,152.642634862998));
#86494=CARTESIAN_POINT('Ctrl Pts',(-113.094847362014,13.1274512359853,152.653520253598));
#86495=CARTESIAN_POINT('Ctrl Pts',(-113.063988424239,13.1081932943863,152.666504445662));
#86496=CARTESIAN_POINT('Ctrl Pts',(-113.051791630358,13.1005817185771,152.671636362887));
#86497=CARTESIAN_POINT('Ctrl Pts',(-113.039698098786,13.0930580740493,152.677096714824));
#86498=CARTESIAN_POINT('Ctrl Pts',(-113.027722336541,13.0856311228787,152.682884240715));
#86499=CARTESIAN_POINT('Ctrl Pts',(-113.026049232486,13.0845935219426,152.68369280161));
#86500=CARTESIAN_POINT('Ctrl Pts',(-113.024377683382,13.0835573316238,152.684508023839));
#86501=CARTESIAN_POINT('Ctrl Pts',(-113.022707717151,13.0825225645949,152.685329889022));
#86502=CARTESIAN_POINT('Ctrl Pts',(-112.972795707585,13.0515954111635,152.709893824593));
#86503=CARTESIAN_POINT('Ctrl Pts',(-112.924466199263,13.0220440815315,152.74032765976));
#86504=CARTESIAN_POINT('Ctrl Pts',(-112.878864738381,12.9944473172043,152.775796511354));
#86505=CARTESIAN_POINT('Ctrl Pts',(-112.837356246389,12.96932750637,152.808081848577));
#86506=CARTESIAN_POINT('Ctrl Pts',(-112.798108353315,12.9458272165739,152.844537973071));
#86507=CARTESIAN_POINT('Ctrl Pts',(-112.7619450575,12.9243594466032,152.884524370354));
#86508=CARTESIAN_POINT('Ctrl Pts',(-112.758379154776,12.9222426047144,152.888467252212));
#86509=CARTESIAN_POINT('Ctrl Pts',(-112.754843207173,12.9201455042233,152.892444455782));
#86510=CARTESIAN_POINT('Ctrl Pts',(-112.751337979856,12.9180685269604,152.896455365444));
#86511=CARTESIAN_POINT('Ctrl Pts',(-112.749642377971,12.917063819921,152.898395583685));
#86512=CARTESIAN_POINT('Ctrl Pts',(-112.747953361917,12.916063438456,152.900344344348));
#86513=CARTESIAN_POINT('Ctrl Pts',(-112.746270995886,12.9150674101679,152.902301551646));
#86514=CARTESIAN_POINT('Ctrl Pts',(-112.707269815393,12.89197714424,152.947674195699));
#86515=CARTESIAN_POINT('Ctrl Pts',(-112.67183902809,12.8712238657582,152.997605490933));
#86516=CARTESIAN_POINT('Ctrl Pts',(-112.640718851925,12.8531192060996,153.051009927998));
#86517=CARTESIAN_POINT('Ctrl Pts',(-112.609598675759,12.8350145464411,153.104414365064));
#86518=CARTESIAN_POINT('Ctrl Pts',(-112.582788322685,12.8195581462718,153.161292777412));
#86519=CARTESIAN_POINT('Ctrl Pts',(-112.561022072452,12.8070625461649,153.22061351513));
#86520=CARTESIAN_POINT('Ctrl Pts',(-112.56036537399,12.8066855477713,153.222403250928));
#86521=CARTESIAN_POINT('Ctrl Pts',(-112.559713246063,12.8063112214621,153.22419533454));
#86522=CARTESIAN_POINT('Ctrl Pts',(-112.559065695038,12.8059395694613,153.225989728665));
#86523=CARTESIAN_POINT('Ctrl Pts',(-112.546565934931,12.7987655234449,153.260627147536));
#86524=CARTESIAN_POINT('Ctrl Pts',(-112.53581288098,12.7926115974439,153.296006270051));
#86525=CARTESIAN_POINT('Ctrl Pts',(-112.526803176794,12.7874655986588,153.331953347758));
#86526=CARTESIAN_POINT('Ctrl Pts',(-112.517741491554,12.7822899102814,153.368107820401));
#86527=CARTESIAN_POINT('Ctrl Pts',(-112.510443061843,12.7781337002311,153.404837909206));
#86528=CARTESIAN_POINT('Ctrl Pts',(-112.504946453002,12.7750090296612,153.441987310219));
#86529=CARTESIAN_POINT('Ctrl Pts',(-112.499569035295,12.7719521159637,153.478331145599));
#86530=CARTESIAN_POINT('Ctrl Pts',(-112.495916044603,12.7698824718338,153.515077343027));
#86531=CARTESIAN_POINT('Ctrl Pts',(-112.494066058465,12.7688355319706,153.552083286413));
#86532=CARTESIAN_POINT('Ctrl Pts',(-112.493133072646,12.7683075388002,153.57074613999));
#86533=CARTESIAN_POINT('Ctrl Pts',(-112.492659348059,12.7680400462376,153.589475021945));
#86534=CARTESIAN_POINT('Ctrl Pts',(-112.492659345135,12.768040044578,153.608250755187));
#86535=CARTESIAN_POINT('',(-118.077578311569,18.0678585669597,152.608250755187));
#86536=CARTESIAN_POINT('Origin',(-104.59506494869,26.6830679909832,152.608250755187));
#86537=CARTESIAN_POINT('',(-118.588969902809,18.9260953769367,153.608250755187));
#86538=CARTESIAN_POINT('Ctrl Pts',(-118.588969902809,18.9260953769367,153.608250755187));
#86539=CARTESIAN_POINT('Ctrl Pts',(-118.588969902308,18.9260953760319,153.570920583163));
#86540=CARTESIAN_POINT('Ctrl Pts',(-118.587912104855,18.9241774989277,153.533707722385));
#86541=CARTESIAN_POINT('Ctrl Pts',(-118.58584346415,18.9204434093274,153.496805212604));
#86542=CARTESIAN_POINT('Ctrl Pts',(-118.584596475761,18.9181924788664,153.474560169703));
#86543=CARTESIAN_POINT('Ctrl Pts',(-118.582981660905,18.9152806425285,153.452427631481));
#86544=CARTESIAN_POINT('Ctrl Pts',(-118.581004941819,18.911722257265,153.430449466818));
#86545=CARTESIAN_POINT('Ctrl Pts',(-118.577602099565,18.9055966404222,153.39261494198));
#86546=CARTESIAN_POINT('Ctrl Pts',(-118.573130216493,18.8975612058818,153.355237560415));
#86547=CARTESIAN_POINT('Ctrl Pts',(-118.567637196493,18.8877211995476,153.318533572216));
#86548=CARTESIAN_POINT('Ctrl Pts',(-118.565894155589,18.8845987762653,153.306886690759));
#86549=CARTESIAN_POINT('Ctrl Pts',(-118.564048110786,18.8812943178558,153.295307498788));
#86550=CARTESIAN_POINT('Ctrl Pts',(-118.562100070791,18.8778102513036,153.283802686776));
#86551=CARTESIAN_POINT('Ctrl Pts',(-118.559067410454,18.8723863429266,153.265892280843));
#86552=CARTESIAN_POINT('Ctrl Pts',(-118.555788379196,18.8665286220844,153.24816250223));
#86553=CARTESIAN_POINT('Ctrl Pts',(-118.552268294674,18.8602489158523,153.230639181705));
#86554=CARTESIAN_POINT('Ctrl Pts',(-118.551651723925,18.8591489754537,153.227569833004));
#86555=CARTESIAN_POINT('Ctrl Pts',(-118.551027749158,18.8580360733877,153.224506614159));
#86556=CARTESIAN_POINT('Ctrl Pts',(-118.550396496785,18.8569104466983,153.221450561457));
#86557=CARTESIAN_POINT('Ctrl Pts',(-118.549451041215,18.8552245440869,153.216873371454));
#86558=CARTESIAN_POINT('Ctrl Pts',(-118.548488694798,18.8535092116976,153.212308955191));
#86559=CARTESIAN_POINT('Ctrl Pts',(-118.547510041777,18.8517655750918,153.207760541832));
#86560=CARTESIAN_POINT('Ctrl Pts',(-118.539440539885,18.8373883866629,153.170256513932));
#86561=CARTESIAN_POINT('Ctrl Pts',(-118.530248612225,18.8210621214486,153.133776898268));
#86562=CARTESIAN_POINT('Ctrl Pts',(-118.519979370497,18.8029154201173,153.098570203321));
#86563=CARTESIAN_POINT('Ctrl Pts',(-118.514671326566,18.7935356148284,153.080372298509));
#86564=CARTESIAN_POINT('Ctrl Pts',(-118.509075277567,18.7836691588754,153.062515275874));
#86565=CARTESIAN_POINT('Ctrl Pts',(-118.50319668039,18.7733327882725,153.045038768438));
#86566=CARTESIAN_POINT('Ctrl Pts',(-118.494570848663,18.7581659396509,153.019394995308));
#86567=CARTESIAN_POINT('Ctrl Pts',(-118.485337290662,18.7419883607805,152.994565543546));
#86568=CARTESIAN_POINT('Ctrl Pts',(-118.475513996705,18.7248554116565,152.970664496244));
#86569=CARTESIAN_POINT('Ctrl Pts',(-118.465690702749,18.7077224625325,152.946763448943));
#86570=CARTESIAN_POINT('Ctrl Pts',(-118.455275811572,18.6896309027286,152.923794471748));
#86571=CARTESIAN_POINT('Ctrl Pts',(-118.444290799697,18.6706436778748,152.901863691503));
#86572=CARTESIAN_POINT('Ctrl Pts',(-118.443473437761,18.6692308951631,152.900231887624));
#86573=CARTESIAN_POINT('Ctrl Pts',(-118.442653055338,18.6678133893012,152.898605923768));
#86574=CARTESIAN_POINT('Ctrl Pts',(-118.441829667636,18.6663911970232,152.896985860847));
#86575=CARTESIAN_POINT('Ctrl Pts',(-118.420960697625,18.6303453732945,152.855924955523));
#86576=CARTESIAN_POINT('Ctrl Pts',(-118.398127427616,18.5912435035496,152.818486237725));
#86577=CARTESIAN_POINT('Ctrl Pts',(-118.373607653542,18.5497069642611,152.785209355589));
#86578=CARTESIAN_POINT('Ctrl Pts',(-118.348072099179,18.5064496914209,152.750553912586));
#86579=CARTESIAN_POINT('Ctrl Pts',(-118.320707604461,18.4605523877565,152.720413135382));
#86580=CARTESIAN_POINT('Ctrl Pts',(-118.2918537178,18.4127621747986,152.695377210154));
#86581=CARTESIAN_POINT('Ctrl Pts',(-118.287748531666,18.4059628232293,152.691815224405));
#86582=CARTESIAN_POINT('Ctrl Pts',(-118.283613234898,18.3991252184581,152.688356527975));
#86583=CARTESIAN_POINT('Ctrl Pts',(-118.279448841604,18.3922515717701,152.685002773781));
#86584=CARTESIAN_POINT('Ctrl Pts',(-118.278651700618,18.3909358301689,152.684360803933));
#86585=CARTESIAN_POINT('Ctrl Pts',(-118.277853564481,18.3896188851033,152.683722731272));
#86586=CARTESIAN_POINT('Ctrl Pts',(-118.277054437491,18.3883007472027,152.683088562518));
#86587=CARTESIAN_POINT('Ctrl Pts',(-118.256302811182,18.3540715127057,152.666620550358));
#86588=CARTESIAN_POINT('Ctrl Pts',(-118.234954792237,18.319160553495,152.652827752379));
#86589=CARTESIAN_POINT('Ctrl Pts',(-118.213106927497,18.283743787874,152.641735383215));
#86590=CARTESIAN_POINT('Ctrl Pts',(-118.191390078416,18.2485394068949,152.630709531951));
#86591=CARTESIAN_POINT('Ctrl Pts',(-118.169178909844,18.212834480398,152.622351680357));
#86592=CARTESIAN_POINT('Ctrl Pts',(-118.146561622526,18.1767968967697,152.616737045581));
#86593=CARTESIAN_POINT('Ctrl Pts',(-118.123944335209,18.1407593131414,152.611122410806));
#86594=CARTESIAN_POINT('Ctrl Pts',(-118.100920482758,18.1043882808045,152.608250762682));
#86595=CARTESIAN_POINT('Ctrl Pts',(-118.077578311569,18.0678585669597,152.608250755187));
#86596=CARTESIAN_POINT('',(-118.588969902809,18.9260953769367,171.108250755187));
#86597=CARTESIAN_POINT('',(-118.588969902809,18.9260953769367,171.608250755187));
#86598=CARTESIAN_POINT('Origin',(-104.59506494869,26.6830679909832,171.108250755187));
#86599=CARTESIAN_POINT('Origin',(-104.59506494869,26.6830679909832,152.108250755187));
#86600=CARTESIAN_POINT('Origin',(-104.59506494869,26.6830679909832,153.108250755187));
#86601=CARTESIAN_POINT('',(-101.803422330775,23.8631510023956,172.108250755187));
#86602=CARTESIAN_POINT('',(-107.386707566605,29.5029849795709,172.108250755187));
#86603=CARTESIAN_POINT('Origin',(-104.59506494869,26.6830679909832,172.108250755187));
#86604=CARTESIAN_POINT('',(-107.386707566605,29.5029849795709,172.608250755187));
#86605=CARTESIAN_POINT('',(-107.386707566605,29.5029849795709,153.108250755187));
#86606=CARTESIAN_POINT('',(-101.803422330775,23.8631510023956,172.608250755187));
#86607=CARTESIAN_POINT('Origin',(-104.59506494869,26.6830679909832,172.608250755187));
#86608=CARTESIAN_POINT('',(-101.803422330775,23.8631510023956,153.108250755187));
#86609=CARTESIAN_POINT('Origin',(-104.59506494869,26.6830679909832,172.108250755187));
#86610=CARTESIAN_POINT('',(-101.451654817389,23.5078207102358,171.608250755187));
#86611=CARTESIAN_POINT('Origin',(-101.451654817389,23.5078207102358,172.108250755187));
#86612=CARTESIAN_POINT('',(-107.738475079991,29.8583152717307,171.608250755187));
#86613=CARTESIAN_POINT('Origin',(-104.59506494869,26.6830679909832,171.608250755187));
#86614=CARTESIAN_POINT('Origin',(-107.738475079991,29.8583152717307,172.108250755187));
#86615=CARTESIAN_POINT('Origin',(-104.59506494869,26.6830679909832,171.108250755187));
#86616=CARTESIAN_POINT('',(-118.286142887994,19.4164054241714,171.608250755187));
#86617=CARTESIAN_POINT('Ctrl Pts',(-118.286142887994,19.4164054241713,171.608250755187));
#86618=CARTESIAN_POINT('Ctrl Pts',(-118.302185325772,19.3896971879647,171.608250755187));
#86619=CARTESIAN_POINT('Ctrl Pts',(-118.318199921039,19.3631642033379,171.606119035114));
#86620=CARTESIAN_POINT('Ctrl Pts',(-118.33408048304,19.3369687870384,171.601866237762));
#86621=CARTESIAN_POINT('Ctrl Pts',(-118.349524991939,19.3114926521192,171.59773021496));
#86622=CARTESIAN_POINT('Ctrl Pts',(-118.36484326585,19.2863349716358,171.59158772586));
#86623=CARTESIAN_POINT('Ctrl Pts',(-118.379930666554,19.2616587919161,171.583402532591));
#86624=CARTESIAN_POINT('Ctrl Pts',(-118.386479406906,19.2509480076639,171.579849720115));
#86625=CARTESIAN_POINT('Ctrl Pts',(-118.39298451303,19.240328189853,171.575911483355));
#86626=CARTESIAN_POINT('Ctrl Pts',(-118.399436615525,19.2298141093875,171.57158222553));
#86627=CARTESIAN_POINT('Ctrl Pts',(-118.413723814319,19.2065322787209,171.561995743106));
#86628=CARTESIAN_POINT('Ctrl Pts',(-118.4276586612,19.1839180856243,171.550546208524));
#86629=CARTESIAN_POINT('Ctrl Pts',(-118.441115563924,19.1621551516899,171.537246666312));
#86630=CARTESIAN_POINT('Ctrl Pts',(-118.453872254784,19.1415246227997,171.52463914792));
#86631=CARTESIAN_POINT('Ctrl Pts',(-118.466199710331,19.1216587053993,171.510368657222));
#86632=CARTESIAN_POINT('Ctrl Pts',(-118.477968777846,19.1027490964865,171.494425144437));
#86633=CARTESIAN_POINT('Ctrl Pts',(-118.482589906378,19.0953242318429,171.488164918489));
#86634=CARTESIAN_POINT('Ctrl Pts',(-118.487124674916,19.0880472321337,171.48164655399));
#86635=CARTESIAN_POINT('Ctrl Pts',(-118.491564119309,19.0809314970593,171.474868716253));
#86636=CARTESIAN_POINT('Ctrl Pts',(-118.493589137647,19.0776857093564,171.471777057816));
#86637=CARTESIAN_POINT('Ctrl Pts',(-118.495593035932,19.0744755040767,171.468633337136));
#86638=CARTESIAN_POINT('Ctrl Pts',(-118.497574879897,19.0713022787009,171.465437794362));
#86639=CARTESIAN_POINT('Ctrl Pts',(-118.509817058045,19.051700740414,171.445698397808));
#86640=CARTESIAN_POINT('Ctrl Pts',(-118.521194139698,19.0335459229592,171.423959301334));
#86641=CARTESIAN_POINT('Ctrl Pts',(-118.531468150003,19.0171904481872,171.400512409472));
#86642=CARTESIAN_POINT('Ctrl Pts',(-118.54099374159,19.002026401407,171.378773525704));
#86643=CARTESIAN_POINT('Ctrl Pts',(-118.549570988509,18.9884092853584,171.355566752543));
#86644=CARTESIAN_POINT('Ctrl Pts',(-118.556992948035,18.9766454465187,171.331150570564));
#86645=CARTESIAN_POINT('Ctrl Pts',(-118.55979681479,18.9722013052469,171.321926628999));
#86646=CARTESIAN_POINT('Ctrl Pts',(-118.562436589657,18.9680203916148,171.312526353858));
#86647=CARTESIAN_POINT('Ctrl Pts',(-118.56489645112,18.964126514061,171.302980969397));
#86648=CARTESIAN_POINT('Ctrl Pts',(-118.566941566645,18.9608891653092,171.295044988349));
#86649=CARTESIAN_POINT('Ctrl Pts',(-118.568864875742,18.9578459265386,171.286995184802));
#86650=CARTESIAN_POINT('Ctrl Pts',(-118.570661329118,18.9550044569664,171.278854434802));
#86651=CARTESIAN_POINT('Ctrl Pts',(-118.575332050019,18.9476167276229,171.257688747076));
#86652=CARTESIAN_POINT('Ctrl Pts',(-118.579148064562,18.9415884594895,171.235909909701));
#86653=CARTESIAN_POINT('Ctrl Pts',(-118.582070947222,18.9369745864019,171.213680494807));
#86654=CARTESIAN_POINT('Ctrl Pts',(-118.584872012388,18.9325530065136,171.192377539143));
#86655=CARTESIAN_POINT('Ctrl Pts',(-118.586852864555,18.9294303689664,171.170659720195));
#86656=CARTESIAN_POINT('Ctrl Pts',(-118.587954670714,18.9276943711425,171.148671871491));
#86657=CARTESIAN_POINT('Ctrl Pts',(-118.588625418196,18.9266375462553,171.13528630994));
#86658=CARTESIAN_POINT('Ctrl Pts',(-118.588969902809,18.9260953769367,171.121800772669));
#86659=CARTESIAN_POINT('Ctrl Pts',(-118.588969902809,18.9260953769367,171.108250755187));
#86660=CARTESIAN_POINT('',(-111.999322625392,13.0659108626764,171.608250755187));
#86661=CARTESIAN_POINT('Origin',(-104.59506494869,26.6830679909832,171.608250755187));
#86662=CARTESIAN_POINT('Ctrl Pts',(-112.492659345135,12.768040044578,171.108250755187));
#86663=CARTESIAN_POINT('Ctrl Pts',(-112.492659345135,12.768040044578,171.13083841899));
#86664=CARTESIAN_POINT('Ctrl Pts',(-112.491148987968,12.7689784818048,171.153252246832));
#86665=CARTESIAN_POINT('Ctrl Pts',(-112.488239747042,12.770782703053,171.17533199473));
#86666=CARTESIAN_POINT('Ctrl Pts',(-112.485198504088,12.7726687878766,171.19841357492));
#86667=CARTESIAN_POINT('Ctrl Pts',(-112.48062856265,12.7755010159135,171.221131109194));
#86668=CARTESIAN_POINT('Ctrl Pts',(-112.474611075407,12.7792252792491,171.243315149928));
#86669=CARTESIAN_POINT('Ctrl Pts',(-112.4731153884,12.7801509699996,171.248829142754));
#86670=CARTESIAN_POINT('Ctrl Pts',(-112.471530056724,12.7811319046715,171.254310195157));
#86671=CARTESIAN_POINT('Ctrl Pts',(-112.469855909556,12.7821675113977,171.259755708108));
#86672=CARTESIAN_POINT('Ctrl Pts',(-112.465313911514,12.7849771351943,171.27452950436));
#86673=CARTESIAN_POINT('Ctrl Pts',(-112.460117552039,12.7881895603694,171.289041238678));
#86674=CARTESIAN_POINT('Ctrl Pts',(-112.45429845138,12.7917840756337,171.303197876379));
#86675=CARTESIAN_POINT('Ctrl Pts',(-112.451837145533,12.7933044482744,171.309185711473));
#86676=CARTESIAN_POINT('Ctrl Pts',(-112.449263349994,12.7948937448599,171.315113565351));
#86677=CARTESIAN_POINT('Ctrl Pts',(-112.446581969183,12.7965487469991,171.320976176106));
#86678=CARTESIAN_POINT('Ctrl Pts',(-112.433991994688,12.8043195323466,171.348503082977));
#86679=CARTESIAN_POINT('Ctrl Pts',(-112.419032456129,12.813537291141,171.374583846366));
#86680=CARTESIAN_POINT('Ctrl Pts',(-112.402171437491,12.8238954967047,171.398817826505));
#86681=CARTESIAN_POINT('Ctrl Pts',(-112.386488190105,12.8335301637326,171.421359021305));
#86682=CARTESIAN_POINT('Ctrl Pts',(-112.369160238947,12.8441512616082,171.442302499413));
#86683=CARTESIAN_POINT('Ctrl Pts',(-112.350556132769,12.8555190964742,171.461373719866));
#86684=CARTESIAN_POINT('Ctrl Pts',(-112.349159012588,12.8563727914249,171.462805919119));
#86685=CARTESIAN_POINT('Ctrl Pts',(-112.347754689754,12.8572307021413,171.464227583082));
#86686=CARTESIAN_POINT('Ctrl Pts',(-112.346343317434,12.858092729399,171.465638607126));
#86687=CARTESIAN_POINT('Ctrl Pts',(-112.343322278299,12.8599378967184,171.468658900776));
#86688=CARTESIAN_POINT('Ctrl Pts',(-112.340265588914,12.8618039160818,171.471633649355));
#86689=CARTESIAN_POINT('Ctrl Pts',(-112.337175174345,12.8636895691223,171.474562315445));
#86690=CARTESIAN_POINT('Ctrl Pts',(-112.320153524577,12.8740755302676,171.490693073098));
#86691=CARTESIAN_POINT('Ctrl Pts',(-112.302126698691,12.8850431839654,171.5054110965));
#86692=CARTESIAN_POINT('Ctrl Pts',(-112.283339116041,12.896436216056,171.518686045026));
#86693=CARTESIAN_POINT('Ctrl Pts',(-112.263152157685,12.9086778475984,171.532949765808));
#86694=CARTESIAN_POINT('Ctrl Pts',(-112.242086394472,12.9214109244347,171.545548160215));
#86695=CARTESIAN_POINT('Ctrl Pts',(-112.220395747739,12.9344717190782,171.556423719585));
#86696=CARTESIAN_POINT('Ctrl Pts',(-112.209365692527,12.941113350736,171.561954122703));
#86697=CARTESIAN_POINT('Ctrl Pts',(-112.198173339535,12.9478401579873,171.567038641577));
#86698=CARTESIAN_POINT('Ctrl Pts',(-112.186848432126,12.9546327985747,171.571666998134));
#86699=CARTESIAN_POINT('Ctrl Pts',(-112.163706014081,12.9685135414746,171.581125032396));
#86700=CARTESIAN_POINT('Ctrl Pts',(-112.139785120082,12.9828022164443,171.58875486132));
#86701=CARTESIAN_POINT('Ctrl Pts',(-112.115420185619,12.9972962282834,171.594560491601));
#86702=CARTESIAN_POINT('Ctrl Pts',(-112.090440971411,13.0121556578048,171.600512491292));
#86703=CARTESIAN_POINT('Ctrl Pts',(-112.064993329893,13.0272319598494,171.604547546384));
#86704=CARTESIAN_POINT('Ctrl Pts',(-112.039420334739,13.0423156811498,171.606621211165));
#86705=CARTESIAN_POINT('Ctrl Pts',(-112.026072225888,13.0501887970118,171.60770358353));
#86706=CARTESIAN_POINT('Ctrl Pts',(-112.01268984259,13.0580639808388,171.608250755187));
#86707=CARTESIAN_POINT('Ctrl Pts',(-111.999322625392,13.0659108626764,171.608250755187));
#86708=CARTESIAN_POINT('Origin',(-104.59506494869,26.6830679909832,172.608250755187));
#86709=CARTESIAN_POINT('',(-107.034940053219,29.147654687411,173.108250755187));
#86710=CARTESIAN_POINT('Origin',(-107.034940053219,29.147654687411,172.608250755187));
#86711=CARTESIAN_POINT('',(-102.15518984416,24.2184812945555,173.108250755187));
#86712=CARTESIAN_POINT('Origin',(-104.59506494869,26.6830679909832,173.108250755187));
#86713=CARTESIAN_POINT('Origin',(-102.15518984416,24.2184812945555,172.608250755187));
#86714=CARTESIAN_POINT('Origin',(-104.59506494869,26.6830679909832,152.108250755187));
#86715=CARTESIAN_POINT('',(-120.09506494869,26.6830679909832,151.608250755187));
#86716=CARTESIAN_POINT('Origin',(-120.09506494869,26.6830679909832,152.108250755187));
#86717=CARTESIAN_POINT('Origin',(-104.59506494869,26.6830679909832,151.608250755187));
#86718=CARTESIAN_POINT('Origin',(-34.5950649486897,26.6830679909832,171.608250755187));
#86719=CARTESIAN_POINT('',(-50.5950649486897,26.6830679909832,152.108250755187));
#86720=CARTESIAN_POINT('',(-18.5950649486897,26.6830679909832,152.108250755187));
#86721=CARTESIAN_POINT('Origin',(-34.5950649486897,26.6830679909832,152.108250755187));
#86722=CARTESIAN_POINT('',(-18.5950649486897,26.6830679909832,171.108250755187));
#86723=CARTESIAN_POINT('',(-18.5950649486897,26.6830679909832,171.608250755187));
#86724=CARTESIAN_POINT('',(-42.4926593451348,12.768040044578,171.108250755187));
#86725=CARTESIAN_POINT('Origin',(-34.5950649486897,26.6830679909832,171.108250755187));
#86726=CARTESIAN_POINT('',(-42.4926593451348,12.768040044578,153.608250755187));
#86727=CARTESIAN_POINT('',(-42.4926593451348,12.768040044578,171.608250755187));
#86728=CARTESIAN_POINT('',(-43.3456993209664,13.2880540647968,152.608250755187));
#86729=CARTESIAN_POINT('Ctrl Pts',(-43.3456993209664,13.2880540647967,152.608250755187));
#86730=CARTESIAN_POINT('Ctrl Pts',(-43.3148053886973,13.2678718158571,152.60825075831));
#86731=CARTESIAN_POINT('Ctrl Pts',(-43.283882083922,13.2478335725253,152.610400982821));
#86732=CARTESIAN_POINT('Ctrl Pts',(-43.2531438546813,13.2280604794972,152.614563215045));
#86733=CARTESIAN_POINT('Ctrl Pts',(-43.2212651740174,13.2075537641154,152.618879874632));
#86734=CARTESIAN_POINT('Ctrl Pts',(-43.1895845524561,13.1873316127627,152.625360599389));
#86735=CARTESIAN_POINT('Ctrl Pts',(-43.1583197319398,13.1675195649551,152.633903745455));
#86736=CARTESIAN_POINT('Ctrl Pts',(-43.126367003911,13.1472716004751,152.642634862993));
#86737=CARTESIAN_POINT('Ctrl Pts',(-43.094847362034,13.1274512359979,152.653520253591));
#86738=CARTESIAN_POINT('Ctrl Pts',(-43.0639884242618,13.1081932944003,152.666504445653));
#86739=CARTESIAN_POINT('Ctrl Pts',(-43.0517916303728,13.1005817185864,152.671636362881));
#86740=CARTESIAN_POINT('Ctrl Pts',(-43.0396980987932,13.0930580740539,152.677096714821));
#86741=CARTESIAN_POINT('Ctrl Pts',(-43.0277223365409,13.0856311228787,152.682884240716));
#86742=CARTESIAN_POINT('Ctrl Pts',(-43.0260492324864,13.0845935219426,152.68369280161));
#86743=CARTESIAN_POINT('Ctrl Pts',(-43.0243776833816,13.0835573316238,152.684508023839));
#86744=CARTESIAN_POINT('Ctrl Pts',(-43.0227077171508,13.0825225645949,152.685329889023));
#86745=CARTESIAN_POINT('Ctrl Pts',(-42.9727957075848,13.0515954111635,152.709893824594));
#86746=CARTESIAN_POINT('Ctrl Pts',(-42.9244661992627,13.0220440815316,152.74032765976));
#86747=CARTESIAN_POINT('Ctrl Pts',(-42.8788647383815,12.9944473172044,152.775796511355));
#86748=CARTESIAN_POINT('Ctrl Pts',(-42.8373562463308,12.9693275063351,152.808081848623));
#86749=CARTESIAN_POINT('Ctrl Pts',(-42.7981083532053,12.9458272165084,152.844537973172));
#86750=CARTESIAN_POINT('Ctrl Pts',(-42.7619450573485,12.9243594465134,152.884524370521));
#86751=CARTESIAN_POINT('Ctrl Pts',(-42.7583791546756,12.922242604655,152.888467252324));
#86752=CARTESIAN_POINT('Ctrl Pts',(-42.7548432071236,12.9201455041938,152.892444455838));
#86753=CARTESIAN_POINT('Ctrl Pts',(-42.7513379798555,12.9180685269602,152.896455365443));
#86754=CARTESIAN_POINT('Ctrl Pts',(-42.7496423779711,12.9170638199208,152.898395583684));
#86755=CARTESIAN_POINT('Ctrl Pts',(-42.7479533619165,12.9160634384558,152.900344344347));
#86756=CARTESIAN_POINT('Ctrl Pts',(-42.7462709958856,12.9150674101677,152.902301551645));
#86757=CARTESIAN_POINT('Ctrl Pts',(-42.707269815392,12.8919771442397,152.947674195698));
#86758=CARTESIAN_POINT('Ctrl Pts',(-42.6718390280897,12.871223865758,152.997605490932));
#86759=CARTESIAN_POINT('Ctrl Pts',(-42.6407188519244,12.8531192060995,153.051009927998));
#86760=CARTESIAN_POINT('Ctrl Pts',(-42.6095986757592,12.835014546441,153.104414365063));
#86761=CARTESIAN_POINT('Ctrl Pts',(-42.582788322685,12.8195581462718,153.161292777412));
#86762=CARTESIAN_POINT('Ctrl Pts',(-42.5610220724519,12.8070625461647,153.22061351513));
#86763=CARTESIAN_POINT('Ctrl Pts',(-42.5603653739899,12.8066855477711,153.222403250928));
#86764=CARTESIAN_POINT('Ctrl Pts',(-42.5597132460627,12.8063112214619,153.22419533454));
#86765=CARTESIAN_POINT('Ctrl Pts',(-42.5590656950375,12.8059395694612,153.225989728665));
#86766=CARTESIAN_POINT('Ctrl Pts',(-42.5465659349297,12.7987655234443,153.260627147538));
#86767=CARTESIAN_POINT('Ctrl Pts',(-42.535812880978,12.7926115974429,153.296006270054));
#86768=CARTESIAN_POINT('Ctrl Pts',(-42.5268031767919,12.7874655986576,153.331953347763));
#86769=CARTESIAN_POINT('Ctrl Pts',(-42.5177414915513,12.7822899102801,153.368107820407));
#86770=CARTESIAN_POINT('Ctrl Pts',(-42.5104430618402,12.7781337002298,153.404837909212));
#86771=CARTESIAN_POINT('Ctrl Pts',(-42.504946453,12.7750090296599,153.441987310225));
#86772=CARTESIAN_POINT('Ctrl Pts',(-42.4995690352926,12.7719521159626,153.478331145603));
#86773=CARTESIAN_POINT('Ctrl Pts',(-42.4959160446013,12.7698824718329,153.515077343029));
#86774=CARTESIAN_POINT('Ctrl Pts',(-42.4940660584642,12.76883553197,153.552083286413));
#86775=CARTESIAN_POINT('Ctrl Pts',(-42.4931330726453,12.7683075387998,153.57074613999));
#86776=CARTESIAN_POINT('Ctrl Pts',(-42.4926593480585,12.7680400462373,153.589475021945));
#86777=CARTESIAN_POINT('Ctrl Pts',(-42.4926593451348,12.768040044578,153.608250755187));
#86778=CARTESIAN_POINT('',(-48.0775783115689,18.0678585669597,152.608250755187));
#86779=CARTESIAN_POINT('Origin',(-34.5950649486897,26.6830679909832,152.608250755187));
#86780=CARTESIAN_POINT('',(-48.5889699028093,18.9260953769367,153.608250755187));
#86781=CARTESIAN_POINT('Ctrl Pts',(-48.5889699028093,18.9260953769367,153.608250755187));
#86782=CARTESIAN_POINT('Ctrl Pts',(-48.5889699023077,18.9260953760317,153.570920583159));
#86783=CARTESIAN_POINT('Ctrl Pts',(-48.5879121048548,18.9241774989272,153.533707722378));
#86784=CARTESIAN_POINT('Ctrl Pts',(-48.5858434641496,18.9204434093262,153.496805212593));
#86785=CARTESIAN_POINT('Ctrl Pts',(-48.5845964757606,18.9181924788654,153.474560169695));
#86786=CARTESIAN_POINT('Ctrl Pts',(-48.5829816609043,18.9152806425278,153.452427631477));
#86787=CARTESIAN_POINT('Ctrl Pts',(-48.5810049418185,18.911722257265,153.430449466818));
#86788=CARTESIAN_POINT('Ctrl Pts',(-48.577602099566,18.9055966404233,153.392614941987));
#86789=CARTESIAN_POINT('Ctrl Pts',(-48.5731302164946,18.8975612058847,153.355237560429));
#86790=CARTESIAN_POINT('Ctrl Pts',(-48.5676371964959,18.8877211995531,153.318533572236));
#86791=CARTESIAN_POINT('Ctrl Pts',(-48.5658941555907,18.8845987762691,153.306886690772));
#86792=CARTESIAN_POINT('Ctrl Pts',(-48.5640481107871,18.8812943178578,153.295307498794));
#86793=CARTESIAN_POINT('Ctrl Pts',(-48.5621000707914,18.8778102513037,153.283802686776));
#86794=CARTESIAN_POINT('Ctrl Pts',(-48.5590674104541,18.8723863429266,153.265892280843));
#86795=CARTESIAN_POINT('Ctrl Pts',(-48.5557883791962,18.8665286220844,153.24816250223));
#86796=CARTESIAN_POINT('Ctrl Pts',(-48.5522682946736,18.8602489158523,153.230639181705));
#86797=CARTESIAN_POINT('Ctrl Pts',(-48.5516517239249,18.8591489754537,153.227569833004));
#86798=CARTESIAN_POINT('Ctrl Pts',(-48.5510277491576,18.8580360733877,153.224506614159));
#86799=CARTESIAN_POINT('Ctrl Pts',(-48.5503964967849,18.8569104466983,153.221450561457));
#86800=CARTESIAN_POINT('Ctrl Pts',(-48.5494510412146,18.855224544087,153.216873371454));
#86801=CARTESIAN_POINT('Ctrl Pts',(-48.5484886947976,18.8535092116976,153.212308955191));
#86802=CARTESIAN_POINT('Ctrl Pts',(-48.5475100417767,18.8517655750918,153.207760541832));
#86803=CARTESIAN_POINT('Ctrl Pts',(-48.5394405398847,18.8373883866618,153.170256513929));
#86804=CARTESIAN_POINT('Ctrl Pts',(-48.530248612224,18.8210621214462,153.133776898263));
#86805=CARTESIAN_POINT('Ctrl Pts',(-48.5199793704951,18.8029154201132,153.098570203313));
#86806=CARTESIAN_POINT('Ctrl Pts',(-48.5146713265647,18.7935356148255,153.080372298504));
#86807=CARTESIAN_POINT('Ctrl Pts',(-48.5090752775665,18.783669158874,153.062515275872));
#86808=CARTESIAN_POINT('Ctrl Pts',(-48.5031966803903,18.7733327882725,153.045038768438));
#86809=CARTESIAN_POINT('Ctrl Pts',(-48.494570848663,18.758165939651,153.019394995308));
#86810=CARTESIAN_POINT('Ctrl Pts',(-48.4853372906616,18.7419883607805,152.994565543546));
#86811=CARTESIAN_POINT('Ctrl Pts',(-48.4755139967052,18.7248554116565,152.970664496244));
#86812=CARTESIAN_POINT('Ctrl Pts',(-48.4656907027488,18.7077224625325,152.946763448943));
#86813=CARTESIAN_POINT('Ctrl Pts',(-48.455275811572,18.6896309027286,152.923794471748));
#86814=CARTESIAN_POINT('Ctrl Pts',(-48.4442907996973,18.6706436778748,152.901863691503));
#86815=CARTESIAN_POINT('Ctrl Pts',(-48.4434734377613,18.6692308951631,152.900231887624));
#86816=CARTESIAN_POINT('Ctrl Pts',(-48.4426530553384,18.6678133893012,152.898605923768));
#86817=CARTESIAN_POINT('Ctrl Pts',(-48.4418296676355,18.6663911970232,152.896985860847));
#86818=CARTESIAN_POINT('Ctrl Pts',(-48.4209606976304,18.6303453733033,152.855924955533));
#86819=CARTESIAN_POINT('Ctrl Pts',(-48.3981274276271,18.5912435035687,152.818486237743));
#86820=CARTESIAN_POINT('Ctrl Pts',(-48.3736076535603,18.5497069642916,152.785209355613));
#86821=CARTESIAN_POINT('Ctrl Pts',(-48.3480720992044,18.5064496914645,152.750553912618));
#86822=CARTESIAN_POINT('Ctrl Pts',(-48.3207076044961,18.4605523878146,152.720413135418));
#86823=CARTESIAN_POINT('Ctrl Pts',(-48.291853717844,18.4127621748717,152.695377210192));
#86824=CARTESIAN_POINT('Ctrl Pts',(-48.2877485316961,18.4059628232783,152.691815224429));
#86825=CARTESIAN_POINT('Ctrl Pts',(-48.283613234913,18.3991252184827,152.688356527986));
#86826=CARTESIAN_POINT('Ctrl Pts',(-48.279448841604,18.3922515717701,152.68500277378));
#86827=CARTESIAN_POINT('Ctrl Pts',(-48.2786517006176,18.3909358301689,152.684360803933));
#86828=CARTESIAN_POINT('Ctrl Pts',(-48.2778535644812,18.3896188851034,152.683722731272));
#86829=CARTESIAN_POINT('Ctrl Pts',(-48.277054437491,18.3883007472027,152.683088562518));
#86830=CARTESIAN_POINT('Ctrl Pts',(-48.2563028111771,18.3540715126977,152.666620550354));
#86831=CARTESIAN_POINT('Ctrl Pts',(-48.2349547922275,18.3191605534787,152.652827752373));
#86832=CARTESIAN_POINT('Ctrl Pts',(-48.2131069274817,18.2837437878493,152.641735383207));
#86833=CARTESIAN_POINT('Ctrl Pts',(-48.1913900784035,18.248539406874,152.630709531945));
#86834=CARTESIAN_POINT('Ctrl Pts',(-48.1691789098335,18.2128344803812,152.622351680354));
#86835=CARTESIAN_POINT('Ctrl Pts',(-48.1465616225185,18.1767968967571,152.616737045579));
#86836=CARTESIAN_POINT('Ctrl Pts',(-48.1239443352035,18.1407593131329,152.611122410805));
#86837=CARTESIAN_POINT('Ctrl Pts',(-48.1009204827551,18.1043882808003,152.608250762682));
#86838=CARTESIAN_POINT('Ctrl Pts',(-48.0775783115689,18.0678585669597,152.608250755187));
#86839=CARTESIAN_POINT('',(-48.5889699028093,18.9260953769367,171.108250755187));
#86840=CARTESIAN_POINT('',(-48.5889699028093,18.9260953769367,171.608250755187));
#86841=CARTESIAN_POINT('Origin',(-34.5950649486897,26.6830679909832,171.108250755187));
#86842=CARTESIAN_POINT('Origin',(-34.5950649486897,26.6830679909832,152.108250755187));
#86843=CARTESIAN_POINT('Origin',(-34.5950649486897,26.6830679909832,153.108250755187));
#86844=CARTESIAN_POINT('',(-31.8034223307746,23.8631510023956,172.108250755187));
#86845=CARTESIAN_POINT('',(-37.3867075666049,29.5029849795709,172.108250755187));
#86846=CARTESIAN_POINT('Origin',(-34.5950649486897,26.6830679909832,172.108250755187));
#86847=CARTESIAN_POINT('',(-37.3867075666049,29.5029849795709,172.608250755187));
#86848=CARTESIAN_POINT('',(-37.3867075666049,29.5029849795709,153.108250755187));
#86849=CARTESIAN_POINT('',(-31.8034223307746,23.8631510023956,172.608250755187));
#86850=CARTESIAN_POINT('Origin',(-34.5950649486897,26.6830679909832,172.608250755187));
#86851=CARTESIAN_POINT('',(-31.8034223307746,23.8631510023956,153.108250755187));
#86852=CARTESIAN_POINT('Origin',(-34.5950649486897,26.6830679909832,172.108250755187));
#86853=CARTESIAN_POINT('',(-31.4516548173888,23.5078207102358,171.608250755187));
#86854=CARTESIAN_POINT('Origin',(-31.4516548173888,23.5078207102358,172.108250755187));
#86855=CARTESIAN_POINT('',(-37.7384750799907,29.8583152717307,171.608250755187));
#86856=CARTESIAN_POINT('Origin',(-34.5950649486897,26.6830679909832,171.608250755187));
#86857=CARTESIAN_POINT('Origin',(-37.7384750799907,29.8583152717307,172.108250755187));
#86858=CARTESIAN_POINT('Origin',(-34.5950649486897,26.6830679909832,171.108250755187));
#86859=CARTESIAN_POINT('',(-48.2861428879937,19.4164054241714,171.608250755187));
#86860=CARTESIAN_POINT('Ctrl Pts',(-48.2861428879937,19.4164054241714,171.608250755187));
#86861=CARTESIAN_POINT('Ctrl Pts',(-48.3021853257697,19.3896971879684,171.608250755187));
#86862=CARTESIAN_POINT('Ctrl Pts',(-48.3181999210346,19.3631642033453,171.606119035115));
#86863=CARTESIAN_POINT('Ctrl Pts',(-48.3340804830342,19.3369687870493,171.601866237764));
#86864=CARTESIAN_POINT('Ctrl Pts',(-48.3495249919314,19.3114926521329,171.597730214963));
#86865=CARTESIAN_POINT('Ctrl Pts',(-48.3648432658407,19.2863349716523,171.591587725864));
#86866=CARTESIAN_POINT('Ctrl Pts',(-48.3799306665435,19.2616587919351,171.583402532597));
#86867=CARTESIAN_POINT('Ctrl Pts',(-48.3864794068996,19.2509480076768,171.57984972012));
#86868=CARTESIAN_POINT('Ctrl Pts',(-48.392984513027,19.2403281898597,171.575911483358));
#86869=CARTESIAN_POINT('Ctrl Pts',(-48.399436615526,19.2298141093882,171.57158222553));
#86870=CARTESIAN_POINT('Ctrl Pts',(-48.4137238143177,19.2065322787241,171.561995743107));
#86871=CARTESIAN_POINT('Ctrl Pts',(-48.4276586611977,19.1839180856298,171.550546208526));
#86872=CARTESIAN_POINT('Ctrl Pts',(-48.4411155639197,19.1621551516974,171.537246666316));
#86873=CARTESIAN_POINT('Ctrl Pts',(-48.4538722547784,19.1415246228092,171.524639147927));
#86874=CARTESIAN_POINT('Ctrl Pts',(-48.4661997103245,19.1216587054105,171.51036865723));
#86875=CARTESIAN_POINT('Ctrl Pts',(-48.4779687778381,19.1027490964993,171.494425144447));
#86876=CARTESIAN_POINT('Ctrl Pts',(-48.4825899063729,19.0953242318513,171.488164918496));
#86877=CARTESIAN_POINT('Ctrl Pts',(-48.4871246749138,19.0880472321378,171.481646553994));
#86878=CARTESIAN_POINT('Ctrl Pts',(-48.4915641193089,19.0809314970594,171.474868716253));
#86879=CARTESIAN_POINT('Ctrl Pts',(-48.4935891376473,19.0776857093565,171.471777057816));
#86880=CARTESIAN_POINT('Ctrl Pts',(-48.4955930359323,19.0744755040767,171.468633337136));
#86881=CARTESIAN_POINT('Ctrl Pts',(-48.4975748798971,19.071302278701,171.465437794362));
#86882=CARTESIAN_POINT('Ctrl Pts',(-48.5098170580377,19.0517007404259,171.44569839782));
#86883=CARTESIAN_POINT('Ctrl Pts',(-48.5211941396845,19.0335459229812,171.42395930136));
#86884=CARTESIAN_POINT('Ctrl Pts',(-48.531468149985,19.0171904482168,171.400512409514));
#86885=CARTESIAN_POINT('Ctrl Pts',(-48.5409937415793,19.0020264014248,171.378773525734));
#86886=CARTESIAN_POINT('Ctrl Pts',(-48.5495709885045,18.9884092853662,171.355566752559));
#86887=CARTESIAN_POINT('Ctrl Pts',(-48.5569929480345,18.9766454465188,171.331150570564));
#86888=CARTESIAN_POINT('Ctrl Pts',(-48.5597968147904,18.972201305247,171.321926628999));
#86889=CARTESIAN_POINT('Ctrl Pts',(-48.5624365896571,18.9680203916148,171.312526353858));
#86890=CARTESIAN_POINT('Ctrl Pts',(-48.5648964511201,18.964126514061,171.302980969397));
#86891=CARTESIAN_POINT('Ctrl Pts',(-48.5669415666449,18.9608891653093,171.295044988349));
#86892=CARTESIAN_POINT('Ctrl Pts',(-48.5688648757415,18.9578459265386,171.286995184802));
#86893=CARTESIAN_POINT('Ctrl Pts',(-48.5706613291176,18.9550044569664,171.278854434802));
#86894=CARTESIAN_POINT('Ctrl Pts',(-48.5753320500147,18.947616727629,171.257688747093));
#86895=CARTESIAN_POINT('Ctrl Pts',(-48.5791480645553,18.9415884594994,171.235909909737));
#86896=CARTESIAN_POINT('Ctrl Pts',(-48.5820709472144,18.9369745864134,171.213680494862));
#86897=CARTESIAN_POINT('Ctrl Pts',(-48.5848720123792,18.9325530065268,171.192377539217));
#86898=CARTESIAN_POINT('Ctrl Pts',(-48.5868528645474,18.9294303689789,171.17065972029));
#86899=CARTESIAN_POINT('Ctrl Pts',(-48.5879546707082,18.9276943711517,171.148671871607));
#86900=CARTESIAN_POINT('Ctrl Pts',(-48.5886254181942,18.9266375462585,171.135286310018));
#86901=CARTESIAN_POINT('Ctrl Pts',(-48.5889699028093,18.9260953769367,171.121800772708));
#86902=CARTESIAN_POINT('Ctrl Pts',(-48.5889699028093,18.9260953769367,171.108250755187));
#86903=CARTESIAN_POINT('',(-41.9993226253918,13.0659108626764,171.608250755187));
#86904=CARTESIAN_POINT('Origin',(-34.5950649486897,26.6830679909832,171.608250755187));
#86905=CARTESIAN_POINT('Ctrl Pts',(-42.4926593451348,12.768040044578,171.108250755187));
#86906=CARTESIAN_POINT('Ctrl Pts',(-42.4926593451348,12.768040044578,171.130838418967));
#86907=CARTESIAN_POINT('Ctrl Pts',(-42.4911489879713,12.7689784818031,171.153252246788));
#86908=CARTESIAN_POINT('Ctrl Pts',(-42.488239747051,12.7707827030479,171.175331994665));
#86909=CARTESIAN_POINT('Ctrl Pts',(-42.4851985041028,12.7726687878681,171.198413574834));
#86910=CARTESIAN_POINT('Ctrl Pts',(-42.4806285626732,12.7755010158997,171.221131109087));
#86911=CARTESIAN_POINT('Ctrl Pts',(-42.4746110754411,12.7792252792283,171.243315149802));
#86912=CARTESIAN_POINT('Ctrl Pts',(-42.4731153884239,12.7801509699851,171.248829142671));
#86913=CARTESIAN_POINT('Ctrl Pts',(-42.4715300567366,12.781131904664,171.254310195115));
#86914=CARTESIAN_POINT('Ctrl Pts',(-42.4698559095559,12.782167511398,171.259755708107));
#86915=CARTESIAN_POINT('Ctrl Pts',(-42.4653139115146,12.7849771351945,171.27452950436));
#86916=CARTESIAN_POINT('Ctrl Pts',(-42.4601175520392,12.7881895603695,171.289041238678));
#86917=CARTESIAN_POINT('Ctrl Pts',(-42.4542984513799,12.7917840756337,171.303197876379));
#86918=CARTESIAN_POINT('Ctrl Pts',(-42.4518371455332,12.7933044482744,171.309185711473));
#86919=CARTESIAN_POINT('Ctrl Pts',(-42.4492633499944,12.7948937448598,171.315113565351));
#86920=CARTESIAN_POINT('Ctrl Pts',(-42.4465819691828,12.796548746999,171.320976176106));
#86921=CARTESIAN_POINT('Ctrl Pts',(-42.4339919946876,12.8043195323464,171.348503082977));
#86922=CARTESIAN_POINT('Ctrl Pts',(-42.4190324561286,12.8135372911409,171.374583846366));
#86923=CARTESIAN_POINT('Ctrl Pts',(-42.4021714374908,12.8238954967045,171.398817826505));
#86924=CARTESIAN_POINT('Ctrl Pts',(-42.3864881901019,12.8335301637344,171.42135902131));
#86925=CARTESIAN_POINT('Ctrl Pts',(-42.3691602389399,12.8441512616124,171.442302499421));
#86926=CARTESIAN_POINT('Ctrl Pts',(-42.3505561327577,12.855519096481,171.461373719878));
#86927=CARTESIAN_POINT('Ctrl Pts',(-42.3491590125803,12.8563727914294,171.462805919127));
#86928=CARTESIAN_POINT('Ctrl Pts',(-42.3477546897505,12.8572307021435,171.464227583086));
#86929=CARTESIAN_POINT('Ctrl Pts',(-42.3463433174337,12.858092729399,171.465638607126));
#86930=CARTESIAN_POINT('Ctrl Pts',(-42.3433222782986,12.8599378967184,171.468658900776));
#86931=CARTESIAN_POINT('Ctrl Pts',(-42.3402655889138,12.8618039160818,171.471633649355));
#86932=CARTESIAN_POINT('Ctrl Pts',(-42.3371751743445,12.8636895691222,171.474562315445));
#86933=CARTESIAN_POINT('Ctrl Pts',(-42.3201535245773,12.8740755302671,171.490693073097));
#86934=CARTESIAN_POINT('Ctrl Pts',(-42.3021266986922,12.8850431839643,171.505411096499));
#86935=CARTESIAN_POINT('Ctrl Pts',(-42.2833391160437,12.8964362160542,171.518686045024));
#86936=CARTESIAN_POINT('Ctrl Pts',(-42.2631521576885,12.9086778475957,171.532949765805));
#86937=CARTESIAN_POINT('Ctrl Pts',(-42.2420863944765,12.9214109244311,171.545548160212));
#86938=CARTESIAN_POINT('Ctrl Pts',(-42.2203957477446,12.9344717190736,171.556423719582));
#86939=CARTESIAN_POINT('Ctrl Pts',(-42.2093656925312,12.9411133507326,171.561954122701));
#86940=CARTESIAN_POINT('Ctrl Pts',(-42.1981733395362,12.9478401579852,171.567038641576));
#86941=CARTESIAN_POINT('Ctrl Pts',(-42.1868484321251,12.9546327985739,171.571666998134));
#86942=CARTESIAN_POINT('Ctrl Pts',(-42.1637060140812,12.9685135414727,171.581125032395));
#86943=CARTESIAN_POINT('Ctrl Pts',(-42.1397851200849,12.9828022164415,171.588754861319));
#86944=CARTESIAN_POINT('Ctrl Pts',(-42.115420185623,12.9972962282797,171.594560491599));
#86945=CARTESIAN_POINT('Ctrl Pts',(-42.0904409714184,13.0121556577995,171.60051249129));
#86946=CARTESIAN_POINT('Ctrl Pts',(-42.0649933299033,13.0272319598426,171.604547546382));
#86947=CARTESIAN_POINT('Ctrl Pts',(-42.0394203347526,13.0423156811413,171.606621211164));
#86948=CARTESIAN_POINT('Ctrl Pts',(-42.0260722258977,13.0501887970062,171.607703583529));
#86949=CARTESIAN_POINT('Ctrl Pts',(-42.0126898425947,13.0580639808361,171.608250755187));
#86950=CARTESIAN_POINT('Ctrl Pts',(-41.9993226253918,13.0659108626764,171.608250755187));
#86951=CARTESIAN_POINT('Origin',(-34.5950649486897,26.6830679909832,172.608250755187));
#86952=CARTESIAN_POINT('',(-37.0349400532192,29.147654687411,173.108250755187));
#86953=CARTESIAN_POINT('Origin',(-37.0349400532192,29.147654687411,172.608250755187));
#86954=CARTESIAN_POINT('',(-32.1551898441603,24.2184812945555,173.108250755187));
#86955=CARTESIAN_POINT('Origin',(-34.5950649486897,26.6830679909832,173.108250755187));
#86956=CARTESIAN_POINT('Origin',(-32.1551898441603,24.2184812945555,172.608250755187));
#86957=CARTESIAN_POINT('Origin',(-34.5950649486897,26.6830679909832,152.108250755187));
#86958=CARTESIAN_POINT('',(-50.0950649486897,26.6830679909832,151.608250755187));
#86959=CARTESIAN_POINT('Origin',(-50.0950649486897,26.6830679909832,152.108250755187));
#86960=CARTESIAN_POINT('Origin',(-34.5950649486897,26.6830679909832,151.608250755187));
#86961=CARTESIAN_POINT('Origin',(35.4049350513103,26.6830679909832,171.608250755187));
#86962=CARTESIAN_POINT('',(19.4049350513103,26.6830679909833,152.108250755187));
#86963=CARTESIAN_POINT('',(51.4049350513103,26.6830679909832,152.108250755187));
#86964=CARTESIAN_POINT('Origin',(35.4049350513103,26.6830679909832,152.108250755187));
#86965=CARTESIAN_POINT('',(51.4049350513103,26.6830679909832,171.108250755187));
#86966=CARTESIAN_POINT('',(51.4049350513103,26.6830679909832,171.608250755187));
#86967=CARTESIAN_POINT('',(27.5073406548652,12.768040044578,171.108250755187));
#86968=CARTESIAN_POINT('Origin',(35.4049350513103,26.6830679909832,171.108250755187));
#86969=CARTESIAN_POINT('',(27.5073406548652,12.768040044578,153.608250755187));
#86970=CARTESIAN_POINT('',(27.5073406548652,12.768040044578,171.608250755187));
#86971=CARTESIAN_POINT('',(26.6543006790336,13.2880540647968,152.608250755187));
#86972=CARTESIAN_POINT('Ctrl Pts',(26.6543006790336,13.2880540647968,152.608250755187));
#86973=CARTESIAN_POINT('Ctrl Pts',(26.6851946113006,13.2678718158584,152.60825075831));
#86974=CARTESIAN_POINT('Ctrl Pts',(26.7161179160738,13.247833572528,152.610400982821));
#86975=CARTESIAN_POINT('Ctrl Pts',(26.7468561453125,13.2280604795012,152.614563215044));
#86976=CARTESIAN_POINT('Ctrl Pts',(26.7787348259742,13.2075537641208,152.61887987463));
#86977=CARTESIAN_POINT('Ctrl Pts',(26.8104154475333,13.1873316127695,152.625360599387));
#86978=CARTESIAN_POINT('Ctrl Pts',(26.8416802680476,13.1675195649632,152.633903745451));
#86979=CARTESIAN_POINT('Ctrl Pts',(26.873632996074,13.1472716004846,152.642634862988));
#86980=CARTESIAN_POINT('Ctrl Pts',(26.9051526379488,13.1274512360087,152.653520253585));
#86981=CARTESIAN_POINT('Ctrl Pts',(26.9360115757189,13.1081932944124,152.666504445645));
#86982=CARTESIAN_POINT('Ctrl Pts',(26.9482083696144,13.1005817185943,152.671636362875));
#86983=CARTESIAN_POINT('Ctrl Pts',(26.9603019012005,13.0930580740578,152.677096714818));
#86984=CARTESIAN_POINT('Ctrl Pts',(26.9722776634591,13.0856311228788,152.682884240716));
#86985=CARTESIAN_POINT('Ctrl Pts',(26.9739507675136,13.0845935219426,152.68369280161));
#86986=CARTESIAN_POINT('Ctrl Pts',(26.9756223166184,13.0835573316238,152.684508023839));
#86987=CARTESIAN_POINT('Ctrl Pts',(26.9772922828492,13.082522564595,152.685329889023));
#86988=CARTESIAN_POINT('Ctrl Pts',(27.0272042924152,13.0515954111636,152.709893824594));
#86989=CARTESIAN_POINT('Ctrl Pts',(27.0755338007373,13.0220440815316,152.74032765976));
#86990=CARTESIAN_POINT('Ctrl Pts',(27.1211352616185,12.9944473172044,152.775796511355));
#86991=CARTESIAN_POINT('Ctrl Pts',(27.1626437536728,12.969327506333,152.808081848625));
#86992=CARTESIAN_POINT('Ctrl Pts',(27.2018916468014,12.9458272165044,152.844537973178));
#86993=CARTESIAN_POINT('Ctrl Pts',(27.2380549426608,12.9243594465078,152.884524370531));
#86994=CARTESIAN_POINT('Ctrl Pts',(27.2416208453306,12.9222426046513,152.888467252331));
#86995=CARTESIAN_POINT('Ctrl Pts',(27.2451567928795,12.9201455041919,152.892444455841));
#86996=CARTESIAN_POINT('Ctrl Pts',(27.2486620201446,12.9180685269602,152.896455365443));
#86997=CARTESIAN_POINT('Ctrl Pts',(27.250357622029,12.9170638199208,152.898395583684));
#86998=CARTESIAN_POINT('Ctrl Pts',(27.2520466380835,12.9160634384558,152.900344344347));
#86999=CARTESIAN_POINT('Ctrl Pts',(27.2537290041144,12.9150674101677,152.902301551645));
#87000=CARTESIAN_POINT('Ctrl Pts',(27.2927301846081,12.8919771442397,152.947674195698));
#87001=CARTESIAN_POINT('Ctrl Pts',(27.3281609719104,12.8712238657579,152.997605490932));
#87002=CARTESIAN_POINT('Ctrl Pts',(27.3592811480756,12.8531192060994,153.051009927998));
#87003=CARTESIAN_POINT('Ctrl Pts',(27.3904013242408,12.835014546441,153.104414365063));
#87004=CARTESIAN_POINT('Ctrl Pts',(27.417211677315,12.8195581462718,153.161292777412));
#87005=CARTESIAN_POINT('Ctrl Pts',(27.4389779275479,12.8070625461649,153.22061351513));
#87006=CARTESIAN_POINT('Ctrl Pts',(27.4396346260099,12.8066855477713,153.222403250928));
#87007=CARTESIAN_POINT('Ctrl Pts',(27.4402867539371,12.8063112214621,153.22419533454));
#87008=CARTESIAN_POINT('Ctrl Pts',(27.4409343049623,12.8059395694613,153.225989728665));
#87009=CARTESIAN_POINT('Ctrl Pts',(27.4534340650697,12.7987655234446,153.260627147537));
#87010=CARTESIAN_POINT('Ctrl Pts',(27.4641871190213,12.7926115974433,153.296006270053));
#87011=CARTESIAN_POINT('Ctrl Pts',(27.4731968232073,12.7874655986581,153.331953347762));
#87012=CARTESIAN_POINT('Ctrl Pts',(27.4822585084477,12.7822899102806,153.368107820404));
#87013=CARTESIAN_POINT('Ctrl Pts',(27.4895569381589,12.7781337002303,153.404837909208));
#87014=CARTESIAN_POINT('Ctrl Pts',(27.4950535469991,12.7750090296604,153.441987310221));
#87015=CARTESIAN_POINT('Ctrl Pts',(27.5004309647065,12.7719521159632,153.478331145598));
#87016=CARTESIAN_POINT('Ctrl Pts',(27.5040839553981,12.7698824718333,153.515077343023));
#87017=CARTESIAN_POINT('Ctrl Pts',(27.5059339415353,12.7688355319703,153.552083286406));
#87018=CARTESIAN_POINT('Ctrl Pts',(27.5068669273545,12.7683075387999,153.570746139986));
#87019=CARTESIAN_POINT('Ctrl Pts',(27.5073406519415,12.7680400462374,153.589475021942));
#87020=CARTESIAN_POINT('Ctrl Pts',(27.5073406548652,12.768040044578,153.608250755187));
#87021=CARTESIAN_POINT('',(21.9224216884311,18.0678585669597,152.608250755187));
#87022=CARTESIAN_POINT('Origin',(35.4049350513103,26.6830679909832,152.608250755187));
#87023=CARTESIAN_POINT('',(21.4110300971907,18.9260953769367,153.608250755187));
#87024=CARTESIAN_POINT('Ctrl Pts',(21.4110300971907,18.9260953769367,153.608250755187));
#87025=CARTESIAN_POINT('Ctrl Pts',(21.4110300976924,18.9260953760316,153.570920583161));
#87026=CARTESIAN_POINT('Ctrl Pts',(21.4120878951452,18.9241774989273,153.533707722381));
#87027=CARTESIAN_POINT('Ctrl Pts',(21.4141565358502,18.9204434093267,153.496805212598));
#87028=CARTESIAN_POINT('Ctrl Pts',(21.4154035242392,18.9181924788658,153.474560169699));
#87029=CARTESIAN_POINT('Ctrl Pts',(21.4170183390955,18.9152806425281,153.452427631479));
#87030=CARTESIAN_POINT('Ctrl Pts',(21.4189950581815,18.911722257265,153.430449466818));
#87031=CARTESIAN_POINT('Ctrl Pts',(21.4223979004345,18.9055966404225,153.392614941982));
#87032=CARTESIAN_POINT('Ctrl Pts',(21.4268697835066,18.8975612058826,153.355237560419));
#87033=CARTESIAN_POINT('Ctrl Pts',(21.4323628035064,18.8877211995491,153.318533572221));
#87034=CARTESIAN_POINT('Ctrl Pts',(21.4341058444109,18.8845987762663,153.306886690763));
#87035=CARTESIAN_POINT('Ctrl Pts',(21.4359518892137,18.8812943178563,153.295307498789));
#87036=CARTESIAN_POINT('Ctrl Pts',(21.4378999292086,18.8778102513037,153.283802686776));
#87037=CARTESIAN_POINT('Ctrl Pts',(21.4409325895459,18.8723863429266,153.265892280843));
#87038=CARTESIAN_POINT('Ctrl Pts',(21.4442116208038,18.8665286220844,153.248162502229));
#87039=CARTESIAN_POINT('Ctrl Pts',(21.4477317053264,18.8602489158523,153.230639181705));
#87040=CARTESIAN_POINT('Ctrl Pts',(21.4483482760751,18.8591489754537,153.227569833004));
#87041=CARTESIAN_POINT('Ctrl Pts',(21.4489722508424,18.8580360733877,153.224506614159));
#87042=CARTESIAN_POINT('Ctrl Pts',(21.4496035032151,18.8569104466983,153.221450561457));
#87043=CARTESIAN_POINT('Ctrl Pts',(21.4505489587854,18.855224544087,153.216873371454));
#87044=CARTESIAN_POINT('Ctrl Pts',(21.4515113052024,18.8535092116976,153.212308955191));
#87045=CARTESIAN_POINT('Ctrl Pts',(21.4524899582233,18.8517655750918,153.207760541832));
#87046=CARTESIAN_POINT('Ctrl Pts',(21.4605594601156,18.8373883866613,153.170256513927));
#87047=CARTESIAN_POINT('Ctrl Pts',(21.4697513877767,18.8210621214449,153.13377689826));
#87048=CARTESIAN_POINT('Ctrl Pts',(21.480020629506,18.8029154201111,153.098570203309));
#87049=CARTESIAN_POINT('Ctrl Pts',(21.4853286734362,18.7935356148241,153.080372298501));
#87050=CARTESIAN_POINT('Ctrl Pts',(21.490924722434,18.7836691588732,153.062515275871));
#87051=CARTESIAN_POINT('Ctrl Pts',(21.4968033196097,18.7733327882725,153.045038768438));
#87052=CARTESIAN_POINT('Ctrl Pts',(21.505429151337,18.758165939651,153.019394995308));
#87053=CARTESIAN_POINT('Ctrl Pts',(21.5146627093384,18.7419883607805,152.994565543546));
#87054=CARTESIAN_POINT('Ctrl Pts',(21.5244860032948,18.7248554116565,152.970664496244));
#87055=CARTESIAN_POINT('Ctrl Pts',(21.5343092972512,18.7077224625325,152.946763448943));
#87056=CARTESIAN_POINT('Ctrl Pts',(21.544724188428,18.6896309027287,152.923794471748));
#87057=CARTESIAN_POINT('Ctrl Pts',(21.5557092003027,18.6706436778749,152.901863691503));
#87058=CARTESIAN_POINT('Ctrl Pts',(21.5565265622387,18.6692308951631,152.900231887624));
#87059=CARTESIAN_POINT('Ctrl Pts',(21.5573469446616,18.6678133893012,152.898605923768));
#87060=CARTESIAN_POINT('Ctrl Pts',(21.5581703323645,18.6663911970232,152.896985860847));
#87061=CARTESIAN_POINT('Ctrl Pts',(21.5790393023703,18.630345373302,152.855924955531));
#87062=CARTESIAN_POINT('Ctrl Pts',(21.6018725723745,18.5912435035659,152.818486237741));
#87063=CARTESIAN_POINT('Ctrl Pts',(21.6263923464424,18.5497069642871,152.785209355609));
#87064=CARTESIAN_POINT('Ctrl Pts',(21.6519279007995,18.5064496914579,152.750553912613));
#87065=CARTESIAN_POINT('Ctrl Pts',(21.6792923955092,18.4605523878058,152.720413135413));
#87066=CARTESIAN_POINT('Ctrl Pts',(21.7081462821627,18.4127621748605,152.695377210186));
#87067=CARTESIAN_POINT('Ctrl Pts',(21.7122514683085,18.4059628232708,152.691815224426));
#87068=CARTESIAN_POINT('Ctrl Pts',(21.7163867650893,18.399125218479,152.688356527985));
#87069=CARTESIAN_POINT('Ctrl Pts',(21.720551158396,18.3922515717701,152.68500277378));
#87070=CARTESIAN_POINT('Ctrl Pts',(21.7213482993824,18.3909358301689,152.684360803933));
#87071=CARTESIAN_POINT('Ctrl Pts',(21.7221464355189,18.3896188851033,152.683722731272));
#87072=CARTESIAN_POINT('Ctrl Pts',(21.722945562509,18.3883007472027,152.683088562518));
#87073=CARTESIAN_POINT('Ctrl Pts',(21.7436971888205,18.3540715127016,152.666620550356));
#87074=CARTESIAN_POINT('Ctrl Pts',(21.7650452077676,18.3191605534867,152.652827752376));
#87075=CARTESIAN_POINT('Ctrl Pts',(21.7868930725109,18.2837437878615,152.641735383211));
#87076=CARTESIAN_POINT('Ctrl Pts',(21.8086099215902,18.2485394068843,152.630709531948));
#87077=CARTESIAN_POINT('Ctrl Pts',(21.8308210901613,18.2128344803894,152.622351680356));
#87078=CARTESIAN_POINT('Ctrl Pts',(21.8534383774776,18.1767968967633,152.61673704558));
#87079=CARTESIAN_POINT('Ctrl Pts',(21.8760556647939,18.1407593131371,152.611122410805));
#87080=CARTESIAN_POINT('Ctrl Pts',(21.8990795172436,18.1043882808024,152.608250762682));
#87081=CARTESIAN_POINT('Ctrl Pts',(21.9224216884311,18.0678585669597,152.608250755187));
#87082=CARTESIAN_POINT('',(21.4110300971907,18.9260953769367,171.108250755187));
#87083=CARTESIAN_POINT('',(21.4110300971907,18.9260953769367,171.608250755187));
#87084=CARTESIAN_POINT('Origin',(35.4049350513103,26.6830679909832,171.108250755187));
#87085=CARTESIAN_POINT('Origin',(35.4049350513103,26.6830679909832,152.108250755187));
#87086=CARTESIAN_POINT('Origin',(35.4049350513103,26.6830679909832,153.108250755187));
#87087=CARTESIAN_POINT('',(38.1965776692254,23.8631510023956,172.108250755187));
#87088=CARTESIAN_POINT('',(32.6132924333951,29.5029849795709,172.108250755187));
#87089=CARTESIAN_POINT('Origin',(35.4049350513103,26.6830679909832,172.108250755187));
#87090=CARTESIAN_POINT('',(32.6132924333951,29.5029849795709,172.608250755187));
#87091=CARTESIAN_POINT('',(32.6132924333951,29.5029849795709,153.108250755187));
#87092=CARTESIAN_POINT('',(38.1965776692254,23.8631510023956,172.608250755187));
#87093=CARTESIAN_POINT('Origin',(35.4049350513103,26.6830679909832,172.608250755187));
#87094=CARTESIAN_POINT('',(38.1965776692254,23.8631510023956,153.108250755187));
#87095=CARTESIAN_POINT('Origin',(35.4049350513103,26.6830679909832,172.108250755187));
#87096=CARTESIAN_POINT('',(38.5483451826112,23.5078207102358,171.608250755187));
#87097=CARTESIAN_POINT('Origin',(38.5483451826112,23.5078207102358,172.108250755187));
#87098=CARTESIAN_POINT('',(32.2615249200093,29.8583152717307,171.608250755187));
#87099=CARTESIAN_POINT('Origin',(35.4049350513103,26.6830679909832,171.608250755187));
#87100=CARTESIAN_POINT('Origin',(32.2615249200093,29.8583152717307,172.108250755187));
#87101=CARTESIAN_POINT('Origin',(35.4049350513103,26.6830679909832,171.108250755187));
#87102=CARTESIAN_POINT('',(21.7138571120063,19.4164054241714,171.608250755187));
#87103=CARTESIAN_POINT('Ctrl Pts',(21.7138571120063,19.4164054241714,171.608250755187));
#87104=CARTESIAN_POINT('Ctrl Pts',(21.6978146742301,19.3896971879681,171.608250755187));
#87105=CARTESIAN_POINT('Ctrl Pts',(21.6818000789652,19.3631642033449,171.606119035115));
#87106=CARTESIAN_POINT('Ctrl Pts',(21.6659195169656,19.3369687870488,171.601866237764));
#87107=CARTESIAN_POINT('Ctrl Pts',(21.6504750080682,19.311492652132,171.597730214963));
#87108=CARTESIAN_POINT('Ctrl Pts',(21.6351567341587,19.2863349716511,171.591587725864));
#87109=CARTESIAN_POINT('Ctrl Pts',(21.6200693334557,19.2616587919335,171.583402532597));
#87110=CARTESIAN_POINT('Ctrl Pts',(21.6135205931,19.2509480076757,171.579849720119));
#87111=CARTESIAN_POINT('Ctrl Pts',(21.6070154869729,19.2403281898591,171.575911483357));
#87112=CARTESIAN_POINT('Ctrl Pts',(21.6005633844741,19.2298141093881,171.57158222553));
#87113=CARTESIAN_POINT('Ctrl Pts',(21.5862761856819,19.2065322787234,171.561995743107));
#87114=CARTESIAN_POINT('Ctrl Pts',(21.5723413388016,19.1839180856286,171.550546208526));
#87115=CARTESIAN_POINT('Ctrl Pts',(21.5588844360793,19.1621551516958,171.537246666315));
#87116=CARTESIAN_POINT('Ctrl Pts',(21.5461277452202,19.1415246228069,171.524639147925));
#87117=CARTESIAN_POINT('Ctrl Pts',(21.5338002896738,19.1216587054077,171.510368657228));
#87118=CARTESIAN_POINT('Ctrl Pts',(21.5220312221599,19.102749096496,171.494425144445));
#87119=CARTESIAN_POINT('Ctrl Pts',(21.5174100936258,19.0953242318491,171.488164918495));
#87120=CARTESIAN_POINT('Ctrl Pts',(21.5128753250856,19.0880472321367,171.481646553993));
#87121=CARTESIAN_POINT('Ctrl Pts',(21.5084358806911,19.0809314970593,171.474868716253));
#87122=CARTESIAN_POINT('Ctrl Pts',(21.5064108623527,19.0776857093565,171.471777057816));
#87123=CARTESIAN_POINT('Ctrl Pts',(21.5044069640677,19.0744755040767,171.468633337136));
#87124=CARTESIAN_POINT('Ctrl Pts',(21.502425120103,19.0713022787009,171.465437794362));
#87125=CARTESIAN_POINT('Ctrl Pts',(21.4901829419552,19.0517007404143,171.445698397808));
#87126=CARTESIAN_POINT('Ctrl Pts',(21.4788058603021,19.0335459229596,171.423959301334));
#87127=CARTESIAN_POINT('Ctrl Pts',(21.4685318499969,19.0171904481876,171.400512409473));
#87128=CARTESIAN_POINT('Ctrl Pts',(21.4590062584099,19.0020264014073,171.378773525704));
#87129=CARTESIAN_POINT('Ctrl Pts',(21.4504290114908,18.9884092853585,171.355566752544));
#87130=CARTESIAN_POINT('Ctrl Pts',(21.4430070519656,18.9766454465187,171.331150570564));
#87131=CARTESIAN_POINT('Ctrl Pts',(21.4402031852097,18.9722013052469,171.321926628999));
#87132=CARTESIAN_POINT('Ctrl Pts',(21.437563410343,18.9680203916148,171.312526353858));
#87133=CARTESIAN_POINT('Ctrl Pts',(21.4351035488799,18.964126514061,171.302980969397));
#87134=CARTESIAN_POINT('Ctrl Pts',(21.433058433355,18.9608891653093,171.295044988349));
#87135=CARTESIAN_POINT('Ctrl Pts',(21.4311351242584,18.9578459265386,171.286995184802));
#87136=CARTESIAN_POINT('Ctrl Pts',(21.4293386708823,18.9550044569664,171.278854434802));
#87137=CARTESIAN_POINT('Ctrl Pts',(21.4246679499804,18.9476167276214,171.257688747072));
#87138=CARTESIAN_POINT('Ctrl Pts',(21.4208519354368,18.941588459487,171.235909909692));
#87139=CARTESIAN_POINT('Ctrl Pts',(21.4179290527765,18.9369745863991,171.213680494794));
#87140=CARTESIAN_POINT('Ctrl Pts',(21.4151279876107,18.932553006511,171.192377539128));
#87141=CARTESIAN_POINT('Ctrl Pts',(21.4131471354433,18.9294303689643,171.170659720179));
#87142=CARTESIAN_POINT('Ctrl Pts',(21.412045329285,18.9276943711411,171.148671871474));
#87143=CARTESIAN_POINT('Ctrl Pts',(21.4113745818035,18.9266375462549,171.135286309929));
#87144=CARTESIAN_POINT('Ctrl Pts',(21.4110300971907,18.9260953769367,171.121800772663));
#87145=CARTESIAN_POINT('Ctrl Pts',(21.4110300971907,18.9260953769367,171.108250755187));
#87146=CARTESIAN_POINT('',(28.0006773746082,13.0659108626764,171.608250755187));
#87147=CARTESIAN_POINT('Origin',(35.4049350513103,26.6830679909832,171.608250755187));
#87148=CARTESIAN_POINT('Ctrl Pts',(27.5073406548652,12.768040044578,171.108250755187));
#87149=CARTESIAN_POINT('Ctrl Pts',(27.5073406548652,12.768040044578,171.13083841897));
#87150=CARTESIAN_POINT('Ctrl Pts',(27.508851012029,12.7689784818034,171.153252246793));
#87151=CARTESIAN_POINT('Ctrl Pts',(27.5117602529499,12.7707827030486,171.175331994673));
#87152=CARTESIAN_POINT('Ctrl Pts',(27.5148014958989,12.7726687878693,171.198413574845));
#87153=CARTESIAN_POINT('Ctrl Pts',(27.5193714373296,12.7755010159017,171.221131109101));
#87154=CARTESIAN_POINT('Ctrl Pts',(27.5253889245633,12.7792252792313,171.243315149819));
#87155=CARTESIAN_POINT('Ctrl Pts',(27.5268846115792,12.7801509699872,171.248829142682));
#87156=CARTESIAN_POINT('Ctrl Pts',(27.5284699432649,12.7811319046652,171.254310195121));
#87157=CARTESIAN_POINT('Ctrl Pts',(27.5301440904439,12.7821675113981,171.259755708108));
#87158=CARTESIAN_POINT('Ctrl Pts',(27.5346860884853,12.7849771351945,171.27452950436));
#87159=CARTESIAN_POINT('Ctrl Pts',(27.5398824479607,12.7881895603696,171.289041238678));
#87160=CARTESIAN_POINT('Ctrl Pts',(27.5457015486201,12.7917840756337,171.303197876379));
#87161=CARTESIAN_POINT('Ctrl Pts',(27.5481628544669,12.7933044482744,171.309185711473));
#87162=CARTESIAN_POINT('Ctrl Pts',(27.5507366500057,12.7948937448598,171.315113565351));
#87163=CARTESIAN_POINT('Ctrl Pts',(27.5534180308173,12.796548746999,171.320976176106));
#87164=CARTESIAN_POINT('Ctrl Pts',(27.5660080053126,12.8043195323464,171.348503082977));
#87165=CARTESIAN_POINT('Ctrl Pts',(27.5809675438715,12.8135372911409,171.374583846366));
#87166=CARTESIAN_POINT('Ctrl Pts',(27.5978285625092,12.8238954967046,171.398817826505));
#87167=CARTESIAN_POINT('Ctrl Pts',(27.6135118098975,12.8335301637343,171.421359021309));
#87168=CARTESIAN_POINT('Ctrl Pts',(27.6308397610588,12.8441512616119,171.44230249942));
#87169=CARTESIAN_POINT('Ctrl Pts',(27.6494438672404,12.8555190964801,171.461373719876));
#87170=CARTESIAN_POINT('Ctrl Pts',(27.6508409874183,12.8563727914288,171.462805919126));
#87171=CARTESIAN_POINT('Ctrl Pts',(27.6522453102488,12.8572307021433,171.464227583086));
#87172=CARTESIAN_POINT('Ctrl Pts',(27.6536566825661,12.8580927293991,171.465638607126));
#87173=CARTESIAN_POINT('Ctrl Pts',(27.6566777217013,12.8599378967185,171.468658900776));
#87174=CARTESIAN_POINT('Ctrl Pts',(27.6597344110861,12.8618039160819,171.471633649355));
#87175=CARTESIAN_POINT('Ctrl Pts',(27.6628248256553,12.8636895691224,171.474562315445));
#87176=CARTESIAN_POINT('Ctrl Pts',(27.6798464754228,12.8740755302673,171.490693073097));
#87177=CARTESIAN_POINT('Ctrl Pts',(27.697873301308,12.8850431839646,171.505411096499));
#87178=CARTESIAN_POINT('Ctrl Pts',(27.7166608839567,12.8964362160547,171.518686045025));
#87179=CARTESIAN_POINT('Ctrl Pts',(27.736847842312,12.9086778475964,171.532949765806));
#87180=CARTESIAN_POINT('Ctrl Pts',(27.7579136055242,12.921410924432,171.545548160212));
#87181=CARTESIAN_POINT('Ctrl Pts',(27.7796042522562,12.9344717190747,171.556423719583));
#87182=CARTESIAN_POINT('Ctrl Pts',(27.7906343074692,12.9411133507335,171.561954122701));
#87183=CARTESIAN_POINT('Ctrl Pts',(27.8018266604637,12.9478401579859,171.567038641576));
#87184=CARTESIAN_POINT('Ctrl Pts',(27.8131515678744,12.9546327985744,171.571666998134));
#87185=CARTESIAN_POINT('Ctrl Pts',(27.8362939859182,12.9685135414732,171.581125032396));
#87186=CARTESIAN_POINT('Ctrl Pts',(27.8602148799146,12.982802216442,171.588754861319));
#87187=CARTESIAN_POINT('Ctrl Pts',(27.8845798143767,12.9972962282802,171.5945604916));
#87188=CARTESIAN_POINT('Ctrl Pts',(27.9095590285816,13.0121556578,171.60051249129));
#87189=CARTESIAN_POINT('Ctrl Pts',(27.9350066700969,13.027231959843,171.604547546382));
#87190=CARTESIAN_POINT('Ctrl Pts',(27.9605796652478,13.0423156811417,171.606621211164));
#87191=CARTESIAN_POINT('Ctrl Pts',(27.9739277741026,13.0501887970065,171.607703583529));
#87192=CARTESIAN_POINT('Ctrl Pts',(27.9873101574055,13.0580639808362,171.608250755187));
#87193=CARTESIAN_POINT('Ctrl Pts',(28.0006773746082,13.0659108626764,171.608250755187));
#87194=CARTESIAN_POINT('Origin',(35.4049350513103,26.6830679909832,172.608250755187));
#87195=CARTESIAN_POINT('',(32.9650599467808,29.147654687411,173.108250755187));
#87196=CARTESIAN_POINT('Origin',(32.9650599467808,29.147654687411,172.608250755187));
#87197=CARTESIAN_POINT('',(37.8448101558397,24.2184812945555,173.108250755187));
#87198=CARTESIAN_POINT('Origin',(35.4049350513103,26.6830679909832,173.108250755187));
#87199=CARTESIAN_POINT('Origin',(37.8448101558397,24.2184812945555,172.608250755187));
#87200=CARTESIAN_POINT('Origin',(35.4049350513103,26.6830679909832,152.108250755187));
#87201=CARTESIAN_POINT('',(19.9049350513103,26.6830679909832,151.608250755187));
#87202=CARTESIAN_POINT('Origin',(19.9049350513103,26.6830679909832,152.108250755187));
#87203=CARTESIAN_POINT('Origin',(35.4049350513103,26.6830679909832,151.608250755187));
#87204=CARTESIAN_POINT('Origin',(125.29348064571,25.4505574462982,227.));
#87205=CARTESIAN_POINT('',(151.316083724746,25.4505574462982,200.));
#87206=CARTESIAN_POINT('Origin',(125.29348064571,25.4505574462982,200.));
#87207=CARTESIAN_POINT('',(151.316083724746,25.4505574462982,226.3));
#87208=CARTESIAN_POINT('',(151.316083724746,25.4505574462982,227.));
#87209=CARTESIAN_POINT('',(119.980756553526,50.9250708612662,226.3));
#87210=CARTESIAN_POINT('Origin',(125.29348064571,25.4505574462982,226.3));
#87211=CARTESIAN_POINT('',(119.980756553526,50.9250708612662,202.7));
#87212=CARTESIAN_POINT('',(119.980756553526,50.9250708612662,227.));
#87213=CARTESIAN_POINT('',(121.344083479533,51.1717186376762,201.3));
#87214=CARTESIAN_POINT('Ctrl Pts',(121.344083479533,51.1717186376762,201.3));
#87215=CARTESIAN_POINT('Ctrl Pts',(121.296814940039,51.164460713567,201.300000001764));
#87216=CARTESIAN_POINT('Ctrl Pts',(121.249631520094,51.1570730071936,201.30261647433));
#87217=CARTESIAN_POINT('Ctrl Pts',(121.202809575166,51.1496136039449,201.307693045627));
#87218=CARTESIAN_POINT('Ctrl Pts',(121.154373252809,51.1418970073598,201.312944652415));
#87219=CARTESIAN_POINT('Ctrl Pts',(121.106322691563,51.1341034996569,201.320828920817));
#87220=CARTESIAN_POINT('Ctrl Pts',(121.058940661441,51.1262905985135,201.331225416489));
#87221=CARTESIAN_POINT('Ctrl Pts',(121.010426286528,51.1182909831689,201.341870369596));
#87222=CARTESIAN_POINT('Ctrl Pts',(120.96261148805,51.1102708092942,201.355149130815));
#87223=CARTESIAN_POINT('Ctrl Pts',(120.915794212708,51.1022880243849,201.370986079636));
#87224=CARTESIAN_POINT('Ctrl Pts',(120.885078842197,51.0970507653943,201.381376213347));
#87225=CARTESIAN_POINT('Ctrl Pts',(120.854792756682,51.0918295287459,201.392868556026));
#87226=CARTESIAN_POINT('Ctrl Pts',(120.825022979086,51.0866405538404,201.405453604755));
#87227=CARTESIAN_POINT('Ctrl Pts',(120.822614540357,51.0862207546636,201.406471762135));
#87228=CARTESIAN_POINT('Ctrl Pts',(120.820208501303,51.0858010088545,201.407497395078));
#87229=CARTESIAN_POINT('Ctrl Pts',(120.817804891954,51.0853813251034,201.408530483275));
#87230=CARTESIAN_POINT('Ctrl Pts',(120.748752458259,51.0733243806588,201.438209704743));
#87231=CARTESIAN_POINT('Ctrl Pts',(120.681875427084,51.0613482917229,201.473987104567));
#87232=CARTESIAN_POINT('Ctrl Pts',(120.618293835989,51.0497349272812,201.51508560388));
#87233=CARTESIAN_POINT('Ctrl Pts',(120.558229638025,51.0387640250305,201.553910495744));
#87234=CARTESIAN_POINT('Ctrl Pts',(120.501106992418,51.0281170259462,201.597483053204));
#87235=CARTESIAN_POINT('Ctrl Pts',(120.447829239022,51.0180241909268,201.645128573345));
#87236=CARTESIAN_POINT('Ctrl Pts',(120.42575040754,51.0138416196026,201.664873351287));
#87237=CARTESIAN_POINT('Ctrl Pts',(120.404331325271,51.0097541109278,201.685317440809));
#87238=CARTESIAN_POINT('Ctrl Pts',(120.383633686815,51.0057775363715,201.706412319778));
#87239=CARTESIAN_POINT('Ctrl Pts',(120.381288649471,51.0053269914529,201.708802364374));
#87240=CARTESIAN_POINT('Ctrl Pts',(120.378951141237,51.0048775527908,201.711202451161));
#87241=CARTESIAN_POINT('Ctrl Pts',(120.376621298644,51.0044292543624,201.713612409408));
#87242=CARTESIAN_POINT('Ctrl Pts',(120.329918672461,50.9954429331492,201.761920985893));
#87243=CARTESIAN_POINT('Ctrl Pts',(120.286217524176,50.986899636637,201.814296128758));
#87244=CARTESIAN_POINT('Ctrl Pts',(120.246644234098,50.9790767475013,201.869390093657));
#87245=CARTESIAN_POINT('Ctrl Pts',(120.235032869601,50.9767814008927,201.885555444244));
#87246=CARTESIAN_POINT('Ctrl Pts',(120.223776558923,50.974548012121,201.901954831386));
#87247=CARTESIAN_POINT('Ctrl Pts',(120.212902870258,50.9723834091261,201.91855423109));
#87248=CARTESIAN_POINT('Ctrl Pts',(120.211224597556,50.9720493188068,201.921116224565));
#87249=CARTESIAN_POINT('Ctrl Pts',(120.209555106758,50.9717168083916,201.923682941432));
#87250=CARTESIAN_POINT('Ctrl Pts',(120.207894399138,50.9713858827489,201.926254375486));
#87251=CARTESIAN_POINT('Ctrl Pts',(120.166433470862,50.9631240525672,201.990452336396));
#87252=CARTESIAN_POINT('Ctrl Pts',(120.130429392281,50.9558466678358,202.057605589415));
#87253=CARTESIAN_POINT('Ctrl Pts',(120.099834407458,50.9496146107615,202.127787837188));
#87254=CARTESIAN_POINT('Ctrl Pts',(120.095136748583,50.9486577193494,202.138563860156));
#87255=CARTESIAN_POINT('Ctrl Pts',(120.090566696606,50.9477254852738,202.149411345588));
#87256=CARTESIAN_POINT('Ctrl Pts',(120.086124170858,50.9468181437796,202.1603306173));
#87257=CARTESIAN_POINT('Ctrl Pts',(120.085241450897,50.9466378570477,202.162500252244));
#87258=CARTESIAN_POINT('Ctrl Pts',(120.084364128845,50.9464586358352,202.164672249676));
#87259=CARTESIAN_POINT('Ctrl Pts',(120.083492209333,50.9462804820366,202.166846579406));
#87260=CARTESIAN_POINT('Ctrl Pts',(120.065306140488,50.9425646376238,202.212197680753));
#87261=CARTESIAN_POINT('Ctrl Pts',(120.049527707131,50.9393249175896,202.258413140069));
#87262=CARTESIAN_POINT('Ctrl Pts',(120.036138534255,50.936566193575,202.305307920115));
#87263=CARTESIAN_POINT('Ctrl Pts',(120.02267110342,50.9337913451802,202.352476794));
#87264=CARTESIAN_POINT('Ctrl Pts',(120.011620718125,50.9315030569102,202.400333921084));
#87265=CARTESIAN_POINT('Ctrl Pts',(120.00301661756,50.9297157845129,202.448711398113));
#87266=CARTESIAN_POINT('Ctrl Pts',(119.994561270883,50.9279594117685,202.496252490468));
#87267=CARTESIAN_POINT('Ctrl Pts',(119.988468284927,50.9266868395961,202.544297037827));
#87268=CARTESIAN_POINT('Ctrl Pts',(119.984813469459,50.9259217362925,202.592691092945));
#87269=CARTESIAN_POINT('Ctrl Pts',(119.982124767438,50.9253588802969,202.628292669809));
#87270=CARTESIAN_POINT('Ctrl Pts',(119.980756556636,50.925070861915,202.664083573468));
#87271=CARTESIAN_POINT('Ctrl Pts',(119.980756553526,50.9250708612662,202.7));
#87272=CARTESIAN_POINT('',(129.242877811887,51.1717186376762,201.3));
#87273=CARTESIAN_POINT('Origin',(125.29348064571,25.4505574462982,201.3));
#87274=CARTESIAN_POINT('',(130.606204737894,50.9250708612662,202.7));
#87275=CARTESIAN_POINT('Ctrl Pts',(130.606204737894,50.9250708612662,202.7));
#87276=CARTESIAN_POINT('Ctrl Pts',(130.606204736907,50.9250708614721,202.649823152623));
#87277=CARTESIAN_POINT('Ctrl Pts',(130.603493048605,50.9256415257708,202.599732878103));
#87278=CARTESIAN_POINT('Ctrl Pts',(130.598216123741,50.9267435592911,202.550016081281));
#87279=CARTESIAN_POINT('Ctrl Pts',(130.592800185238,50.9278746244338,202.49898956089));
#87280=CARTESIAN_POINT('Ctrl Pts',(130.584681986303,50.9295654689291,202.44835525433));
#87281=CARTESIAN_POINT('Ctrl Pts',(130.573966511743,50.9317850515479,202.398409849753));
#87282=CARTESIAN_POINT('Ctrl Pts',(130.563222416445,50.934010562611,202.348331042373));
#87283=CARTESIAN_POINT('Ctrl Pts',(130.549866888012,50.9367677238324,202.298943529959));
#87284=CARTESIAN_POINT('Ctrl Pts',(130.533955804295,50.9400355548964,202.250551985476));
#87285=CARTESIAN_POINT('Ctrl Pts',(130.52453817908,50.9419697542745,202.221909472014));
#87286=CARTESIAN_POINT('Ctrl Pts',(130.514224327984,50.9440830480728,202.193616080543));
#87287=CARTESIAN_POINT('Ctrl Pts',(130.503018172532,50.9463726044773,202.165738725987));
#87288=CARTESIAN_POINT('Ctrl Pts',(130.502391057095,50.946500731931,202.164178662017));
#87289=CARTESIAN_POINT('Ctrl Pts',(130.501761172559,50.9466294061949,202.162619958756));
#87290=CARTESIAN_POINT('Ctrl Pts',(130.501128521321,50.9467586264223,202.161062631988));
#87291=CARTESIAN_POINT('Ctrl Pts',(130.467437757633,50.9536400294536,202.07812984855));
#87292=CARTESIAN_POINT('Ctrl Pts',(130.425599590938,50.9621200262788,201.998148794283));
#87293=CARTESIAN_POINT('Ctrl Pts',(130.376670295168,50.9718651713917,201.92287275644));
#87294=CARTESIAN_POINT('Ctrl Pts',(130.327740999398,50.9816103165046,201.847596718597));
#87295=CARTESIAN_POINT('Ctrl Pts',(130.271720626042,50.9926205787292,201.777026086224));
#87296=CARTESIAN_POINT('Ctrl Pts',(130.20970669802,51.0045511176674,201.712958049445));
#87297=CARTESIAN_POINT('Ctrl Pts',(130.207830086632,51.0049121492283,201.71101927841));
#87298=CARTESIAN_POINT('Ctrl Pts',(130.205947872494,51.0052740452498,201.709086313541));
#87299=CARTESIAN_POINT('Ctrl Pts',(130.204060089613,51.0056367953596,201.707159214017));
#87300=CARTESIAN_POINT('Ctrl Pts',(130.163509016277,51.0134289553865,201.665763588018));
#87301=CARTESIAN_POINT('Ctrl Pts',(130.119885380912,51.0217082832857,201.626558866243));
#87302=CARTESIAN_POINT('Ctrl Pts',(130.074141666999,51.0302581165978,201.590396521904));
#87303=CARTESIAN_POINT('Ctrl Pts',(130.050982804967,51.0345866765929,201.572088460059));
#87304=CARTESIAN_POINT('Ctrl Pts',(130.027281461632,51.0389844001929,201.554560066656));
#87305=CARTESIAN_POINT('Ctrl Pts',(130.00316572107,51.043422400071,201.5379199304));
#87306=CARTESIAN_POINT('Ctrl Pts',(130.001082367498,51.0438057979135,201.536482392654));
#87307=CARTESIAN_POINT('Ctrl Pts',(129.998995800011,51.0441895186937,201.535051370118));
#87308=CARTESIAN_POINT('Ctrl Pts',(129.996906096631,51.0445735445554,201.533626931406));
#87309=CARTESIAN_POINT('Ctrl Pts',(129.930621956132,51.0567546150476,201.488444588001));
#87310=CARTESIAN_POINT('Ctrl Pts',(129.86081854997,51.0693171758067,201.449358588045));
#87311=CARTESIAN_POINT('Ctrl Pts',(129.787469755343,51.0821772615741,201.416548723103));
#87312=CARTESIAN_POINT('Ctrl Pts',(129.78103100378,51.0833061539812,201.413668586214));
#87313=CARTESIAN_POINT('Ctrl Pts',(129.774564952339,51.0844373354015,201.410836785548));
#87314=CARTESIAN_POINT('Ctrl Pts',(129.768071595154,51.0855707469888,201.408053427281));
#87315=CARTESIAN_POINT('Ctrl Pts',(129.766264252068,51.0858862176364,201.407278715036));
#87316=CARTESIAN_POINT('Ctrl Pts',(129.764454981671,51.0862018282248,201.4065078337));
#87317=CARTESIAN_POINT('Ctrl Pts',(129.762643778742,51.0865175784956,201.405740780295));
#87318=CARTESIAN_POINT('Ctrl Pts',(129.714272775736,51.0949501826254,201.385255421096));
#87319=CARTESIAN_POINT('Ctrl Pts',(129.664883221933,51.1034125934789,201.367706325503));
#87320=CARTESIAN_POINT('Ctrl Pts',(129.614679793085,51.1118624165726,201.35310702986));
#87321=CARTESIAN_POINT('Ctrl Pts',(129.564594471029,51.1202923609145,201.338542079997));
#87322=CARTESIAN_POINT('Ctrl Pts',(129.51369823572,51.1287099459605,201.326912907498));
#87323=CARTESIAN_POINT('Ctrl Pts',(129.46218278672,51.1370724391893,201.318283262024));
#87324=CARTESIAN_POINT('Ctrl Pts',(129.41177367354,51.1452553411305,201.309838945148));
#87325=CARTESIAN_POINT('Ctrl Pts',(129.360770860779,51.1533856413995,201.304266683087));
#87326=CARTESIAN_POINT('Ctrl Pts',(129.309355143587,51.1614203559357,201.301675514577));
#87327=CARTESIAN_POINT('Ctrl Pts',(129.287267165588,51.1648720358419,201.300562359376));
#87328=CARTESIAN_POINT('Ctrl Pts',(129.265103069234,51.1683060247023,201.300000002005));
#87329=CARTESIAN_POINT('Ctrl Pts',(129.242877811887,51.1717186376762,201.3));
#87330=CARTESIAN_POINT('',(130.606204737894,50.9250708612662,226.3));
#87331=CARTESIAN_POINT('',(130.606204737894,50.9250708612662,227.));
#87332=CARTESIAN_POINT('Origin',(125.29348064571,25.4505574462982,226.3));
#87333=CARTESIAN_POINT('Origin',(125.29348064571,25.4505574462982,226.3));
#87334=CARTESIAN_POINT('',(130.749115378049,50.178482477843,227.));
#87335=CARTESIAN_POINT('Ctrl Pts',(130.606204737894,50.9250708612662,226.3));
#87336=CARTESIAN_POINT('Ctrl Pts',(130.606204737894,50.9250708612662,226.327283375706));
#87337=CARTESIAN_POINT('Ctrl Pts',(130.606521196537,50.9233280888925,226.354433744169));
#87338=CARTESIAN_POINT('Ctrl Pts',(130.607134490211,50.9199608865016,226.381298026589));
#87339=CARTESIAN_POINT('Ctrl Pts',(130.607772970913,50.9164553982781,226.409265583844));
#87340=CARTESIAN_POINT('Ctrl Pts',(130.608733160752,50.9111893063652,226.436924230535));
#87341=CARTESIAN_POINT('Ctrl Pts',(130.610002771111,50.9042414687086,226.464113586868));
#87342=CARTESIAN_POINT('Ctrl Pts',(130.610977695644,50.8989062748601,226.484992095236));
#87343=CARTESIAN_POINT('Ctrl Pts',(130.612135280192,50.8925782669583,226.505594295321));
#87344=CARTESIAN_POINT('Ctrl Pts',(130.613473681732,50.8852727968182,226.525845500815));
#87345=CARTESIAN_POINT('Ctrl Pts',(130.614470475815,50.8798319413003,226.540927881695));
#87346=CARTESIAN_POINT('Ctrl Pts',(130.615567141013,50.8738512343175,226.555805651625));
#87347=CARTESIAN_POINT('Ctrl Pts',(130.616760678055,50.8673492154425,226.570416316965));
#87348=CARTESIAN_POINT('Ctrl Pts',(130.618997538772,50.8551634934195,226.597798813054));
#87349=CARTESIAN_POINT('Ctrl Pts',(130.621587650642,50.8410803822523,226.624424058888));
#87350=CARTESIAN_POINT('Ctrl Pts',(130.624488519249,50.8253628624445,226.649987233896));
#87351=CARTESIAN_POINT('Ctrl Pts',(130.625554698216,50.8195860792457,226.659382667889));
#87352=CARTESIAN_POINT('Ctrl Pts',(130.62666277844,50.8135889080171,226.668634944449));
#87353=CARTESIAN_POINT('Ctrl Pts',(130.62781040101,50.8073856540369,226.677730163301));
#87354=CARTESIAN_POINT('Ctrl Pts',(130.631954405204,50.7849860331286,226.710572515881));
#87355=CARTESIAN_POINT('Ctrl Pts',(130.636632724928,50.7597985255623,226.741511971335));
#87356=CARTESIAN_POINT('Ctrl Pts',(130.641763810671,50.7323297966851,226.770042486735));
#87357=CARTESIAN_POINT('Ctrl Pts',(130.643470156645,50.7231950526413,226.779530328593));
#87358=CARTESIAN_POINT('Ctrl Pts',(130.645226560496,50.7138080496165,226.788752180359));
#87359=CARTESIAN_POINT('Ctrl Pts',(130.647029992641,50.7041874189799,226.797690746489));
#87360=CARTESIAN_POINT('Ctrl Pts',(130.647571851327,50.7012968071615,226.800376425409));
#87361=CARTESIAN_POINT('Ctrl Pts',(130.648118782333,50.6983807626333,226.803040587555));
#87362=CARTESIAN_POINT('Ctrl Pts',(130.64867056125,50.6954405413581,226.805682465323));
#87363=CARTESIAN_POINT('Ctrl Pts',(130.653661469249,50.6688458792137,226.829578573851));
#87364=CARTESIAN_POINT('Ctrl Pts',(130.659056798759,50.6402484831699,226.851675168384));
#87365=CARTESIAN_POINT('Ctrl Pts',(130.664705914535,50.6104938033034,226.871445497822));
#87366=CARTESIAN_POINT('Ctrl Pts',(130.665956597121,50.6039062838658,226.875822538006));
#87367=CARTESIAN_POINT('Ctrl Pts',(130.667219752626,50.5972618524138,226.880085629563));
#87368=CARTESIAN_POINT('Ctrl Pts',(130.668493801137,50.5905693773403,226.884229173985));
#87369=CARTESIAN_POINT('Ctrl Pts',(130.676235766143,50.5499014534891,226.909408102141));
#87370=CARTESIAN_POINT('Ctrl Pts',(130.684436648208,50.5071526195933,226.930546414023));
#87371=CARTESIAN_POINT('Ctrl Pts',(130.693116168835,50.4623179858518,226.947750095497));
#87372=CARTESIAN_POINT('Ctrl Pts',(130.693628527943,50.4596713612343,226.9487656427));
#87373=CARTESIAN_POINT('Ctrl Pts',(130.694142145785,50.4570196470152,226.949766385399));
#87374=CARTESIAN_POINT('Ctrl Pts',(130.694656993051,50.4543629986236,226.950752326852));
#87375=CARTESIAN_POINT('Ctrl Pts',(130.700229539504,50.4256082638754,226.961423850053));
#87376=CARTESIAN_POINT('Ctrl Pts',(130.705926064316,50.3963849653276,226.970325357774));
#87377=CARTESIAN_POINT('Ctrl Pts',(130.711726791672,50.3668025158223,226.977508176548));
#87378=CARTESIAN_POINT('Ctrl Pts',(130.717754981156,50.3360600588667,226.984972652975));
#87379=CARTESIAN_POINT('Ctrl Pts',(130.723895866631,50.3049288077942,226.990581437737));
#87380=CARTESIAN_POINT('Ctrl Pts',(130.730132469486,50.2735099108083,226.994338233717));
#87381=CARTESIAN_POINT('Ctrl Pts',(130.73636907234,50.2420910138223,226.998095029697));
#87382=CARTESIAN_POINT('Ctrl Pts',(130.742701591324,50.2103833747577,227.));
#87383=CARTESIAN_POINT('Ctrl Pts',(130.749115378049,50.178482477843,227.));
#87384=CARTESIAN_POINT('',(119.837845913371,50.178482477843,227.));
#87385=CARTESIAN_POINT('Origin',(125.29348064571,25.4505574462982,227.));
#87386=CARTESIAN_POINT('Ctrl Pts',(119.980756553526,50.9250708612662,226.3));
#87387=CARTESIAN_POINT('Ctrl Pts',(119.980756553526,50.9250708612662,226.330760525798));
#87388=CARTESIAN_POINT('Ctrl Pts',(119.980359541554,50.9228826666961,226.361320229286));
#87389=CARTESIAN_POINT('Ctrl Pts',(119.979587330222,50.918642522777,226.39147985655));
#87390=CARTESIAN_POINT('Ctrl Pts',(119.978786079618,50.9142429267913,226.422773646943));
#87391=CARTESIAN_POINT('Ctrl Pts',(119.97758088991,50.9076341444555,226.453637771802));
#87392=CARTESIAN_POINT('Ctrl Pts',(119.97598628326,50.898913553164,226.48386189553));
#87393=CARTESIAN_POINT('Ctrl Pts',(119.974422187669,50.8903598208746,226.513507713618));
#87394=CARTESIAN_POINT('Ctrl Pts',(119.972483366779,50.8797738865834,226.542538859668));
#87395=CARTESIAN_POINT('Ctrl Pts',(119.970174805301,50.8671999665045,226.570752225921));
#87396=CARTESIAN_POINT('Ctrl Pts',(119.969982103564,50.8661503881186,226.573107270269));
#87397=CARTESIAN_POINT('Ctrl Pts',(119.969786983124,50.8650878548648,226.575455559618));
#87398=CARTESIAN_POINT('Ctrl Pts',(119.96958943686,50.8640123484877,226.577797141023));
#87399=CARTESIAN_POINT('Ctrl Pts',(119.966196766862,50.8455415451015,226.618011583879));
#87400=CARTESIAN_POINT('Ctrl Pts',(119.962106793885,50.8233369857853,226.656038781937));
#87401=CARTESIAN_POINT('Ctrl Pts',(119.957332733188,50.7975628028764,226.691909536739));
#87402=CARTESIAN_POINT('Ctrl Pts',(119.953498572278,50.7768629477846,226.720718187204));
#87403=CARTESIAN_POINT('Ctrl Pts',(119.949209307764,50.7537894010272,226.748100234994));
#87404=CARTESIAN_POINT('Ctrl Pts',(119.944585796445,50.7290437736179,226.773441873749));
#87405=CARTESIAN_POINT('Ctrl Pts',(119.943048816176,50.720817657481,226.781866120184));
#87406=CARTESIAN_POINT('Ctrl Pts',(119.941474871115,50.7124065814287,226.790065256546));
#87407=CARTESIAN_POINT('Ctrl Pts',(119.939868307432,50.7038357163588,226.798017899287));
#87408=CARTESIAN_POINT('Ctrl Pts',(119.939373357799,50.7011952069503,226.800467946955));
#87409=CARTESIAN_POINT('Ctrl Pts',(119.938874561918,50.6985355852531,226.802898076406));
#87410=CARTESIAN_POINT('Ctrl Pts',(119.938372010707,50.6958573802167,226.80530808448));
#87411=CARTESIAN_POINT('Ctrl Pts',(119.933610160355,50.670480440854,226.828143762831));
#87412=CARTESIAN_POINT('Ctrl Pts',(119.928517223032,50.6434770554831,226.849139888348));
#87413=CARTESIAN_POINT('Ctrl Pts',(119.923155669031,50.6152163475391,226.868195456293));
#87414=CARTESIAN_POINT('Ctrl Pts',(119.917432532216,50.5850497395014,226.888536130357));
#87415=CARTESIAN_POINT('Ctrl Pts',(119.911403216501,50.5534497793912,226.906666565703));
#87416=CARTESIAN_POINT('Ctrl Pts',(119.905133396445,50.5208108759897,226.92244047314));
#87417=CARTESIAN_POINT('Ctrl Pts',(119.901430938444,50.5015369306507,226.931755290674));
#87418=CARTESIAN_POINT('Ctrl Pts',(119.897644428727,50.4818997258722,226.94024784624));
#87419=CARTESIAN_POINT('Ctrl Pts',(119.89378614051,50.4619741917207,226.947882574378));
#87420=CARTESIAN_POINT('Ctrl Pts',(119.887076253848,50.4273220174062,226.961160006656));
#87421=CARTESIAN_POINT('Ctrl Pts',(119.8800777526,50.391437659274,226.971955518833));
#87422=CARTESIAN_POINT('Ctrl Pts',(119.872890492327,50.3548503848194,226.98021787587));
#87423=CARTESIAN_POINT('Ctrl Pts',(119.865851227239,50.3190164906886,226.988310100059));
#87424=CARTESIAN_POINT('Ctrl Pts',(119.858630540141,50.2825064549341,226.993972516927));
#87425=CARTESIAN_POINT('Ctrl Pts',(119.851320043032,50.245811059138,226.997110112562));
#87426=CARTESIAN_POINT('Ctrl Pts',(119.846855087645,50.2233989984148,226.999026428829));
#87427=CARTESIAN_POINT('Ctrl Pts',(119.842356609805,50.2009177829365,227.));
#87428=CARTESIAN_POINT('Ctrl Pts',(119.837845913371,50.178482477843,227.));
#87429=CARTESIAN_POINT('Origin',(-190.5,58.8,211.4));
#87430=CARTESIAN_POINT('',(-190.,58.8,102.225104347671));
#87431=CARTESIAN_POINT('',(-189.999800857363,58.8,102.333498885934));
#87432=CARTESIAN_POINT('Origin',(-160.5,58.8,102.225104347671));
#87433=CARTESIAN_POINT('',(1.15828019241431E-14,58.8,195.5));
#87434=CARTESIAN_POINT('Ctrl Pts',(-189.999800857363,58.8,102.333498885934));
#87435=CARTESIAN_POINT('Ctrl Pts',(-189.98025109905,58.8,107.654006604893));
#87436=CARTESIAN_POINT('Ctrl Pts',(-189.93589337482,58.7999999999999,112.972770159136));
#87437=CARTESIAN_POINT('Ctrl Pts',(-189.816879937051,58.7999999999999,118.286284921046));
#87438=CARTESIAN_POINT('Ctrl Pts',(-189.757373218167,58.7999999999999,120.943042302001));
#87439=CARTESIAN_POINT('Ctrl Pts',(-189.678761610221,58.7999999999999,123.598456482408));
#87440=CARTESIAN_POINT('Ctrl Pts',(-189.570666695347,58.7999999999999,126.251797790585));
#87441=CARTESIAN_POINT('Ctrl Pts',(-189.462571780473,58.7999999999999,128.905139098762));
#87442=CARTESIAN_POINT('Ctrl Pts',(-189.325139639205,58.8,131.556417805139));
#87443=CARTESIAN_POINT('Ctrl Pts',(-189.143206561331,58.8,134.204567800212));
#87444=CARTESIAN_POINT('Ctrl Pts',(-188.961273483458,58.8,136.852717795285));
#87445=CARTESIAN_POINT('Ctrl Pts',(-188.735101605105,58.8,139.497757508966));
#87446=CARTESIAN_POINT('Ctrl Pts',(-188.441756887885,58.8,142.138074526077));
#87447=CARTESIAN_POINT('Ctrl Pts',(-188.148412170664,58.8,144.778391543189));
#87448=CARTESIAN_POINT('Ctrl Pts',(-187.788398583062,58.8,147.41402129609));
#87449=CARTESIAN_POINT('Ctrl Pts',(-187.325444057625,58.8,150.042413617553));
#87450=CARTESIAN_POINT('Ctrl Pts',(-187.093966794906,58.8,151.356609778285));
#87451=CARTESIAN_POINT('Ctrl Pts',(-186.83650703826,58.8,152.668979197212));
#87452=CARTESIAN_POINT('Ctrl Pts',(-186.546468546693,58.8,153.979058114737));
#87453=CARTESIAN_POINT('Ctrl Pts',(-186.256430055127,58.8,155.289137032263));
#87454=CARTESIAN_POINT('Ctrl Pts',(-185.933727730554,58.8,156.596161198099));
#87455=CARTESIAN_POINT('Ctrl Pts',(-185.574584035801,58.8,157.885628894788));
#87456=CARTESIAN_POINT('Ctrl Pts',(-184.856296646294,58.8,160.464564288164));
#87457=CARTESIAN_POINT('Ctrl Pts',(-183.99092543291,58.8,162.986625821545));
#87458=CARTESIAN_POINT('Ctrl Pts',(-182.913145481925,58.8,165.426553885135));
#87459=CARTESIAN_POINT('Ctrl Pts',(-182.374255506433,58.8,166.646517916931));
#87460=CARTESIAN_POINT('Ctrl Pts',(-181.781931362085,58.8,167.845820210719));
#87461=CARTESIAN_POINT('Ctrl Pts',(-181.12595295987,58.8,169.020508898055));
#87462=CARTESIAN_POINT('Ctrl Pts',(-180.797963758762,58.8,169.607853241724));
#87463=CARTESIAN_POINT('Ctrl Pts',(-180.452895188786,58.8,170.190776016641));
#87464=CARTESIAN_POINT('Ctrl Pts',(-180.094025945826,58.8,170.761526129557));
#87465=CARTESIAN_POINT('Ctrl Pts',(-179.735156702866,58.8,171.332276242472));
#87466=CARTESIAN_POINT('Ctrl Pts',(-179.362497837563,58.7999999999999,171.891096446703));
#87467=CARTESIAN_POINT('Ctrl Pts',(-178.975721840832,58.7999999999999,172.437703402131));
#87468=CARTESIAN_POINT('Ctrl Pts',(-177.428617853909,58.7999999999999,174.624131223845));
#87469=CARTESIAN_POINT('Ctrl Pts',(-175.653687288283,58.8,176.613457906034));
#87470=CARTESIAN_POINT('Ctrl Pts',(-173.645004150579,58.8,178.400556654236));
#87471=CARTESIAN_POINT('Ctrl Pts',(-173.142833366153,58.8,178.847331341286));
#87472=CARTESIAN_POINT('Ctrl Pts',(-172.624619471942,58.8,179.282785482727));
#87473=CARTESIAN_POINT('Ctrl Pts',(-172.095993754087,58.8,179.702765830952));
#87474=CARTESIAN_POINT('Ctrl Pts',(-171.567368036232,58.8,180.122746179177));
#87475=CARTESIAN_POINT('Ctrl Pts',(-171.029630345955,58.7999999999999,180.526399139266));
#87476=CARTESIAN_POINT('Ctrl Pts',(-170.483419960298,58.7999999999999,180.914870206751));
#87477=CARTESIAN_POINT('Ctrl Pts',(-169.390999188983,58.7999999999999,181.691812341722));
#87478=CARTESIAN_POINT('Ctrl Pts',(-168.264719930409,58.8,182.408084773304));
#87479=CARTESIAN_POINT('Ctrl Pts',(-167.109367700984,58.8,183.07226248173));
#87480=CARTESIAN_POINT('Ctrl Pts',(-164.798663242132,58.8,184.400617898584));
#87481=CARTESIAN_POINT('Ctrl Pts',(-162.372251203749,58.8,185.521641414205));
#87482=CARTESIAN_POINT('Ctrl Pts',(-159.861852893949,58.8,186.492173204115));
#87483=CARTESIAN_POINT('Ctrl Pts',(-158.606653739049,58.8,186.97743909907));
#87484=CARTESIAN_POINT('Ctrl Pts',(-157.337498640633,58.7999999999999,187.422033931911));
#87485=CARTESIAN_POINT('Ctrl Pts',(-156.060779329092,58.7999999999999,187.832008793431));
#87486=CARTESIAN_POINT('Ctrl Pts',(-154.784060017551,58.7999999999999,188.241983654951));
#87487=CARTESIAN_POINT('Ctrl Pts',(-153.498376682177,58.7999999999999,188.61784576423));
#87488=CARTESIAN_POINT('Ctrl Pts',(-152.205313605643,58.7999999999999,188.965624137122));
#87489=CARTESIAN_POINT('Ctrl Pts',(-149.619187452575,58.7999999999999,189.661180882907));
#87490=CARTESIAN_POINT('Ctrl Pts',(-147.003773115772,58.7999999999999,190.24528092407));
#87491=CARTESIAN_POINT('Ctrl Pts',(-144.368026627399,58.7999999999999,190.752006600492));
#87492=CARTESIAN_POINT('Ctrl Pts',(-143.050153383213,58.7999999999999,191.005369438703));
#87493=CARTESIAN_POINT('Ctrl Pts',(-141.726406587005,58.8,191.239238184733));
#87494=CARTESIAN_POINT('Ctrl Pts',(-140.40217354554,58.8,191.455987813524));
#87495=CARTESIAN_POINT('Ctrl Pts',(-139.077940504076,58.8,191.672737442316));
#87496=CARTESIAN_POINT('Ctrl Pts',(-137.752328543611,58.7999999999999,191.87255073608));
#87497=CARTESIAN_POINT('Ctrl Pts',(-136.425559458292,58.7999999999999,192.058151843066));
#87498=CARTESIAN_POINT('Ctrl Pts',(-133.772021287655,58.7999999999999,192.429354057037));
#87499=CARTESIAN_POINT('Ctrl Pts',(-131.113885005295,58.8,192.744080755892));
#87500=CARTESIAN_POINT('Ctrl Pts',(-128.45244324479,58.8,193.018208488718));
#87501=CARTESIAN_POINT('Ctrl Pts',(-123.129559723779,58.8,193.56646395437));
#87502=CARTESIAN_POINT('Ctrl Pts',(-117.793666862818,58.8,193.954934442914));
#87503=CARTESIAN_POINT('Ctrl Pts',(-112.450694014707,58.8,194.256446208796));
#87504=CARTESIAN_POINT('Ctrl Pts',(-107.107721166596,58.8,194.557957974678));
#87505=CARTESIAN_POINT('Ctrl Pts',(-101.757516044789,58.8,194.770640584592));
#87506=CARTESIAN_POINT('Ctrl Pts',(-96.4031808681222,58.8,194.932596507142));
#87507=CARTESIAN_POINT('Ctrl Pts',(-91.0488456914553,58.8,195.094552429692));
#87508=CARTESIAN_POINT('Ctrl Pts',(-85.6929541823069,58.8,195.204966816985));
#87509=CARTESIAN_POINT('Ctrl Pts',(-80.3374898338037,58.8,195.285751221278));
#87510=CARTESIAN_POINT('Ctrl Pts',(-74.9820254853004,58.8,195.366535625571));
#87511=CARTESIAN_POINT('Ctrl Pts',(-69.6263951900152,58.8,195.417356847769));
#87512=CARTESIAN_POINT('Ctrl Pts',(-64.2706727216169,58.8,195.451535386383));
#87513=CARTESIAN_POINT('Ctrl Pts',(-53.5592277848204,58.8,195.519892463612));
#87514=CARTESIAN_POINT('Ctrl Pts',(-42.8474268145233,58.8,195.523964494124));
#87515=CARTESIAN_POINT('Ctrl Pts',(-32.1355782419999,58.8,195.51944151511));
#87516=CARTESIAN_POINT('Ctrl Pts',(-21.4237296694766,58.8,195.514918536095));
#87517=CARTESIAN_POINT('Ctrl Pts',(-10.7118235226534,58.8,195.500000000149));
#87518=CARTESIAN_POINT('Ctrl Pts',(1.15828019241431E-14,58.8,195.5));
#87519=CARTESIAN_POINT('',(189.999800857363,58.8,102.333498885935));
#87520=CARTESIAN_POINT('Ctrl Pts',(8.88178419700125E-15,58.8,195.5));
#87521=CARTESIAN_POINT('Ctrl Pts',(10.6608822212759,58.8,195.500000000296));
#87522=CARTESIAN_POINT('Ctrl Pts',(21.3218250169713,58.8,195.514760894626));
#87523=CARTESIAN_POINT('Ctrl Pts',(31.9827261779419,58.8,195.51937615705));
#87524=CARTESIAN_POINT('Ctrl Pts',(42.6436273389126,58.8,195.523991419473));
#87525=CARTESIAN_POINT('Ctrl Pts',(53.3044940402517,58.8,195.520209490269));
#87526=CARTESIAN_POINT('Ctrl Pts',(63.9651023694078,58.8,195.453466915477));
#87527=CARTESIAN_POINT('Ctrl Pts',(69.2954065339858,58.8,195.420095628081));
#87528=CARTESIAN_POINT('Ctrl Pts',(74.6256438146957,58.8,195.370425946996));
#87529=CARTESIAN_POINT('Ctrl Pts',(79.9557608635996,58.8,195.291457941204));
#87530=CARTESIAN_POINT('Ctrl Pts',(85.2858779125034,58.8,195.212489935411));
#87531=CARTESIAN_POINT('Ctrl Pts',(90.617169770423,58.8,195.10450581883));
#87532=CARTESIAN_POINT('Ctrl Pts',(95.9430357498042,58.8,194.946385956025));
#87533=CARTESIAN_POINT('Ctrl Pts',(101.268901729185,58.8,194.78826609322));
#87534=CARTESIAN_POINT('Ctrl Pts',(106.58996338726,58.8,194.580711495765));
#87535=CARTESIAN_POINT('Ctrl Pts',(111.902657189983,58.8,194.287054682287));
#87536=CARTESIAN_POINT('Ctrl Pts',(117.215350992707,58.8,193.993397868808));
#87537=CARTESIAN_POINT('Ctrl Pts',(122.519844509403,58.8,193.615363067472));
#87538=CARTESIAN_POINT('Ctrl Pts',(127.809401981597,58.8,193.083641750981));
#87539=CARTESIAN_POINT('Ctrl Pts',(130.454180717694,58.8,192.817781092736));
#87540=CARTESIAN_POINT('Ctrl Pts',(133.095165732892,58.8,192.512884413637));
#87541=CARTESIAN_POINT('Ctrl Pts',(135.730906077612,58.8,192.154021965476));
#87542=CARTESIAN_POINT('Ctrl Pts',(138.366646422331,58.8,191.795159517316));
#87543=CARTESIAN_POINT('Ctrl Pts',(140.997169684096,58.8000000000001,191.382615165556));
#87544=CARTESIAN_POINT('Ctrl Pts',(143.620258990582,58.8000000000001,190.893578093325));
#87545=CARTESIAN_POINT('Ctrl Pts',(146.243348297067,58.8000000000001,190.404541021094));
#87546=CARTESIAN_POINT('Ctrl Pts',(148.859060109816,58.8,189.839592196665));
#87547=CARTESIAN_POINT('Ctrl Pts',(151.463804706251,58.8,189.161794669432));
#87548=CARTESIAN_POINT('Ctrl Pts',(152.766177004469,58.8,188.822895905815));
#87549=CARTESIAN_POINT('Ctrl Pts',(154.063722484329,58.8,188.455855238128));
#87550=CARTESIAN_POINT('Ctrl Pts',(155.345610999807,58.8,188.057834736658));
#87551=CARTESIAN_POINT('Ctrl Pts',(156.627499515284,58.8,187.659814235188));
#87552=CARTESIAN_POINT('Ctrl Pts',(157.896230834775,58.8,187.230200792086));
#87553=CARTESIAN_POINT('Ctrl Pts',(159.149225485557,58.8,186.762800600376));
#87554=CARTESIAN_POINT('Ctrl Pts',(161.655214787121,58.8,185.828000216956));
#87555=CARTESIAN_POINT('Ctrl Pts',(164.099002476109,58.8,184.743841876054));
#87556=CARTESIAN_POINT('Ctrl Pts',(166.452402824297,58.8,183.442646258576));
#87557=CARTESIAN_POINT('Ctrl Pts',(167.040752911344,58.8,183.117347354207));
#87558=CARTESIAN_POINT('Ctrl Pts',(167.623396019085,58.8,182.778344901958));
#87559=CARTESIAN_POINT('Ctrl Pts',(168.19976750543,58.8,182.42428308841));
#87560=CARTESIAN_POINT('Ctrl Pts',(168.776138991775,58.8,182.070221274862));
#87561=CARTESIAN_POINT('Ctrl Pts',(169.345685170054,58.8,181.701285645968));
#87562=CARTESIAN_POINT('Ctrl Pts',(169.901687100616,58.8,181.320740058355));
#87563=CARTESIAN_POINT('Ctrl Pts',(171.013690961741,58.8,180.559648883128));
#87564=CARTESIAN_POINT('Ctrl Pts',(172.078138682642,58.8,179.748063563893));
#87565=CARTESIAN_POINT('Ctrl Pts',(173.091864655936,58.8,178.882622922976));
#87566=CARTESIAN_POINT('Ctrl Pts',(175.119316602522,58.8,177.151741641143));
#87567=CARTESIAN_POINT('Ctrl Pts',(176.942436203403,58.8,175.203904423765));
#87568=CARTESIAN_POINT('Ctrl Pts',(178.549784955921,58.8,173.026966100971));
#87569=CARTESIAN_POINT('Ctrl Pts',(178.951622144051,58.8,172.482731520272));
#87570=CARTESIAN_POINT('Ctrl Pts',(179.340199864675,58.8,171.923832776685));
#87571=CARTESIAN_POINT('Ctrl Pts',(179.710556657438,58.8,171.358822781541));
#87572=CARTESIAN_POINT('Ctrl Pts',(180.080913450202,58.8,170.793812786397));
#87573=CARTESIAN_POINT('Ctrl Pts',(180.434508985294,58.8,170.220810507793));
#87574=CARTESIAN_POINT('Ctrl Pts',(180.772486437532,58.8,169.640361046698));
#87575=CARTESIAN_POINT('Ctrl Pts',(181.44844134201,58.8,168.47946212451));
#87576=CARTESIAN_POINT('Ctrl Pts',(182.061965606304,58.8,167.288794351923));
#87577=CARTESIAN_POINT('Ctrl Pts',(182.621837291323,58.8,166.072543378534));
#87578=CARTESIAN_POINT('Ctrl Pts',(183.181708976343,58.8,164.856292405145));
#87579=CARTESIAN_POINT('Ctrl Pts',(183.68794311769,58.8,163.614465400397));
#87580=CARTESIAN_POINT('Ctrl Pts',(184.148570796702,58.8,162.350891830973));
#87581=CARTESIAN_POINT('Ctrl Pts',(184.609198475714,58.8,161.087318261549));
#87582=CARTESIAN_POINT('Ctrl Pts',(185.025180861451,58.8,159.798417119322));
#87583=CARTESIAN_POINT('Ctrl Pts',(185.399766833237,58.8,158.501874284172));
#87584=CARTESIAN_POINT('Ctrl Pts',(186.148938776808,58.8,155.908788613871));
#87585=CARTESIAN_POINT('Ctrl Pts',(186.736003435447,58.8,153.285009470254));
#87586=CARTESIAN_POINT('Ctrl Pts',(187.218096335368,58.8,150.641354922102));
#87587=CARTESIAN_POINT('Ctrl Pts',(187.70018923529,58.8,147.99770037395));
#87588=CARTESIAN_POINT('Ctrl Pts',(188.076546005177,58.8,145.334025694806));
#87589=CARTESIAN_POINT('Ctrl Pts',(188.383194380381,58.8,142.657152393827));
#87590=CARTESIAN_POINT('Ctrl Pts',(188.689842755585,58.8,139.980279092848));
#87591=CARTESIAN_POINT('Ctrl Pts',(188.925895877108,58.8,137.293871517216));
#87592=CARTESIAN_POINT('Ctrl Pts',(189.115096080232,58.8,134.608587766533));
#87593=CARTESIAN_POINT('Ctrl Pts',(189.304296283357,58.8,131.923304015851));
#87594=CARTESIAN_POINT('Ctrl Pts',(189.446683812067,58.8,129.236274241946));
#87595=CARTESIAN_POINT('Ctrl Pts',(189.558470527221,58.8,126.548103116225));
#87596=CARTESIAN_POINT('Ctrl Pts',(189.670257242375,58.8,123.859931990504));
#87597=CARTESIAN_POINT('Ctrl Pts',(189.751276588566,58.8,121.170613300767));
#87598=CARTESIAN_POINT('Ctrl Pts',(189.812493834118,58.8,118.480556030551));
#87599=CARTESIAN_POINT('Ctrl Pts',(189.934928325222,58.8,113.100441490117));
#87600=CARTESIAN_POINT('Ctrl Pts',(189.980018010671,58.8,107.717442136363));
#87601=CARTESIAN_POINT('Ctrl Pts',(189.999800857363,58.8,102.333498885935));
#87602=CARTESIAN_POINT('',(190.,58.8,102.225104347672));
#87603=CARTESIAN_POINT('Origin',(160.5,58.8,102.225104347672));
#87604=CARTESIAN_POINT('',(190.,58.8,40.5));
#87605=CARTESIAN_POINT('',(190.,58.8,211.4));
#87606=CARTESIAN_POINT('',(-190.,58.8,40.5));
#87607=CARTESIAN_POINT('',(-190.5,58.8,40.5));
#87608=CARTESIAN_POINT('',(-190.,58.8,211.4));
#87609=CARTESIAN_POINT('Origin',(-160.5,51.6013867006571,102.225104347671));
#87610=CARTESIAN_POINT('',(-190.499797482064,58.2999999999999,102.335336081498));
#87611=CARTESIAN_POINT('',(-190.499797482064,55.3,102.335336081498));
#87612=CARTESIAN_POINT('',(-190.499797482064,58.8,102.335336081498));
#87613=CARTESIAN_POINT('',(-190.5,58.2999999999999,102.225104347671));
#87614=CARTESIAN_POINT('Origin',(-160.5,58.3,102.225104347671));
#87615=CARTESIAN_POINT('',(-190.5,55.3,102.225104347671));
#87616=CARTESIAN_POINT('',(-190.5,58.8,102.225104347671));
#87617=CARTESIAN_POINT('Origin',(-160.5,55.3,102.225104347671));
#87618=CARTESIAN_POINT('Ctrl Pts',(-190.499797482064,55.2999999999999,102.335336081498));
#87619=CARTESIAN_POINT('Ctrl Pts',(-190.499797482064,58.9,102.335336081498));
#87620=CARTESIAN_POINT('Ctrl Pts',(-190.141509581597,55.2999999999999,199.844139409912));
#87621=CARTESIAN_POINT('Ctrl Pts',(-190.141509581597,58.9,199.844139409912));
#87622=CARTESIAN_POINT('Ctrl Pts',(-180.969631132311,55.2999999999999,196.));
#87623=CARTESIAN_POINT('Ctrl Pts',(-180.969631132311,58.9,196.));
#87624=CARTESIAN_POINT('Ctrl Pts',(1.20290037631083E-14,55.3,196.));
#87625=CARTESIAN_POINT('Ctrl Pts',(1.20290037631083E-14,58.9,196.));
#87626=CARTESIAN_POINT('',(1.20290037631083E-14,55.3,196.));
#87627=CARTESIAN_POINT('',(1.16465450439953E-14,58.3,196.));
#87628=CARTESIAN_POINT('',(3.34339434094657E-14,-112.6,196.));
#87629=CARTESIAN_POINT('Ctrl Pts',(1.16465450439953E-14,58.3,196.));
#87630=CARTESIAN_POINT('Ctrl Pts',(-10.7117531408873,58.3,196.));
#87631=CARTESIAN_POINT('Ctrl Pts',(-21.4235888453057,58.3000000000004,196.014918521175));
#87632=CARTESIAN_POINT('Ctrl Pts',(-32.1353671216415,58.3000000000002,196.019441470522));
#87633=CARTESIAN_POINT('Ctrl Pts',(-37.9435658896329,58.3000000000001,196.021893928756));
#87634=CARTESIAN_POINT('Ctrl Pts',(-43.7517506038881,58.3000000000219,196.02182007439));
#87635=CARTESIAN_POINT('Ctrl Pts',(-49.5598722236178,58.3000000000338,196.010342241869));
#87636=CARTESIAN_POINT('Ctrl Pts',(-54.4645909813284,58.3000000000439,196.000649686488));
#87637=CARTESIAN_POINT('Ctrl Pts',(-59.3692646648713,58.300000000047,195.982824814488));
#87638=CARTESIAN_POINT('Ctrl Pts',(-64.2738634995991,58.3000000000241,195.951525205213));
#87639=CARTESIAN_POINT('Ctrl Pts',(-69.6310359294076,58.299999999999,195.917337413403));
#87640=CARTESIAN_POINT('Ctrl Pts',(-74.9881325496685,58.3000000000011,195.866500385808));
#87641=CARTESIAN_POINT('Ctrl Pts',(-80.3450312167436,58.3000000000005,195.785694345575));
#87642=CARTESIAN_POINT('Ctrl Pts',(-82.3276213464493,58.3000000000003,195.755788000926));
#87643=CARTESIAN_POINT('Ctrl Pts',(-84.3102735136791,58.2999999999996,195.721822619659));
#87644=CARTESIAN_POINT('Ctrl Pts',(-86.2928865664701,58.2999999999997,195.68268720698));
#87645=CARTESIAN_POINT('Ctrl Pts',(-89.6683095657664,58.3,195.616058687683));
#87646=CARTESIAN_POINT('Ctrl Pts',(-93.0436168853548,58.3000000000031,195.534444015978));
#87647=CARTESIAN_POINT('Ctrl Pts',(-96.4182977668297,58.3000000000172,195.432367934214));
#87648=CARTESIAN_POINT('Ctrl Pts',(-99.0028780309804,58.300000000028,195.354190519628));
#87649=CARTESIAN_POINT('Ctrl Pts',(-101.58649661917,58.3000000000233,195.264202002625));
#87650=CARTESIAN_POINT('Ctrl Pts',(-104.168805586391,58.3000000000169,195.158122276966));
#87651=CARTESIAN_POINT('Ctrl Pts',(-106.940478976983,58.30000000001,195.044263572752));
#87652=CARTESIAN_POINT('Ctrl Pts',(-109.710642796453,58.3,194.911866797889));
#87653=CARTESIAN_POINT('Ctrl Pts',(-112.478864925773,58.3,194.755651977743));
#87654=CARTESIAN_POINT('Ctrl Pts',(-114.594746753345,58.3,194.636249674133));
#87655=CARTESIAN_POINT('Ctrl Pts',(-116.709518796986,58.3000000000003,194.50322857681));
#87656=CARTESIAN_POINT('Ctrl Pts',(-118.822815220673,58.3000000000008,194.352073391081));
#87657=CARTESIAN_POINT('Ctrl Pts',(-121.558136194221,58.3000000000013,194.156427411107));
#87658=CARTESIAN_POINT('Ctrl Pts',(-124.290983473982,58.3000000000019,193.930399062793));
#87659=CARTESIAN_POINT('Ctrl Pts',(-127.020560439236,58.3000000000014,193.664236652735));
#87660=CARTESIAN_POINT('Ctrl Pts',(-127.515039874691,58.3000000000013,193.61601971658));
#87661=CARTESIAN_POINT('Ctrl Pts',(-128.009411994897,58.3000000000012,193.566485817347));
#87662=CARTESIAN_POINT('Ctrl Pts',(-128.503672075522,58.300000000001,193.515577171767));
#87663=CARTESIAN_POINT('Ctrl Pts',(-130.44029839942,58.3000000000004,193.316105219635));
#87664=CARTESIAN_POINT('Ctrl Pts',(-132.375178704953,58.3000000000097,193.09517822546));
#87665=CARTESIAN_POINT('Ctrl Pts',(-134.307814874518,58.3000000000101,192.846714080737));
#87666=CARTESIAN_POINT('Ctrl Pts',(-135.037148072975,58.3000000000103,192.752949329654));
#87667=CARTESIAN_POINT('Ctrl Pts',(-135.766161858712,58.3000000000092,192.655263232269));
#87668=CARTESIAN_POINT('Ctrl Pts',(-136.494829730514,58.3000000000057,192.553330224408));
#87669=CARTESIAN_POINT('Ctrl Pts',(-136.887919456177,58.3000000000039,192.498341086494));
#87670=CARTESIAN_POINT('Ctrl Pts',(-137.280910057353,58.3000000000028,192.442107471789));
#87671=CARTESIAN_POINT('Ctrl Pts',(-137.673799736929,58.3000000000017,192.384558364539));
#87672=CARTESIAN_POINT('Ctrl Pts',(-138.610834557934,58.2999999999991,192.247304778573));
#87673=CARTESIAN_POINT('Ctrl Pts',(-139.547276794965,58.299999999998,192.10257023963));
#87674=CARTESIAN_POINT('Ctrl Pts',(-140.482938496475,58.3000000000027,191.949421722643));
#87675=CARTESIAN_POINT('Ctrl Pts',(-140.735750537704,58.300000000004,191.908041607235));
#87676=CARTESIAN_POINT('Ctrl Pts',(-140.988534787172,58.3000000000047,191.866041232622));
#87677=CARTESIAN_POINT('Ctrl Pts',(-141.241276754389,58.300000000005,191.823400409433));
#87678=CARTESIAN_POINT('Ctrl Pts',(-142.316874391201,58.3000000000062,191.641933242905));
#87679=CARTESIAN_POINT('Ctrl Pts',(-143.391615355279,58.3000000000001,191.448879234469));
#87680=CARTESIAN_POINT('Ctrl Pts',(-144.462423620222,58.3000000000008,191.243014958559));
#87681=CARTESIAN_POINT('Ctrl Pts',(-144.849418251539,58.300000000001,191.16861473943));
#87682=CARTESIAN_POINT('Ctrl Pts',(-145.235966544853,58.3000000000006,191.092555291249));
#87683=CARTESIAN_POINT('Ctrl Pts',(-145.622053820955,58.3000000000003,191.014726875239));
#87684=CARTESIAN_POINT('Ctrl Pts',(-147.026899875961,58.2999999999989,190.731534576587));
#87685=CARTESIAN_POINT('Ctrl Pts',(-148.425594601788,58.2999999999958,190.424926449121));
#87686=CARTESIAN_POINT('Ctrl Pts',(-149.816784842427,58.2999999999984,190.089768387871));
#87687=CARTESIAN_POINT('Ctrl Pts',(-150.659099143544,58.2999999999999,189.886842562288));
#87688=CARTESIAN_POINT('Ctrl Pts',(-151.498662614194,58.3000000000036,189.673451611131));
#87689=CARTESIAN_POINT('Ctrl Pts',(-152.33517708753,58.3000000000109,189.448465183433));
#87690=CARTESIAN_POINT('Ctrl Pts',(-152.632968472974,58.3000000000135,189.368372104178));
#87691=CARTESIAN_POINT('Ctrl Pts',(-152.930371233519,58.3000000000145,189.286797584502));
#87692=CARTESIAN_POINT('Ctrl Pts',(-153.227374012079,58.3000000000153,189.203666691527));
#87693=CARTESIAN_POINT('Ctrl Pts',(-154.162302092042,58.300000000018,188.941980903497));
#87694=CARTESIAN_POINT('Ctrl Pts',(-155.093230771767,58.3000000000155,188.664878377644));
#87695=CARTESIAN_POINT('Ctrl Pts',(-156.019362355789,58.3000000000071,188.370172325877));
#87696=CARTESIAN_POINT('Ctrl Pts',(-156.084148129711,58.3000000000066,188.349556724409));
#87697=CARTESIAN_POINT('Ctrl Pts',(-156.148910434322,58.3000000000059,188.328855002121));
#87698=CARTESIAN_POINT('Ctrl Pts',(-156.213648998875,58.3000000000053,188.308066420174));
#87699=CARTESIAN_POINT('Ctrl Pts',(-156.416564742649,58.3000000000033,188.242906949971));
#87700=CARTESIAN_POINT('Ctrl Pts',(-156.619277404117,58.300000000003,188.176883122836));
#87701=CARTESIAN_POINT('Ctrl Pts',(-156.821789346548,58.300000000003,188.109962018534));
#87702=CARTESIAN_POINT('Ctrl Pts',(-157.674439750132,58.3000000000032,187.82819934367));
#87703=CARTESIAN_POINT('Ctrl Pts',(-158.523442517442,58.3000000000126,187.530554246495));
#87704=CARTESIAN_POINT('Ctrl Pts',(-159.366711643314,58.3000000000119,187.215315791802));
#87705=CARTESIAN_POINT('Ctrl Pts',(-159.592281256958,58.3000000000117,187.130991328533));
#87706=CARTESIAN_POINT('Ctrl Pts',(-159.817440715442,58.3000000000108,187.045408267945));
#87707=CARTESIAN_POINT('Ctrl Pts',(-160.042150350673,58.3000000000089,186.958534466439));
#87708=CARTESIAN_POINT('Ctrl Pts',(-160.341043439003,58.3000000000062,186.842980993174));
#87709=CARTESIAN_POINT('Ctrl Pts',(-160.638745189105,58.3000000000063,186.725316023782));
#87710=CARTESIAN_POINT('Ctrl Pts',(-160.93521712623,58.3000000000063,186.605440004865));
#87711=CARTESIAN_POINT('Ctrl Pts',(-162.043912968536,58.3000000000061,186.157147849276));
#87712=CARTESIAN_POINT('Ctrl Pts',(-163.135358586009,58.3000000000134,185.67794905054));
#87713=CARTESIAN_POINT('Ctrl Pts',(-164.206821638704,58.3000000000175,185.16295321028));
#87714=CARTESIAN_POINT('Ctrl Pts',(-165.21381224214,58.3000000000213,184.678945879701));
#87715=CARTESIAN_POINT('Ctrl Pts',(-166.203152864415,58.3000000000223,184.163320138608));
#87716=CARTESIAN_POINT('Ctrl Pts',(-167.172600014669,58.3000000000118,183.612061847702));
#87717=CARTESIAN_POINT('Ctrl Pts',(-167.234668748967,58.3000000000112,183.576767603576));
#87718=CARTESIAN_POINT('Ctrl Pts',(-167.296655944745,58.3000000000105,183.541327310698));
#87719=CARTESIAN_POINT('Ctrl Pts',(-167.358561016714,58.3000000000097,183.505739922036));
#87720=CARTESIAN_POINT('Ctrl Pts',(-168.394805402409,58.2999999999968,182.910033778262));
#87721=CARTESIAN_POINT('Ctrl Pts',(-169.407907923029,58.3000000000085,182.272891065632));
#87722=CARTESIAN_POINT('Ctrl Pts',(-170.394542881228,58.3000000000045,181.588329914564));
#87723=CARTESIAN_POINT('Ctrl Pts',(-170.521203484904,58.300000000004,181.500448446422));
#87724=CARTESIAN_POINT('Ctrl Pts',(-170.647427870475,58.3000000000033,181.411785539936));
#87725=CARTESIAN_POINT('Ctrl Pts',(-170.77320899952,58.3000000000023,181.322328563753));
#87726=CARTESIAN_POINT('Ctrl Pts',(-170.892813072123,58.3000000000014,181.237264780691));
#87727=CARTESIAN_POINT('Ctrl Pts',(-171.012017677299,58.3000000000012,181.151481007302));
#87728=CARTESIAN_POINT('Ctrl Pts',(-171.130802553357,58.300000000001,181.064975844131));
#87729=CARTESIAN_POINT('Ctrl Pts',(-171.508826193717,58.3000000000003,180.789679882414));
#87730=CARTESIAN_POINT('Ctrl Pts',(-171.882642934083,58.3000000000006,180.507051767321));
#87731=CARTESIAN_POINT('Ctrl Pts',(-172.252308609757,58.3000000000003,180.216507805986));
#87732=CARTESIAN_POINT('Ctrl Pts',(-172.303960387306,58.3000000000002,180.175911361559));
#87733=CARTESIAN_POINT('Ctrl Pts',(-172.355531082787,58.3000000000002,180.135160300748));
#87734=CARTESIAN_POINT('Ctrl Pts',(-172.407020808966,58.3000000000001,180.094252958564));
#87735=CARTESIAN_POINT('Ctrl Pts',(-172.455054775942,58.3,180.056091133491));
#87736=CARTESIAN_POINT('Ctrl Pts',(-172.503007691249,58.3,180.017800246934));
#87737=CARTESIAN_POINT('Ctrl Pts',(-172.550875975171,58.3,179.979382822756));
#87738=CARTESIAN_POINT('Ctrl Pts',(-172.597530076584,58.3,179.94193985934));
#87739=CARTESIAN_POINT('Ctrl Pts',(-172.644097658298,58.3,179.904381602751));
#87740=CARTESIAN_POINT('Ctrl Pts',(-172.690571407457,58.3,179.866713790957));
#87741=CARTESIAN_POINT('Ctrl Pts',(-173.036090106872,58.3000000000001,179.586664654043));
#87742=CARTESIAN_POINT('Ctrl Pts',(-173.37649834377,58.3000000000002,179.300504243075));
#87743=CARTESIAN_POINT('Ctrl Pts',(-173.710509907641,58.3000000000002,179.00917403755));
#87744=CARTESIAN_POINT('Ctrl Pts',(-173.799924383646,58.3000000000003,178.93118530755));
#87745=CARTESIAN_POINT('Ctrl Pts',(-173.888880292515,58.3000000000003,178.85282585907));
#87746=CARTESIAN_POINT('Ctrl Pts',(-173.977352529315,58.3000000000003,178.77411328332));
#87747=CARTESIAN_POINT('Ctrl Pts',(-174.08688548205,58.3000000000003,178.676663267914));
#87748=CARTESIAN_POINT('Ctrl Pts',(-174.195746814185,58.3000000000004,178.578606695465));
#87749=CARTESIAN_POINT('Ctrl Pts',(-174.303919105548,58.3000000000005,178.47996099629));
#87750=CARTESIAN_POINT('Ctrl Pts',(-174.958585105133,58.3000000000017,177.882950574851));
#87751=CARTESIAN_POINT('Ctrl Pts',(-175.588161570033,58.3000000000061,177.264237400956));
#87752=CARTESIAN_POINT('Ctrl Pts',(-176.192889049001,58.3000000000103,176.624027669967));
#87753=CARTESIAN_POINT('Ctrl Pts',(-176.801495037263,58.3000000000146,175.979711859004));
#87754=CARTESIAN_POINT('Ctrl Pts',(-177.384932288338,58.3000000000186,175.313622817443));
#87755=CARTESIAN_POINT('Ctrl Pts',(-177.94340602101,58.3000000000187,174.625935950806));
#87756=CARTESIAN_POINT('Ctrl Pts',(-178.443543937974,58.3000000000188,174.010081960041));
#87757=CARTESIAN_POINT('Ctrl Pts',(-178.92366058504,58.3000000000158,173.376906024021));
#87758=CARTESIAN_POINT('Ctrl Pts',(-179.383876297428,58.3000000000071,172.726511192076));
#87759=CARTESIAN_POINT('Ctrl Pts',(-179.775881961455,58.2999999999996,172.172513466414));
#87760=CARTESIAN_POINT('Ctrl Pts',(-180.153586615474,58.2999999999989,171.606136536173));
#87761=CARTESIAN_POINT('Ctrl Pts',(-180.517306782578,58.3000000000017,171.027671453041));
#87762=CARTESIAN_POINT('Ctrl Pts',(-180.773257891743,58.3000000000037,170.620603621693));
#87763=CARTESIAN_POINT('Ctrl Pts',(-181.02228224259,58.3000000000012,170.207421559621));
#87764=CARTESIAN_POINT('Ctrl Pts',(-181.263216377716,58.3000000000022,169.790863880058));
#87765=CARTESIAN_POINT('Ctrl Pts',(-181.364433854457,58.3000000000026,169.615866189419));
#87766=CARTESIAN_POINT('Ctrl Pts',(-181.464223374814,58.3000000000036,169.440272954189));
#87767=CARTESIAN_POINT('Ctrl Pts',(-181.562498312604,58.3000000000056,169.264287803901));
#87768=CARTESIAN_POINT('Ctrl Pts',(-181.963798132055,58.3000000000141,168.545662988413));
#87769=CARTESIAN_POINT('Ctrl Pts',(-182.341570768327,58.3000000000098,167.817936557716));
#87770=CARTESIAN_POINT('Ctrl Pts',(-182.698077172536,58.3000000000056,167.081982270718));
#87771=CARTESIAN_POINT('Ctrl Pts',(-182.931096083592,58.3000000000029,166.600949491171));
#87772=CARTESIAN_POINT('Ctrl Pts',(-183.155029793797,58.3,166.11640183649));
#87773=CARTESIAN_POINT('Ctrl Pts',(-183.370511496512,58.3,165.628584399065));
#87774=CARTESIAN_POINT('Ctrl Pts',(-183.755752982814,58.3,164.756456917848));
#87775=CARTESIAN_POINT('Ctrl Pts',(-184.114155312767,58.3,163.873945558567));
#87776=CARTESIAN_POINT('Ctrl Pts',(-184.448595069682,58.3000000000002,162.982163713652));
#87777=CARTESIAN_POINT('Ctrl Pts',(-184.791126443434,58.3000000000005,162.068805615186));
#87778=CARTESIAN_POINT('Ctrl Pts',(-185.108521692177,58.3000000000011,161.145723081237));
#87779=CARTESIAN_POINT('Ctrl Pts',(-185.403902451678,58.3000000000022,160.21412405169));
#87780=CARTESIAN_POINT('Ctrl Pts',(-185.613943251761,58.300000000003,159.551678041825));
#87781=CARTESIAN_POINT('Ctrl Pts',(-185.812853271099,58.300000000004,158.884925982554));
#87782=CARTESIAN_POINT('Ctrl Pts',(-186.001763980044,58.3000000000055,158.214305556729));
#87783=CARTESIAN_POINT('Ctrl Pts',(-186.020019206364,58.3000000000056,158.149500720008));
#87784=CARTESIAN_POINT('Ctrl Pts',(-186.038181070206,58.3000000000058,158.084659736397));
#87785=CARTESIAN_POINT('Ctrl Pts',(-186.056250572068,58.3000000000059,158.019783088719));
#87786=CARTESIAN_POINT('Ctrl Pts',(-186.248767774588,58.3000000000077,157.32857030296));
#87787=CARTESIAN_POINT('Ctrl Pts',(-186.430890237263,58.3000000000059,156.632353763643));
#87788=CARTESIAN_POINT('Ctrl Pts',(-186.603184824574,58.3000000000038,155.93332206803));
#87789=CARTESIAN_POINT('Ctrl Pts',(-186.726566962198,58.3000000000024,155.432737422754));
#87790=CARTESIAN_POINT('Ctrl Pts',(-186.844909305794,58.3000000000008,154.930709352884));
#87791=CARTESIAN_POINT('Ctrl Pts',(-186.958421382134,58.3000000000002,154.428044798887));
#87792=CARTESIAN_POINT('Ctrl Pts',(-186.984076158333,58.3000000000001,154.314437973502));
#87793=CARTESIAN_POINT('Ctrl Pts',(-187.009484242047,58.3,154.200798493157));
#87794=CARTESIAN_POINT('Ctrl Pts',(-187.034647948172,58.3000000000001,154.087136197121));
#87795=CARTESIAN_POINT('Ctrl Pts',(-187.249235323321,58.3000000000005,153.117863481938));
#87796=CARTESIAN_POINT('Ctrl Pts',(-187.446091763184,58.3000000000003,152.147365334446));
#87797=CARTESIAN_POINT('Ctrl Pts',(-187.627848879965,58.3000000000049,151.175800942874));
#87798=CARTESIAN_POINT('Ctrl Pts',(-187.693091881787,58.3000000000065,150.827051036998));
#87799=CARTESIAN_POINT('Ctrl Pts',(-187.756389540824,58.3000000000085,150.478163535845));
#87800=CARTESIAN_POINT('Ctrl Pts',(-187.817864007364,58.3000000000118,150.129146500694));
#87801=CARTESIAN_POINT('Ctrl Pts',(-188.069630134647,58.3000000000257,148.699761713139));
#87802=CARTESIAN_POINT('Ctrl Pts',(-188.291104381093,58.300000000021,147.268244389129));
#87803=CARTESIAN_POINT('Ctrl Pts',(-188.488029483918,58.3000000000165,145.834998732404));
#87804=CARTESIAN_POINT('Ctrl Pts',(-188.654658778524,58.3000000000128,144.622249776835));
#87805=CARTESIAN_POINT('Ctrl Pts',(-188.803712708488,58.3000000000085,143.408263442865));
#87806=CARTESIAN_POINT('Ctrl Pts',(-188.938699247615,58.3000000000175,142.193285856765));
#87807=CARTESIAN_POINT('Ctrl Pts',(-189.136760752398,58.3000000000306,140.410587444496));
#87808=CARTESIAN_POINT('Ctrl Pts',(-189.304299635183,58.3000000000179,138.625740791404));
#87809=CARTESIAN_POINT('Ctrl Pts',(-189.448306843471,58.300000000011,136.83923745387));
#87810=CARTESIAN_POINT('Ctrl Pts',(-189.518148309857,58.3000000000076,135.972808514095));
#87811=CARTESIAN_POINT('Ctrl Pts',(-189.582455698063,58.3000000000052,135.105989966169));
#87812=CARTESIAN_POINT('Ctrl Pts',(-189.642030732453,58.3000000000086,134.238837995223));
#87813=CARTESIAN_POINT('Ctrl Pts',(-189.792507729526,58.3000000000171,132.048550974295));
#87814=CARTESIAN_POINT('Ctrl Pts',(-189.912606188582,58.3000000000056,129.85612495635));
#87815=CARTESIAN_POINT('Ctrl Pts',(-190.010855650094,58.3000000000114,127.66216080368));
#87816=CARTESIAN_POINT('Ctrl Pts',(-190.031601675758,58.3000000000126,127.198890716326));
#87817=CARTESIAN_POINT('Ctrl Pts',(-190.05137369699,58.3000000000145,126.73555206654));
#87818=CARTESIAN_POINT('Ctrl Pts',(-190.070252291175,58.3000000000178,126.272150491644));
#87819=CARTESIAN_POINT('Ctrl Pts',(-190.155978461159,58.3000000000328,124.167881402989));
#87820=CARTESIAN_POINT('Ctrl Pts',(-190.223187158372,58.3000000000361,122.062308228899));
#87821=CARTESIAN_POINT('Ctrl Pts',(-190.277034713559,58.3000000000306,119.955794495884));
#87822=CARTESIAN_POINT('Ctrl Pts',(-190.291163272368,58.3000000000292,119.403085964254));
#87823=CARTESIAN_POINT('Ctrl Pts',(-190.304372107163,58.300000000027,118.850312644463));
#87824=CARTESIAN_POINT('Ctrl Pts',(-190.316754563799,58.3000000000245,118.297481238444));
#87825=CARTESIAN_POINT('Ctrl Pts',(-190.39715529836,58.3000000000085,114.707882466758));
#87826=CARTESIAN_POINT('Ctrl Pts',(-190.443516404958,58.300000000003,111.115886215597));
#87827=CARTESIAN_POINT('Ctrl Pts',(-190.471166980605,58.300000000001,107.522572735381));
#87828=CARTESIAN_POINT('Ctrl Pts',(-190.484470219448,58.3000000000001,105.793758548108));
#87829=CARTESIAN_POINT('Ctrl Pts',(-190.493443302044,58.3,104.064639496642));
#87830=CARTESIAN_POINT('Ctrl Pts',(-190.499797482064,58.3,102.335336081498));
#87831=CARTESIAN_POINT('Ctrl Pts',(-190.499797482064,55.2999999999999,102.335336081498));
#87832=CARTESIAN_POINT('Ctrl Pts',(-190.486691892323,55.3,105.902049807941));
#87833=CARTESIAN_POINT('Ctrl Pts',(-190.462485288409,55.2999999999994,109.468349270102));
#87834=CARTESIAN_POINT('Ctrl Pts',(-190.4120617449,55.2999999999994,113.033670360094));
#87835=CARTESIAN_POINT('Ctrl Pts',(-190.386326129341,55.2999999999994,114.853370574095));
#87836=CARTESIAN_POINT('Ctrl Pts',(-190.353761766739,55.2999999999996,116.6728159339));
#87837=CARTESIAN_POINT('Ctrl Pts',(-190.312364415728,55.2999999999999,118.491931513318));
#87838=CARTESIAN_POINT('Ctrl Pts',(-190.26239910735,55.3000000000004,120.687547142897));
#87839=CARTESIAN_POINT('Ctrl Pts',(-190.199254190876,55.2999999999999,122.882671101962));
#87840=CARTESIAN_POINT('Ctrl Pts',(-190.116985654538,55.2999999999998,125.077081385043));
#87841=CARTESIAN_POINT('Ctrl Pts',(-190.098341748212,55.2999999999998,125.574384261422));
#87842=CARTESIAN_POINT('Ctrl Pts',(-190.078715787918,55.2999999999998,126.071650491612));
#87843=CARTESIAN_POINT('Ctrl Pts',(-190.058038765853,55.2999999999997,126.568877497678));
#87844=CARTESIAN_POINT('Ctrl Pts',(-190.005527764093,55.2999999999996,127.831626461638));
#87845=CARTESIAN_POINT('Ctrl Pts',(-189.946274541593,55.3000000000004,129.094132890502));
#87846=CARTESIAN_POINT('Ctrl Pts',(-189.878604951289,55.2999999999989,130.356321825266));
#87847=CARTESIAN_POINT('Ctrl Pts',(-189.801961025494,55.2999999999971,131.785902152592));
#87848=CARTESIAN_POINT('Ctrl Pts',(-189.714520017616,55.2999999999926,133.215074811835));
#87849=CARTESIAN_POINT('Ctrl Pts',(-189.613859593324,55.2999999999818,134.643729735402));
#87850=CARTESIAN_POINT('Ctrl Pts',(-189.567223188341,55.2999999999768,135.30563167021));
#87851=CARTESIAN_POINT('Ctrl Pts',(-189.51774671133,55.2999999999746,135.967606041755));
#87852=CARTESIAN_POINT('Ctrl Pts',(-189.465075917415,55.2999999999738,136.629493724172));
#87853=CARTESIAN_POINT('Ctrl Pts',(-189.329240119307,55.2999999999716,138.336474669696));
#87854=CARTESIAN_POINT('Ctrl Pts',(-189.172155668906,55.2999999999801,140.042873666388));
#87855=CARTESIAN_POINT('Ctrl Pts',(-188.987779803917,55.2999999999871,141.745933189677));
#87856=CARTESIAN_POINT('Ctrl Pts',(-188.952829258419,55.2999999999884,142.068767522461));
#87857=CARTESIAN_POINT('Ctrl Pts',(-188.916898181551,55.2999999999897,142.391481893429));
#87858=CARTESIAN_POINT('Ctrl Pts',(-188.879945626183,55.2999999999908,142.714057575824));
#87859=CARTESIAN_POINT('Ctrl Pts',(-188.750614226618,55.2999999999948,143.843050254512));
#87860=CARTESIAN_POINT('Ctrl Pts',(-188.608928166082,55.2999999999971,144.969702294663));
#87861=CARTESIAN_POINT('Ctrl Pts',(-188.452204690944,55.2999999999979,146.093506559918));
#87862=CARTESIAN_POINT('Ctrl Pts',(-188.257218139742,55.299999999999,147.491680749931));
#87863=CARTESIAN_POINT('Ctrl Pts',(-188.038953458898,55.2999999999974,148.885446027331));
#87864=CARTESIAN_POINT('Ctrl Pts',(-187.792286254426,55.2999999999928,150.273830439671));
#87865=CARTESIAN_POINT('Ctrl Pts',(-187.765197067702,55.2999999999923,150.426303909631));
#87866=CARTESIAN_POINT('Ctrl Pts',(-187.737765380842,55.2999999999918,150.578712491456));
#87867=CARTESIAN_POINT('Ctrl Pts',(-187.709984445717,55.2999999999912,150.731054904143));
#87868=CARTESIAN_POINT('Ctrl Pts',(-187.493624536488,55.2999999999867,151.917508507399));
#87869=CARTESIAN_POINT('Ctrl Pts',(-187.256237229441,55.2999999999887,153.099979686043));
#87870=CARTESIAN_POINT('Ctrl Pts',(-186.992719010159,55.2999999999906,154.277501006747));
#87871=CARTESIAN_POINT('Ctrl Pts',(-186.740879122074,55.2999999999925,155.402838140671));
#87872=CARTESIAN_POINT('Ctrl Pts',(-186.465172879604,55.2999999999945,156.523654431007));
#87873=CARTESIAN_POINT('Ctrl Pts',(-186.161192902748,55.2999999999918,157.639113379179));
#87874=CARTESIAN_POINT('Ctrl Pts',(-186.070081234826,55.2999999999909,157.973448970351));
#87875=CARTESIAN_POINT('Ctrl Pts',(-185.976429868101,55.2999999999897,158.307303327867));
#87876=CARTESIAN_POINT('Ctrl Pts',(-185.88012104457,55.2999999999879,158.640654079262));
#87877=CARTESIAN_POINT('Ctrl Pts',(-185.612786098818,55.2999999999829,159.56597225648));
#87878=CARTESIAN_POINT('Ctrl Pts',(-185.324526062901,55.2999999999913,160.487428138369));
#87879=CARTESIAN_POINT('Ctrl Pts',(-185.014202918841,55.2999999999948,161.398696211986));
#87880=CARTESIAN_POINT('Ctrl Pts',(-184.886035202094,55.2999999999962,161.775062430795));
#87881=CARTESIAN_POINT('Ctrl Pts',(-184.75410415523,55.2999999999968,162.149691352719));
#87882=CARTESIAN_POINT('Ctrl Pts',(-184.618330478778,55.2999999999954,162.522139724443));
#87883=CARTESIAN_POINT('Ctrl Pts',(-184.23064261954,55.2999999999914,163.585627991711));
#87884=CARTESIAN_POINT('Ctrl Pts',(-183.810946185528,55.2999999999973,164.633847666811));
#87885=CARTESIAN_POINT('Ctrl Pts',(-183.354597012639,55.2999999999993,165.664583381619));
#87886=CARTESIAN_POINT('Ctrl Pts',(-183.263221822042,55.2999999999997,165.870968487565));
#87887=CARTESIAN_POINT('Ctrl Pts',(-183.170377275705,55.3,166.076652697458));
#87888=CARTESIAN_POINT('Ctrl Pts',(-183.076026323033,55.2999999999999,166.281618301401));
#87889=CARTESIAN_POINT('Ctrl Pts',(-182.580805460325,55.2999999999997,167.35742347703));
#87890=CARTESIAN_POINT('Ctrl Pts',(-182.044068007193,55.2999999999999,168.413424777875));
#87891=CARTESIAN_POINT('Ctrl Pts',(-181.45994811726,55.2999999999962,169.446823583728));
#87892=CARTESIAN_POINT('Ctrl Pts',(-181.375812919564,55.2999999999957,169.59567181562));
#87893=CARTESIAN_POINT('Ctrl Pts',(-181.290694734727,55.2999999999953,169.744051101896));
#87894=CARTESIAN_POINT('Ctrl Pts',(-181.204575998837,55.2999999999944,169.891953198675));
#87895=CARTESIAN_POINT('Ctrl Pts',(-180.915435634367,55.2999999999914,170.3885288361));
#87896=CARTESIAN_POINT('Ctrl Pts',(-180.615009421971,55.2999999999974,170.879720750648));
#87897=CARTESIAN_POINT('Ctrl Pts',(-180.302607188989,55.2999999999992,171.365199942073));
#87898=CARTESIAN_POINT('Ctrl Pts',(-180.245054999167,55.2999999999995,171.454637172764));
#87899=CARTESIAN_POINT('Ctrl Pts',(-180.187096430933,55.2999999999997,171.543880399659));
#87900=CARTESIAN_POINT('Ctrl Pts',(-180.128726879727,55.2999999999996,171.632927989696));
#87901=CARTESIAN_POINT('Ctrl Pts',(-179.894241861513,55.2999999999995,171.990654327147));
#87902=CARTESIAN_POINT('Ctrl Pts',(-179.652545955628,55.2999999999997,172.345968524669));
#87903=CARTESIAN_POINT('Ctrl Pts',(-179.404876266101,55.2999999999998,172.696746542243));
#87904=CARTESIAN_POINT('Ctrl Pts',(-179.255994389225,55.2999999999999,172.907610010127));
#87905=CARTESIAN_POINT('Ctrl Pts',(-179.104954749709,55.3,173.116833074002));
#87906=CARTESIAN_POINT('Ctrl Pts',(-178.952022467963,55.3,173.323959339789));
#87907=CARTESIAN_POINT('Ctrl Pts',(-178.41719983759,55.3,174.048304867251));
#87908=CARTESIAN_POINT('Ctrl Pts',(-177.858788574558,55.3,174.747631024544));
#87909=CARTESIAN_POINT('Ctrl Pts',(-177.277237712592,55.3,175.422402984304));
#87910=CARTESIAN_POINT('Ctrl Pts',(-176.681725802524,55.3,176.113373912038));
#87911=CARTESIAN_POINT('Ctrl Pts',(-176.061949956807,55.3,176.778597639781));
#87912=CARTESIAN_POINT('Ctrl Pts',(-175.418353704452,55.3,177.41853304461));
#87913=CARTESIAN_POINT('Ctrl Pts',(-174.774757452097,55.3,178.05846844944));
#87914=CARTESIAN_POINT('Ctrl Pts',(-174.107341075041,55.3000000000009,178.673115079697));
#87915=CARTESIAN_POINT('Ctrl Pts',(-173.416509908913,55.2999999999999,179.26289316856));
#87916=CARTESIAN_POINT('Ctrl Pts',(-172.902930290524,55.2999999999991,179.70134762844));
#87917=CARTESIAN_POINT('Ctrl Pts',(-172.376508960269,55.2999999999991,180.126166505602));
#87918=CARTESIAN_POINT('Ctrl Pts',(-171.837640512919,55.2999999999989,180.537771132798));
#87919=CARTESIAN_POINT('Ctrl Pts',(-171.568206289244,55.2999999999988,180.743573446396));
#87920=CARTESIAN_POINT('Ctrl Pts',(-171.295660191796,55.2999999999986,180.946072091014));
#87921=CARTESIAN_POINT('Ctrl Pts',(-171.020051006383,55.2999999999983,181.145319119996));
#87922=CARTESIAN_POINT('Ctrl Pts',(-170.876736551081,55.2999999999981,181.248925897057));
#87923=CARTESIAN_POINT('Ctrl Pts',(-170.732593857952,55.2999999999978,181.351653459219));
#87924=CARTESIAN_POINT('Ctrl Pts',(-170.587629750578,55.2999999999975,181.453509083908));
#87925=CARTESIAN_POINT('Ctrl Pts',(-170.453812213327,55.2999999999972,181.547532832943));
#87926=CARTESIAN_POINT('Ctrl Pts',(-170.319291857913,55.2999999999971,181.640815489386));
#87927=CARTESIAN_POINT('Ctrl Pts',(-170.184091336249,55.2999999999959,181.733351070885));
#87928=CARTESIAN_POINT('Ctrl Pts',(-169.902739839192,55.2999999999936,181.925917076294));
#87929=CARTESIAN_POINT('Ctrl Pts',(-169.618005644094,55.2999999999945,182.115519126605));
#87930=CARTESIAN_POINT('Ctrl Pts',(-169.330645353429,55.299999999996,182.301804073465));
#87931=CARTESIAN_POINT('Ctrl Pts',(-169.186572407503,55.2999999999967,182.395201184853));
#87932=CARTESIAN_POINT('Ctrl Pts',(-169.041839246008,55.2999999999975,182.487764336891));
#87933=CARTESIAN_POINT('Ctrl Pts',(-168.89654087646,55.2999999999981,182.579448043434));
#87934=CARTESIAN_POINT('Ctrl Pts',(-168.834229760776,55.2999999999984,182.618766544133));
#87935=CARTESIAN_POINT('Ctrl Pts',(-168.771814695492,55.2999999999986,182.657923295422));
#87936=CARTESIAN_POINT('Ctrl Pts',(-168.709303172194,55.2999999999988,182.696914667427));
#87937=CARTESIAN_POINT('Ctrl Pts',(-168.650733708525,55.2999999999989,182.733447191761));
#87938=CARTESIAN_POINT('Ctrl Pts',(-168.59208268385,55.299999999999,182.76983257515));
#87939=CARTESIAN_POINT('Ctrl Pts',(-168.533364737283,55.299999999999,182.806062700292));
#87940=CARTESIAN_POINT('Ctrl Pts',(-168.509414306756,55.299999999999,182.82084058586));
#87941=CARTESIAN_POINT('Ctrl Pts',(-168.485452338166,55.299999999999,182.835592892692));
#87942=CARTESIAN_POINT('Ctrl Pts',(-168.46147926487,55.299999999999,182.850319418911));
#87943=CARTESIAN_POINT('Ctrl Pts',(-168.169963101635,55.2999999999989,183.029396184255));
#87944=CARTESIAN_POINT('Ctrl Pts',(-167.876944721106,55.2999999999992,183.204614901524));
#87945=CARTESIAN_POINT('Ctrl Pts',(-167.582420661782,55.2999999999995,183.376193981152));
#87946=CARTESIAN_POINT('Ctrl Pts',(-167.384297559265,55.2999999999997,183.491613345061));
#87947=CARTESIAN_POINT('Ctrl Pts',(-167.185493054643,55.2999999999999,183.605385566813));
#87948=CARTESIAN_POINT('Ctrl Pts',(-166.986005355678,55.3,183.717575256982));
#87949=CARTESIAN_POINT('Ctrl Pts',(-166.888940425809,55.3,183.772163507109));
#87950=CARTESIAN_POINT('Ctrl Pts',(-166.791714965253,55.3,183.826376357779));
#87951=CARTESIAN_POINT('Ctrl Pts',(-166.694335930232,55.3,183.880217249607));
#87952=CARTESIAN_POINT('Ctrl Pts',(-165.743362040703,55.3,184.40601094131));
#87953=CARTESIAN_POINT('Ctrl Pts',(-164.777788310111,55.3,184.896759395401));
#87954=CARTESIAN_POINT('Ctrl Pts',(-163.799410499353,55.3,185.356773166156));
#87955=CARTESIAN_POINT('Ctrl Pts',(-162.812239834025,55.3,185.820921162096));
#87956=CARTESIAN_POINT('Ctrl Pts',(-161.812033992515,55.2999999999999,186.253779761824));
#87957=CARTESIAN_POINT('Ctrl Pts',(-160.800656964796,55.2999999999999,186.659825139884));
#87958=CARTESIAN_POINT('Ctrl Pts',(-160.31097753273,55.2999999999999,186.856420538704));
#87959=CARTESIAN_POINT('Ctrl Pts',(-159.818679305665,55.3000000000012,187.046731154551));
#87960=CARTESIAN_POINT('Ctrl Pts',(-159.323976398265,55.2999999999994,187.231268441749));
#87961=CARTESIAN_POINT('Ctrl Pts',(-158.693118416369,55.299999999997,187.466595177949));
#87962=CARTESIAN_POINT('Ctrl Pts',(-158.058297774248,55.2999999999972,187.692418003419));
#87963=CARTESIAN_POINT('Ctrl Pts',(-157.419838084174,55.2999999999965,187.909507127552));
#87964=CARTESIAN_POINT('Ctrl Pts',(-157.019499284202,55.2999999999961,188.045630364137));
#87965=CARTESIAN_POINT('Ctrl Pts',(-156.617729738341,55.2999999999953,188.178319823437));
#87966=CARTESIAN_POINT('Ctrl Pts',(-156.214609655659,55.2999999999934,188.307766485117));
#87967=CARTESIAN_POINT('Ctrl Pts',(-155.974834462964,55.2999999999922,188.384761156387));
#87968=CARTESIAN_POINT('Ctrl Pts',(-155.734577656072,55.2999999999914,188.460609746169));
#87969=CARTESIAN_POINT('Ctrl Pts',(-155.493876194086,55.299999999987,188.535346445525));
#87970=CARTESIAN_POINT('Ctrl Pts',(-154.849286915679,55.2999999999753,188.735488458418));
#87971=CARTESIAN_POINT('Ctrl Pts',(-154.200851882109,55.2999999999802,188.927821054047));
#87972=CARTESIAN_POINT('Ctrl Pts',(-153.549758382643,55.2999999999871,189.112746132645));
#87973=CARTESIAN_POINT('Ctrl Pts',(-153.22421163291,55.2999999999906,189.205208671944));
#87974=CARTESIAN_POINT('Ctrl Pts',(-152.898000237317,55.2999999999945,189.295819123002));
#87975=CARTESIAN_POINT('Ctrl Pts',(-152.571272698333,55.2999999999971,189.384626541979));
#87976=CARTESIAN_POINT('Ctrl Pts',(-152.406379380498,55.2999999999984,189.429445996161));
#87977=CARTESIAN_POINT('Ctrl Pts',(-152.241354602361,55.2999999999993,189.473806200192));
#87978=CARTESIAN_POINT('Ctrl Pts',(-152.076217481013,55.2999999999997,189.517713389758));
#87979=CARTESIAN_POINT('Ctrl Pts',(-151.943218512572,55.3,189.553075583744));
#87980=CARTESIAN_POINT('Ctrl Pts',(-151.810145280887,55.2999999999999,189.588144270557));
#87981=CARTESIAN_POINT('Ctrl Pts',(-151.677027873674,55.2999999999993,189.622917512509));
#87982=CARTESIAN_POINT('Ctrl Pts',(-151.647927448919,55.2999999999991,189.630519193853));
#87983=CARTESIAN_POINT('Ctrl Pts',(-151.618824705037,55.2999999999989,189.638106811891));
#87984=CARTESIAN_POINT('Ctrl Pts',(-151.58971975818,55.2999999999988,189.645680399349));
#87985=CARTESIAN_POINT('Ctrl Pts',(-150.2812980681,55.29999999999,189.98615331447));
#87986=CARTESIAN_POINT('Ctrl Pts',(-148.970507516151,55.2999999999809,190.298209232362));
#87987=CARTESIAN_POINT('Ctrl Pts',(-147.657489395253,55.2999999999767,190.586549148109));
#87988=CARTESIAN_POINT('Ctrl Pts',(-147.000980334804,55.2999999999746,190.730719105983));
#87989=CARTESIAN_POINT('Ctrl Pts',(-146.34391436091,55.2999999999738,190.868959783947));
#87990=CARTESIAN_POINT('Ctrl Pts',(-145.686309051212,55.2999999999748,191.00185772528));
#87991=CARTESIAN_POINT('Ctrl Pts',(-145.236865028949,55.2999999999755,191.092687565646));
#87992=CARTESIAN_POINT('Ctrl Pts',(-144.787169075752,55.2999999999771,191.181021739963));
#87993=CARTESIAN_POINT('Ctrl Pts',(-144.33722679863,55.2999999999798,191.267047451344));
#87994=CARTESIAN_POINT('Ctrl Pts',(-144.128834743028,55.299999999981,191.3068905062));
#87995=CARTESIAN_POINT('Ctrl Pts',(-143.920388717415,55.2999999999825,191.346238574216));
#87996=CARTESIAN_POINT('Ctrl Pts',(-143.711897764384,55.2999999999843,191.385108697693));
#87997=CARTESIAN_POINT('Ctrl Pts',(-141.950706217328,55.3000000000001,191.71345739535));
#87998=CARTESIAN_POINT('Ctrl Pts',(-140.186182407371,55.3000000000011,192.007447721363));
#87999=CARTESIAN_POINT('Ctrl Pts',(-138.418979168621,55.2999999999956,192.273910691535));
#88000=CARTESIAN_POINT('Ctrl Pts',(-137.546066740989,55.2999999999928,192.405530435697));
#88001=CARTESIAN_POINT('Ctrl Pts',(-136.672500176854,55.2999999999896,192.530434732744));
#88002=CARTESIAN_POINT('Ctrl Pts',(-135.79835995011,55.2999999999832,192.64945104723));
#88003=CARTESIAN_POINT('Ctrl Pts',(-133.742775638351,55.2999999999681,192.929323842712));
#88004=CARTESIAN_POINT('Ctrl Pts',(-131.684009902325,55.2999999999751,193.176457453746));
#88005=CARTESIAN_POINT('Ctrl Pts',(-129.622742521771,55.2999999999818,193.397881768966));
#88006=CARTESIAN_POINT('Ctrl Pts',(-129.035163425207,55.2999999999837,193.461000363051));
#88007=CARTESIAN_POINT('Ctrl Pts',(-128.447380807758,55.2999999999854,193.522030170679));
#88008=CARTESIAN_POINT('Ctrl Pts',(-127.859411366078,55.2999999999871,193.581134526229));
#88009=CARTESIAN_POINT('Ctrl Pts',(-125.144150681436,55.2999999999946,193.854080229763));
#88010=CARTESIAN_POINT('Ctrl Pts',(-122.424955472583,55.2999999999977,194.086609801097));
#88011=CARTESIAN_POINT('Ctrl Pts',(-119.702735665975,55.2999999999966,194.288037001772));
#88012=CARTESIAN_POINT('Ctrl Pts',(-117.522588010382,55.2999999999957,194.449354261406));
#88013=CARTESIAN_POINT('Ctrl Pts',(-115.340500490943,55.2999999999921,194.590723897809));
#88014=CARTESIAN_POINT('Ctrl Pts',(-113.156942060905,55.299999999986,194.716950287514));
#88015=CARTESIAN_POINT('Ctrl Pts',(-112.748096052287,55.2999999999848,194.740584716025));
#88016=CARTESIAN_POINT('Ctrl Pts',(-112.339198609107,55.2999999999837,194.763688283965));
#88017=CARTESIAN_POINT('Ctrl Pts',(-111.930252346801,55.2999999999822,194.786292608757));
#88018=CARTESIAN_POINT('Ctrl Pts',(-107.974707073947,55.2999999999682,195.004933634036));
#88019=CARTESIAN_POINT('Ctrl Pts',(-104.014517429673,55.2999999999849,195.175894152784));
#88020=CARTESIAN_POINT('Ctrl Pts',(-100.051160906159,55.2999999999941,195.314262519372));
#88021=CARTESIAN_POINT('Ctrl Pts',(-98.6870868231336,55.2999999999972,195.361884957993));
#88022=CARTESIAN_POINT('Ctrl Pts',(-97.3226375965247,55.2999999999995,195.405647209011));
#88023=CARTESIAN_POINT('Ctrl Pts',(-95.9578737332236,55.2999999999994,195.446165741684));
#88024=CARTESIAN_POINT('Ctrl Pts',(-93.2937797771208,55.2999999999991,195.525260141021));
#88025=CARTESIAN_POINT('Ctrl Pts',(-90.6283351791982,55.2999999999899,195.591817563438));
#88026=CARTESIAN_POINT('Ctrl Pts',(-87.9622980004871,55.2999999999833,195.648477101291));
#88027=CARTESIAN_POINT('Ctrl Pts',(-86.4341087402463,55.2999999999795,195.680954704353));
#88028=CARTESIAN_POINT('Ctrl Pts',(-84.9057247909427,55.2999999999766,195.710180235644));
#88029=CARTESIAN_POINT('Ctrl Pts',(-83.3772890352257,55.2999999999766,195.736651020953));
#88030=CARTESIAN_POINT('Ctrl Pts',(-82.3556648250435,55.2999999999767,195.754344401283));
#88031=CARTESIAN_POINT('Ctrl Pts',(-81.3340174708388,55.299999999978,195.770807037021));
#88032=CARTESIAN_POINT('Ctrl Pts',(-80.3123896643528,55.2999999999814,195.786187504847));
#88033=CARTESIAN_POINT('Ctrl Pts',(-80.1959820125014,55.2999999999818,195.787940006231));
#88034=CARTESIAN_POINT('Ctrl Pts',(-80.0795746244709,55.2999999999822,195.789678457632));
#88035=CARTESIAN_POINT('Ctrl Pts',(-79.9631677685342,55.2999999999827,195.791403075907));
#88036=CARTESIAN_POINT('Ctrl Pts',(-76.1297427206355,55.2999999999984,195.848196937737));
#88037=CARTESIAN_POINT('Ctrl Pts',(-72.2961721091227,55.3000000000004,195.889842603839));
#88038=CARTESIAN_POINT('Ctrl Pts',(-68.4625314791343,55.3000000000001,195.921169797769));
#88039=CARTESIAN_POINT('Ctrl Pts',(-66.964441063854,55.3,195.933411677876));
#88040=CARTESIAN_POINT('Ctrl Pts',(-65.4663401615409,55.2999999999993,195.944077956465));
#88041=CARTESIAN_POINT('Ctrl Pts',(-63.9682326441714,55.2999999999994,195.953457116585));
#88042=CARTESIAN_POINT('Ctrl Pts',(-58.6374128389523,55.2999999999997,195.986831632062));
#88043=CARTESIAN_POINT('Ctrl Pts',(-53.3064763293846,55.2999999999998,196.004466674216));
#88044=CARTESIAN_POINT('Ctrl Pts',(-47.9754976701425,55.2999999999999,196.01317970203));
#88045=CARTESIAN_POINT('Ctrl Pts',(-44.2886966671822,55.2999999999999,196.019205462352));
#88046=CARTESIAN_POINT('Ctrl Pts',(-40.6018755026786,55.3,196.020964151304));
#88047=CARTESIAN_POINT('Ctrl Pts',(-36.915058817711,55.3,196.020712339862));
#88048=CARTESIAN_POINT('Ctrl Pts',(-35.2708741678306,55.3,196.020600041219));
#88049=CARTESIAN_POINT('Ctrl Pts',(-33.6266905523897,55.2999999999999,196.020087900419));
#88050=CARTESIAN_POINT('Ctrl Pts',(-31.9825097205406,55.2999999999999,196.019376110131));
#88051=CARTESIAN_POINT('Ctrl Pts',(-21.3216725475468,55.2999999999999,196.014760875474));
#88052=CARTESIAN_POINT('Ctrl Pts',(-10.6608381121449,55.3,196.));
#88053=CARTESIAN_POINT('Ctrl Pts',(1.06581410364015E-14,55.3,196.));
#88054=CARTESIAN_POINT('Origin',(160.5,51.6013867006572,102.225104347672));
#88055=CARTESIAN_POINT('',(190.5,58.3,102.225104347672));
#88056=CARTESIAN_POINT('',(190.5,55.3,102.225104347672));
#88057=CARTESIAN_POINT('',(190.5,51.6013867006572,102.225104347672));
#88058=CARTESIAN_POINT('',(190.499797482064,58.3,102.335336081499));
#88059=CARTESIAN_POINT('Origin',(160.5,58.3,102.225104347672));
#88060=CARTESIAN_POINT('',(190.499797482064,55.3,102.335336081499));
#88061=CARTESIAN_POINT('',(190.499797482064,51.6013867006573,102.335336081499));
#88062=CARTESIAN_POINT('Origin',(160.5,55.3,102.225104347672));
#88063=CARTESIAN_POINT('Ctrl Pts',(1.20290037631083E-14,55.2999999999999,
196.));
#88064=CARTESIAN_POINT('Ctrl Pts',(1.15700533001727E-14,58.9,196.));
#88065=CARTESIAN_POINT('Ctrl Pts',(180.96963113231,55.3,196.));
#88066=CARTESIAN_POINT('Ctrl Pts',(180.96963113231,58.9,196.));
#88067=CARTESIAN_POINT('Ctrl Pts',(190.141509581597,55.3,199.844139409912));
#88068=CARTESIAN_POINT('Ctrl Pts',(190.141509581597,58.9,199.844139409912));
#88069=CARTESIAN_POINT('Ctrl Pts',(190.499797482064,55.3,102.335336081499));
#88070=CARTESIAN_POINT('Ctrl Pts',(190.499797482064,58.9,102.335336081499));
#88071=CARTESIAN_POINT('Ctrl Pts',(190.499797482064,58.3,102.335336081499));
#88072=CARTESIAN_POINT('Ctrl Pts',(190.486691892692,58.3,105.902049707337));
#88073=CARTESIAN_POINT('Ctrl Pts',(190.462485289776,58.3,109.468349068915));
#88074=CARTESIAN_POINT('Ctrl Pts',(190.412061749167,58.3,113.033670058396));
#88075=CARTESIAN_POINT('Ctrl Pts',(190.386326132941,58.3,114.853370372991));
#88076=CARTESIAN_POINT('Ctrl Pts',(190.353761769027,58.3,116.672815833366));
#88077=CARTESIAN_POINT('Ctrl Pts',(190.312364415728,58.3,118.491931513319));
#88078=CARTESIAN_POINT('Ctrl Pts',(190.262398908667,58.3,120.687555873587));
#88079=CARTESIAN_POINT('Ctrl Pts',(190.19925368868,58.3,122.882688559424));
#88080=CARTESIAN_POINT('Ctrl Pts',(190.116984673134,58.3,125.077107562727));
#88081=CARTESIAN_POINT('Ctrl Pts',(190.098341059481,58.3,125.574401711925));
#88082=CARTESIAN_POINT('Ctrl Pts',(190.07871542511,58.3,126.071659216176));
#88083=CARTESIAN_POINT('Ctrl Pts',(190.058038765853,58.3,126.568877497679));
#88084=CARTESIAN_POINT('Ctrl Pts',(190.005527904509,58.3,127.831623085003));
#88085=CARTESIAN_POINT('Ctrl Pts',(189.946274858486,58.3000000000002,129.094126138524));
#88086=CARTESIAN_POINT('Ctrl Pts',(189.878605494142,58.3000000000003,130.356311699848));
#88087=CARTESIAN_POINT('Ctrl Pts',(189.801961438374,58.3000000000005,131.785895404238));
#88088=CARTESIAN_POINT('Ctrl Pts',(189.714520255269,58.3000000000007,133.215071438881));
#88089=CARTESIAN_POINT('Ctrl Pts',(189.613859593324,58.3000000000004,134.643729735403));
#88090=CARTESIAN_POINT('Ctrl Pts',(189.567223198167,58.3000000000003,135.305631530741));
#88091=CARTESIAN_POINT('Ctrl Pts',(189.51774673218,58.3000000000036,135.967605762786));
#88092=CARTESIAN_POINT('Ctrl Pts',(189.46507595071,58.3000000000082,136.629493305773));
#88093=CARTESIAN_POINT('Ctrl Pts',(189.329240157618,58.3000000000201,138.336474231981));
#88094=CARTESIAN_POINT('Ctrl Pts',(189.172155713213,58.3000000000407,140.042873209594));
#88095=CARTESIAN_POINT('Ctrl Pts',(188.9877798554,58.3000000000341,141.745932714139));
#88096=CARTESIAN_POINT('Ctrl Pts',(188.952829293703,58.3000000000328,142.068767205554));
#88097=CARTESIAN_POINT('Ctrl Pts',(188.916898199695,58.3000000000306,142.391481735044));
#88098=CARTESIAN_POINT('Ctrl Pts',(188.879945626183,58.3000000000271,142.714057575825));
#88099=CARTESIAN_POINT('Ctrl Pts',(188.750614304397,58.3000000000151,143.843049575544));
#88100=CARTESIAN_POINT('Ctrl Pts',(188.608928336502,58.3000000000094,144.969700939541));
#88101=CARTESIAN_POINT('Ctrl Pts',(188.452204973701,58.3000000000058,146.093504532372));
#88102=CARTESIAN_POINT('Ctrl Pts',(188.25721844303,58.3000000000012,147.491678740773));
#88103=CARTESIAN_POINT('Ctrl Pts',(188.038953784735,58.3000000000009,148.885444036944));
#88104=CARTESIAN_POINT('Ctrl Pts',(187.792286604651,58.3000000000004,150.273828468404));
#88105=CARTESIAN_POINT('Ctrl Pts',(187.765197304137,58.3000000000004,150.426302596012));
#88106=CARTESIAN_POINT('Ctrl Pts',(187.737765500565,58.3000000000003,150.578711834932));
#88107=CARTESIAN_POINT('Ctrl Pts',(187.709984445717,58.3000000000003,150.731054904144));
#88108=CARTESIAN_POINT('Ctrl Pts',(187.493624541263,58.2999999999998,151.917508481214));
#88109=CARTESIAN_POINT('Ctrl Pts',(187.256237239919,58.3000000000075,153.09997963385));
#88110=CARTESIAN_POINT('Ctrl Pts',(186.992719027606,58.3000000000135,154.277500928785));
#88111=CARTESIAN_POINT('Ctrl Pts',(186.740879139795,58.3000000000192,155.402838066619));
#88112=CARTESIAN_POINT('Ctrl Pts',(186.465172897544,58.3000000000235,156.523654360854));
#88113=CARTESIAN_POINT('Ctrl Pts',(186.161192920807,58.3000000000189,157.639113312908));
#88114=CARTESIAN_POINT('Ctrl Pts',(186.070081247201,58.3000000000175,157.973448926234));
#88115=CARTESIAN_POINT('Ctrl Pts',(185.976429874464,58.3000000000152,158.307303305843));
#88116=CARTESIAN_POINT('Ctrl Pts',(185.880121044569,58.300000000012,158.640654079262));
#88117=CARTESIAN_POINT('Ctrl Pts',(185.61278602088,58.300000000003,159.565972526244));
#88118=CARTESIAN_POINT('Ctrl Pts',(185.324525894825,58.3000000000103,160.487428675641));
#88119=CARTESIAN_POINT('Ctrl Pts',(185.014202647431,58.3000000000117,161.398697008986));
#88120=CARTESIAN_POINT('Ctrl Pts',(184.886035015842,58.3000000000123,161.775062959677));
#88121=CARTESIAN_POINT('Ctrl Pts',(184.754104059391,58.3000000000119,162.14969161562));
#88122=CARTESIAN_POINT('Ctrl Pts',(184.618330478778,58.3000000000092,162.522139724444));
#88123=CARTESIAN_POINT('Ctrl Pts',(184.230642847717,58.3000000000013,163.585627365785));
#88124=CARTESIAN_POINT('Ctrl Pts',(183.810946679566,58.3000000000002,164.633846432934));
#88125=CARTESIAN_POINT('Ctrl Pts',(183.354597818405,58.3000000000001,165.66458156167));
#88126=CARTESIAN_POINT('Ctrl Pts',(183.263222367858,58.3000000000001,165.870967278386));
#88127=CARTESIAN_POINT('Ctrl Pts',(183.17037755304,58.3000000000001,166.076652094981));
#88128=CARTESIAN_POINT('Ctrl Pts',(183.076026323032,58.3000000000001,166.281618301402));
#88129=CARTESIAN_POINT('Ctrl Pts',(182.580804157945,58.3000000000003,167.357426306289));
#88130=CARTESIAN_POINT('Ctrl Pts',(182.044065184055,58.3000000000001,168.413430332222));
#88131=CARTESIAN_POINT('Ctrl Pts',(181.459943508732,58.3000000000056,169.446831736928));
#88132=CARTESIAN_POINT('Ctrl Pts',(181.375809811316,58.3000000000064,169.595677233963));
#88133=CARTESIAN_POINT('Ctrl Pts',(181.290693162334,58.300000000007,169.744053802355));
#88134=CARTESIAN_POINT('Ctrl Pts',(181.204575998837,58.3000000000083,169.891953198676));
#88135=CARTESIAN_POINT('Ctrl Pts',(180.915435742078,58.3000000000128,170.388528651114));
#88136=CARTESIAN_POINT('Ctrl Pts',(180.6150096458,58.3000000000038,170.879720384691));
#88137=CARTESIAN_POINT('Ctrl Pts',(180.302607538116,58.3000000000012,171.365199399522));
#88138=CARTESIAN_POINT('Ctrl Pts',(180.245055233562,58.3000000000007,171.454636811847));
#88139=CARTESIAN_POINT('Ctrl Pts',(180.187096548962,58.3000000000004,171.543880219597));
#88140=CARTESIAN_POINT('Ctrl Pts',(180.128726879727,58.3000000000005,171.632927989697));
#88141=CARTESIAN_POINT('Ctrl Pts',(179.894241878965,58.3000000000007,171.990654300523));
#88142=CARTESIAN_POINT('Ctrl Pts',(179.652545991606,58.3000000000004,172.345968471778));
#88143=CARTESIAN_POINT('Ctrl Pts',(179.404876321403,58.3000000000002,172.696746463919));
#88144=CARTESIAN_POINT('Ctrl Pts',(179.255994426627,58.3000000000001,172.907609958317));
#88145=CARTESIAN_POINT('Ctrl Pts',(179.104954768645,58.3,173.116833048357));
#88146=CARTESIAN_POINT('Ctrl Pts',(178.952022467963,58.3,173.323959339789));
#88147=CARTESIAN_POINT('Ctrl Pts',(178.417199844465,58.3,174.04830485794));
#88148=CARTESIAN_POINT('Ctrl Pts',(177.858788588915,58.3,174.747631006561));
#88149=CARTESIAN_POINT('Ctrl Pts',(177.277237735021,58.3,175.422402958276));
#88150=CARTESIAN_POINT('Ctrl Pts',(176.681725821823,58.3,176.113373890994));
#88151=CARTESIAN_POINT('Ctrl Pts',(176.061949972666,58.3,176.778597623392));
#88152=CARTESIAN_POINT('Ctrl Pts',(175.418353716571,58.3,177.418533032557));
#88153=CARTESIAN_POINT('Ctrl Pts',(174.774757460475,58.3,178.058468441722));
#88154=CARTESIAN_POINT('Ctrl Pts',(174.107341079373,58.3,178.673115075999));
#88155=CARTESIAN_POINT('Ctrl Pts',(173.416509908913,58.3,179.262893168561));
#88156=CARTESIAN_POINT('Ctrl Pts',(172.902930290527,58.3,179.701347628437));
#88157=CARTESIAN_POINT('Ctrl Pts',(172.376508960271,58.3,180.126166505599));
#88158=CARTESIAN_POINT('Ctrl Pts',(171.83764051292,58.3,180.537771132796));
#88159=CARTESIAN_POINT('Ctrl Pts',(171.568206289245,58.3,180.743573446395));
#88160=CARTESIAN_POINT('Ctrl Pts',(171.295660191797,58.3,180.946072091013));
#88161=CARTESIAN_POINT('Ctrl Pts',(171.020051006383,58.3,181.145319119995));
#88162=CARTESIAN_POINT('Ctrl Pts',(170.87673654841,58.3,181.248925898987));
#88163=CARTESIAN_POINT('Ctrl Pts',(170.73259385258,58.3,181.351653463048));
#88164=CARTESIAN_POINT('Ctrl Pts',(170.587629742474,58.3,181.453509089602));
#88165=CARTESIAN_POINT('Ctrl Pts',(170.453812207896,58.3,181.547532836709));
#88166=CARTESIAN_POINT('Ctrl Pts',(170.319291855183,58.3,181.640815491254));
#88167=CARTESIAN_POINT('Ctrl Pts',(170.184091336249,58.3,181.733351070886));
#88168=CARTESIAN_POINT('Ctrl Pts',(169.902739839191,58.3,181.925917076294));
#88169=CARTESIAN_POINT('Ctrl Pts',(169.618005644093,58.3,182.115519126606));
#88170=CARTESIAN_POINT('Ctrl Pts',(169.330645353427,58.3,182.301804073466));
#88171=CARTESIAN_POINT('Ctrl Pts',(169.186572409167,58.3,182.395201183774));
#88172=CARTESIAN_POINT('Ctrl Pts',(169.041839249353,58.3,182.487764334752));
#88173=CARTESIAN_POINT('Ctrl Pts',(168.896540881497,58.3,182.579448040255));
#88174=CARTESIAN_POINT('Ctrl Pts',(168.834229775528,58.3,182.618766534837));
#88175=CARTESIAN_POINT('Ctrl Pts',(168.771814719992,58.3,182.657923280058));
#88176=CARTESIAN_POINT('Ctrl Pts',(168.70930320647,58.3,182.696914646047));
#88177=CARTESIAN_POINT('Ctrl Pts',(168.65073375144,58.3,182.73344716507));
#88178=CARTESIAN_POINT('Ctrl Pts',(168.592082735421,58.3,182.769832543196));
#88179=CARTESIAN_POINT('Ctrl Pts',(168.53336479753,58.3,182.806062663119));
#88180=CARTESIAN_POINT('Ctrl Pts',(168.50941434694,58.3,182.820840561121));
#88181=CARTESIAN_POINT('Ctrl Pts',(168.485452358266,58.3,182.835592880344));
#88182=CARTESIAN_POINT('Ctrl Pts',(168.46147926487,58.3,182.850319418911));
#88183=CARTESIAN_POINT('Ctrl Pts',(168.16996310164,58.3,183.029396184252));
#88184=CARTESIAN_POINT('Ctrl Pts',(167.876944721109,58.3,183.204614901521));
#88185=CARTESIAN_POINT('Ctrl Pts',(167.582420661783,58.3,183.376193981151));
#88186=CARTESIAN_POINT('Ctrl Pts',(167.384297562419,58.3,183.491613343224));
#88187=CARTESIAN_POINT('Ctrl Pts',(167.185493060971,58.3,183.605385563191));
#88188=CARTESIAN_POINT('Ctrl Pts',(166.986005365204,58.3,183.717575251625));
#88189=CARTESIAN_POINT('Ctrl Pts',(166.88894043217,58.3,183.772163503562));
#88190=CARTESIAN_POINT('Ctrl Pts',(166.791714968437,58.3,183.826376356018));
#88191=CARTESIAN_POINT('Ctrl Pts',(166.694335930232,58.3,183.880217249608));
#88192=CARTESIAN_POINT('Ctrl Pts',(165.743362022725,58.3,184.40601095125));
#88193=CARTESIAN_POINT('Ctrl Pts',(164.77778827359,58.300000000006,184.896759413961));
#88194=CARTESIAN_POINT('Ctrl Pts',(163.799410443834,58.3000000000113,185.356773192257));
#88195=CARTESIAN_POINT('Ctrl Pts',(162.812239974668,58.3000000000167,185.820921094562));
#88196=CARTESIAN_POINT('Ctrl Pts',(161.812034334544,58.3000000000215,186.253779613209));
#88197=CARTESIAN_POINT('Ctrl Pts',(160.800657512328,58.3000000000187,186.65982492006));
#88198=CARTESIAN_POINT('Ctrl Pts',(160.310977899702,58.3000000000174,186.85642039684));
#88199=CARTESIAN_POINT('Ctrl Pts',(159.818679490042,58.3000000000149,187.046731085773));
#88200=CARTESIAN_POINT('Ctrl Pts',(159.323976398265,58.3000000000085,187.23126844175));
#88201=CARTESIAN_POINT('Ctrl Pts',(158.693118416376,58.3000000000002,187.466595177947));
#88202=CARTESIAN_POINT('Ctrl Pts',(158.058297774254,58.2999999999984,187.692418003417));
#88203=CARTESIAN_POINT('Ctrl Pts',(157.419838084178,58.2999999999987,187.90950712755));
#88204=CARTESIAN_POINT('Ctrl Pts',(157.019499271022,58.2999999999989,188.045630368619));
#88205=CARTESIAN_POINT('Ctrl Pts',(156.617729711881,58.2999999999999,188.178319832175));
#88206=CARTESIAN_POINT('Ctrl Pts',(156.214609615834,58.3000000000006,188.307766497905));
#88207=CARTESIAN_POINT('Ctrl Pts',(155.974834436361,58.300000000001,188.384761164785));
#88208=CARTESIAN_POINT('Ctrl Pts',(155.734577642747,58.3000000000014,188.460609750306));
#88209=CARTESIAN_POINT('Ctrl Pts',(155.493876194085,58.3000000000011,188.535346445525));
#88210=CARTESIAN_POINT('Ctrl Pts',(154.849286915676,58.3000000000005,188.735488458419));
#88211=CARTESIAN_POINT('Ctrl Pts',(154.200851882107,58.3000000000027,188.927821054048));
#88212=CARTESIAN_POINT('Ctrl Pts',(153.549758382642,58.3000000000043,189.112746132646));
#88213=CARTESIAN_POINT('Ctrl Pts',(153.22421163291,58.3000000000051,189.205208671945));
#88214=CARTESIAN_POINT('Ctrl Pts',(152.898000237318,58.3000000000059,189.295819123002));
#88215=CARTESIAN_POINT('Ctrl Pts',(152.571272698334,58.300000000006,189.384626541979));
#88216=CARTESIAN_POINT('Ctrl Pts',(152.40637937128,58.3000000000061,189.429445998667));
#88217=CARTESIAN_POINT('Ctrl Pts',(152.241354583909,58.3000000000061,189.473806205152));
#88218=CARTESIAN_POINT('Ctrl Pts',(152.076217453316,58.3000000000058,189.517713397122));
#88219=CARTESIAN_POINT('Ctrl Pts',(151.943218487967,58.3000000000057,189.553075590242));
#88220=CARTESIAN_POINT('Ctrl Pts',(151.810145259381,58.3000000000053,189.588144276204));
#88221=CARTESIAN_POINT('Ctrl Pts',(151.677027855266,58.3000000000049,189.622917517318));
#88222=CARTESIAN_POINT('Ctrl Pts',(151.647927436647,58.3000000000048,189.630519197052));
#88223=CARTESIAN_POINT('Ctrl Pts',(151.6188246989,58.3000000000047,189.638106813488));
#88224=CARTESIAN_POINT('Ctrl Pts',(151.58971975818,58.3000000000046,189.645680399349));
#88225=CARTESIAN_POINT('Ctrl Pts',(150.281298068072,58.2999999999996,189.986153314478));
#88226=CARTESIAN_POINT('Ctrl Pts',(148.970507516125,58.2999999999987,190.29820923237));
#88227=CARTESIAN_POINT('Ctrl Pts',(147.657489395235,58.3000000000009,190.586549148116));
#88228=CARTESIAN_POINT('Ctrl Pts',(147.000980334791,58.3000000000021,190.730719105988));
#88229=CARTESIAN_POINT('Ctrl Pts',(146.343914360902,58.3000000000039,190.86895978395));
#88230=CARTESIAN_POINT('Ctrl Pts',(145.686309051208,58.3000000000064,191.001857725282));
#88231=CARTESIAN_POINT('Ctrl Pts',(145.236864991416,58.3000000000082,191.092687573232));
#88232=CARTESIAN_POINT('Ctrl Pts',(144.787169000648,58.3000000000102,191.181021754716));
#88233=CARTESIAN_POINT('Ctrl Pts',(144.337226685912,58.3000000000124,191.267047472895));
#88234=CARTESIAN_POINT('Ctrl Pts',(144.128834667865,58.3000000000135,191.306890520389));
#88235=CARTESIAN_POINT('Ctrl Pts',(143.920388679827,58.3000000000144,191.346238581224));
#88236=CARTESIAN_POINT('Ctrl Pts',(143.711897764384,58.3000000000166,191.385108697693));
#88237=CARTESIAN_POINT('Ctrl Pts',(141.950705915482,58.3000000000348,191.713457451624));
#88238=CARTESIAN_POINT('Ctrl Pts',(140.18618180257,58.3000000000201,192.00744782213));
#88239=CARTESIAN_POINT('Ctrl Pts',(138.418978260056,58.3000000000199,192.273910828531));
#88240=CARTESIAN_POINT('Ctrl Pts',(137.546066134828,58.3000000000198,192.405530522368));
#88241=CARTESIAN_POINT('Ctrl Pts',(136.67249987358,58.3000000000189,192.530434774035));
#88242=CARTESIAN_POINT('Ctrl Pts',(135.798359950109,58.300000000037,192.64945104723));
#88243=CARTESIAN_POINT('Ctrl Pts',(133.742775355374,58.3000000000793,192.92932388124));
#88244=CARTESIAN_POINT('Ctrl Pts',(131.684009335516,58.3000000000285,193.176457521784));
#88245=CARTESIAN_POINT('Ctrl Pts',(129.622741670531,58.3000000000104,193.397881860408));
#88246=CARTESIAN_POINT('Ctrl Pts',(129.035162857518,58.3000000000053,193.461000421995));
#88247=CARTESIAN_POINT('Ctrl Pts',(128.447380523824,58.3000000000026,193.522030199221));
#88248=CARTESIAN_POINT('Ctrl Pts',(127.859411366078,58.300000000006,193.581134526229));
#88249=CARTESIAN_POINT('Ctrl Pts',(125.144150532821,58.3000000000217,193.854080244702));
#88250=CARTESIAN_POINT('Ctrl Pts',(122.424955174928,58.3000000000296,194.086609826551));
#88251=CARTESIAN_POINT('Ctrl Pts',(119.702735219,58.3000000000308,194.288037034846));
#88252=CARTESIAN_POINT('Ctrl Pts',(117.52258727193,58.3000000000318,194.449354313301));
#88253=CARTESIAN_POINT('Ctrl Pts',(115.34049946053,58.3000000000286,194.590723963524));
#88254=CARTESIAN_POINT('Ctrl Pts',(113.156940738231,58.3000000000219,194.716950363975));
#88255=CARTESIAN_POINT('Ctrl Pts',(112.748095170393,58.3000000000206,194.740584765853));
#88256=CARTESIAN_POINT('Ctrl Pts',(112.339198168107,58.3000000000193,194.763688308341));
#88257=CARTESIAN_POINT('Ctrl Pts',(111.930252346801,58.3000000000176,194.786292608757));
#88258=CARTESIAN_POINT('Ctrl Pts',(107.974706849214,58.3000000000011,195.004933646458));
#88259=CARTESIAN_POINT('Ctrl Pts',(104.014516979677,58.3000000000813,195.175894172209));
#88260=CARTESIAN_POINT('Ctrl Pts',(100.051160230625,58.3000000000906,195.314262542956));
#88261=CARTESIAN_POINT('Ctrl Pts',(98.6870863726536,58.3000000000937,195.361884972441));
#88262=CARTESIAN_POINT('Ctrl Pts',(97.3226373712284,58.3000000000908,195.4056472157));
#88263=CARTESIAN_POINT('Ctrl Pts',(95.9578737332232,58.3000000000677,195.446165741684));
#88264=CARTESIAN_POINT('Ctrl Pts',(93.2937797771291,58.3000000000226,195.525260141021));
#88265=CARTESIAN_POINT('Ctrl Pts',(90.6283351792062,58.3000000000059,195.591817563437));
#88266=CARTESIAN_POINT('Ctrl Pts',(87.9622980004928,58.3000000000006,195.648477101291));
#88267=CARTESIAN_POINT('Ctrl Pts',(86.4341094435501,58.2999999999976,195.680954689406));
#88268=CARTESIAN_POINT('Ctrl Pts',(84.9057261977232,58.2999999999983,195.710180208743));
#88269=CARTESIAN_POINT('Ctrl Pts',(83.3772911454653,58.2999999999996,195.736650984406));
#88270=CARTESIAN_POINT('Ctrl Pts',(82.3556671155038,58.3000000000005,195.75434436331));
#88271=CARTESIAN_POINT('Ctrl Pts',(81.3340199414989,58.3000000000017,195.770806997954));
#88272=CARTESIAN_POINT('Ctrl Pts',(80.3123923151694,58.3000000000021,195.78618746494));
#88273=CARTESIAN_POINT('Ctrl Pts',(80.1959837797084,58.3000000000022,195.787939979839));
#88274=CARTESIAN_POINT('Ctrl Pts',(80.07957550807,58.3000000000022,195.789678444541));
#88275=CARTESIAN_POINT('Ctrl Pts',(79.963167768534,58.3000000000022,195.791403075907));
#88276=CARTESIAN_POINT('Ctrl Pts',(76.1297303378317,58.3000000000006,195.848197121193));
#88277=CARTESIAN_POINT('Ctrl Pts',(72.296147342554,58.3000000000581,195.889842872884));
#88278=CARTESIAN_POINT('Ctrl Pts',(68.4624943285942,58.3000000000755,195.92117010135));
#88279=CARTESIAN_POINT('Ctrl Pts',(66.9644162966496,58.3000000000824,195.933411854215));
#88280=CARTESIAN_POINT('Ctrl Pts',(65.4663277778819,58.3000000000841,195.944078033995));
#88281=CARTESIAN_POINT('Ctrl Pts',(63.9682326441713,58.3000000000717,195.953457116585));
#88282=CARTESIAN_POINT('Ctrl Pts',(58.6374128389633,58.3000000000276,195.986831632062));
#88283=CARTESIAN_POINT('Ctrl Pts',(53.3064763293957,58.3000000000836,196.004466674216));
#88284=CARTESIAN_POINT('Ctrl Pts',(47.9754976701507,58.3000000001318,196.01317970203));
#88285=CARTESIAN_POINT('Ctrl Pts',(44.2887044272162,58.3000000001652,196.019205449669));
#88286=CARTESIAN_POINT('Ctrl Pts',(40.6018910228219,58.3000000001949,196.020964143901));
#88287=CARTESIAN_POINT('Ctrl Pts',(36.9150820978944,58.3000000001853,196.020712341452));
#88288=CARTESIAN_POINT('Ctrl Pts',(35.270889687944,58.300000000181,196.020600046054));
#88289=CARTESIAN_POINT('Ctrl Pts',(33.6266983124335,58.3000000001696,196.020087903778));
#88290=CARTESIAN_POINT('Ctrl Pts',(31.9825097205404,58.3000000001458,196.019376110131));
#88291=CARTESIAN_POINT('Ctrl Pts',(21.3216725475386,58.2999999999912,196.014760875474));
#88292=CARTESIAN_POINT('Ctrl Pts',(10.6608381121449,58.3,196.));
#88293=CARTESIAN_POINT('Ctrl Pts',(1.06581410364015E-14,58.3,196.));
#88294=CARTESIAN_POINT('Ctrl Pts',(1.20290037631083E-14,55.3,196.));
#88295=CARTESIAN_POINT('Ctrl Pts',(10.7117531408873,55.3,196.));
#88296=CARTESIAN_POINT('Ctrl Pts',(21.4235888453034,55.3,196.014918521175));
#88297=CARTESIAN_POINT('Ctrl Pts',(32.1353671216414,55.3,196.019441470522));
#88298=CARTESIAN_POINT('Ctrl Pts',(37.9435392315241,55.2999999999999,196.0218939175));
#88299=CARTESIAN_POINT('Ctrl Pts',(43.751697287797,55.2999999999995,196.021820075071));
#88300=CARTESIAN_POINT('Ctrl Pts',(49.5597922503515,55.2999999999992,196.010342399909));
#88301=CARTESIAN_POINT('Ctrl Pts',(54.4645376663083,55.2999999999989,196.000649880244));
#88302=CARTESIAN_POINT('Ctrl Pts',(59.3692380077688,55.2999999999989,195.982824984605));
#88303=CARTESIAN_POINT('Ctrl Pts',(64.273863499599,55.2999999999994,195.951525205213));
#88304=CARTESIAN_POINT('Ctrl Pts',(69.6310359294058,55.2999999999999,195.917337413403));
#88305=CARTESIAN_POINT('Ctrl Pts',(74.9881325496578,55.299999999963,195.866500385808));
#88306=CARTESIAN_POINT('Ctrl Pts',(80.3450312167435,55.2999999999824,195.785694345575));
#88307=CARTESIAN_POINT('Ctrl Pts',(82.3276173506661,55.2999999999896,195.7557880612));
#88308=CARTESIAN_POINT('Ctrl Pts',(84.310265521851,55.2999999999926,195.72182275657));
#88309=CARTESIAN_POINT('Ctrl Pts',(86.2928745789687,55.2999999999948,195.682687443605));
#88310=CARTESIAN_POINT('Ctrl Pts',(89.6683015743703,55.2999999999986,195.616058880913));
#88311=CARTESIAN_POINT('Ctrl Pts',(93.0436128903952,55.2999999999982,195.534444136816));
#88312=CARTESIAN_POINT('Ctrl Pts',(96.4182977668295,55.2999999999993,195.432367934215));
#88313=CARTESIAN_POINT('Ctrl Pts',(99.0028738236992,55.3000000000002,195.354190646888));
#88314=CARTESIAN_POINT('Ctrl Pts',(101.586488207725,55.2999999999912,195.264202295603));
#88315=CARTESIAN_POINT('Ctrl Pts',(104.168792975622,55.2999999999847,195.15812279501));
#88316=CARTESIAN_POINT('Ctrl Pts',(106.940470574378,55.2999999999776,195.044263974341));
#88317=CARTESIAN_POINT('Ctrl Pts',(109.71063859809,55.2999999999726,194.911867034808));
#88318=CARTESIAN_POINT('Ctrl Pts',(112.478864925772,55.2999999999828,194.755651977743));
#88319=CARTESIAN_POINT('Ctrl Pts',(114.594741665139,55.2999999999906,194.636249961268));
#88320=CARTESIAN_POINT('Ctrl Pts',(116.709508625892,55.2999999999934,194.503229216588));
#88321=CARTESIAN_POINT('Ctrl Pts',(118.822799974681,55.2999999999957,194.352074481563));
#88322=CARTESIAN_POINT('Ctrl Pts',(121.558121076672,55.2999999999986,194.156428605941));
#88323=CARTESIAN_POINT('Ctrl Pts',(124.290968486144,55.299999999999,193.930400377491));
#88324=CARTESIAN_POINT('Ctrl Pts',(127.020545582271,55.2999999999995,193.664238101445));
#88325=CARTESIAN_POINT('Ctrl Pts',(127.515029972198,55.2999999999997,193.616020708766));
#88326=CARTESIAN_POINT('Ctrl Pts',(128.009407044772,55.2999999999998,193.566486327208));
#88327=CARTESIAN_POINT('Ctrl Pts',(128.503672075522,55.2999999999999,193.515577171767));
#88328=CARTESIAN_POINT('Ctrl Pts',(130.440299623163,55.3000000000005,193.316105093589));
#88329=CARTESIAN_POINT('Ctrl Pts',(132.375181150211,55.2999999999988,193.095177946254));
#88330=CARTESIAN_POINT('Ctrl Pts',(134.307818538159,55.2999999999985,192.846713609731));
#88331=CARTESIAN_POINT('Ctrl Pts',(135.03715051433,55.2999999999985,192.752949002519));
#88332=CARTESIAN_POINT('Ctrl Pts',(135.766163078809,55.2999999999985,192.655263061591));
#88333=CARTESIAN_POINT('Ctrl Pts',(136.494829730513,55.2999999999989,192.553330224408));
#88334=CARTESIAN_POINT('Ctrl Pts',(136.887919350373,55.2999999999991,192.498341101294));
#88335=CARTESIAN_POINT('Ctrl Pts',(137.280909845793,55.2999999999986,192.442107502062));
#88336=CARTESIAN_POINT('Ctrl Pts',(137.673799419673,55.2999999999978,192.38455841101));
#88337=CARTESIAN_POINT('Ctrl Pts',(138.610834346566,55.299999999996,192.247304811242));
#88338=CARTESIAN_POINT('Ctrl Pts',(139.547276689375,55.299999999993,192.102570256913));
#88339=CARTESIAN_POINT('Ctrl Pts',(140.482938496474,55.299999999998,191.949421722643));
#88340=CARTESIAN_POINT('Ctrl Pts',(140.735750542117,55.2999999999994,191.908041606513));
#88341=CARTESIAN_POINT('Ctrl Pts',(140.988534796001,55.2999999999993,191.866041231155));
#88342=CARTESIAN_POINT('Ctrl Pts',(141.241276767632,55.2999999999987,191.823400407199));
#88343=CARTESIAN_POINT('Ctrl Pts',(142.316874400025,55.2999999999962,191.64193324132));
#88344=CARTESIAN_POINT('Ctrl Pts',(143.391615359688,55.2999999999831,191.448879233622));
#88345=CARTESIAN_POINT('Ctrl Pts',(144.462423620222,55.2999999999908,191.243014958559));
#88346=CARTESIAN_POINT('Ctrl Pts',(144.849418372946,55.2999999999936,191.168614716089));
#88347=CARTESIAN_POINT('Ctrl Pts',(145.235966787396,55.2999999999938,191.092555243525));
#88348=CARTESIAN_POINT('Ctrl Pts',(145.622054184335,55.2999999999945,191.014726801987));
#88349=CARTESIAN_POINT('Ctrl Pts',(147.026900291875,55.2999999999974,190.731534488493));
#88350=CARTESIAN_POINT('Ctrl Pts',(148.425595069659,55.2999999999977,190.424926343951));
#88351=CARTESIAN_POINT('Ctrl Pts',(149.816785361501,55.2999999999978,190.089768262817));
#88352=CARTESIAN_POINT('Ctrl Pts',(150.659099488471,55.2999999999978,189.886842474617));
#88353=CARTESIAN_POINT('Ctrl Pts',(151.498662786036,55.2999999999977,189.673451564913));
#88354=CARTESIAN_POINT('Ctrl Pts',(152.33517708753,55.299999999998,189.448465183433));
#88355=CARTESIAN_POINT('Ctrl Pts',(152.632968543411,55.2999999999981,189.368372085234));
#88356=CARTESIAN_POINT('Ctrl Pts',(152.930371374219,55.2999999999987,189.286797545909));
#88357=CARTESIAN_POINT('Ctrl Pts',(153.227374222845,55.2999999999992,189.203666632533));
#88358=CARTESIAN_POINT('Ctrl Pts',(154.1623023375,55.3000000000009,188.941980832308));
#88359=CARTESIAN_POINT('Ctrl Pts',(155.093231051561,55.3000000000026,188.664878292928));
#88360=CARTESIAN_POINT('Ctrl Pts',(156.019362669451,55.2999999999938,188.370172226066));
#88361=CARTESIAN_POINT('Ctrl Pts',(156.084148338743,55.2999999999931,188.349556657591));
#88362=CARTESIAN_POINT('Ctrl Pts',(156.148910538799,55.2999999999925,188.328854968572));
#88363=CARTESIAN_POINT('Ctrl Pts',(156.213648998874,55.2999999999917,188.308066420174));
#88364=CARTESIAN_POINT('Ctrl Pts',(156.416564746944,55.2999999999895,188.242906948592));
#88365=CARTESIAN_POINT('Ctrl Pts',(156.619277412703,55.2999999999878,188.17688312004));
#88366=CARTESIAN_POINT('Ctrl Pts',(156.821789359415,55.299999999986,188.109962014282));
#88367=CARTESIAN_POINT('Ctrl Pts',(157.67443976817,55.2999999999783,187.828199337537));
#88368=CARTESIAN_POINT('Ctrl Pts',(158.523442540595,55.2999999999708,187.530554238279));
#88369=CARTESIAN_POINT('Ctrl Pts',(159.36671167149,55.2999999999747,187.215315781269));
#88370=CARTESIAN_POINT('Ctrl Pts',(159.592281275708,55.2999999999758,187.130991321406));
#88371=CARTESIAN_POINT('Ctrl Pts',(159.817440724798,55.2999999999776,187.045408264328));
#88372=CARTESIAN_POINT('Ctrl Pts',(160.042150350672,55.2999999999805,186.958534466439));
#88373=CARTESIAN_POINT('Ctrl Pts',(160.341043434012,55.2999999999843,186.842980995103));
#88374=CARTESIAN_POINT('Ctrl Pts',(160.638745179164,55.2999999999854,186.725316027712));
#88375=CARTESIAN_POINT('Ctrl Pts',(160.935217111381,55.2999999999872,186.605440010869));
#88376=CARTESIAN_POINT('Ctrl Pts',(162.043912956315,55.2999999999939,186.157147854555));
#88377=CARTESIAN_POINT('Ctrl Pts',(163.135358576353,55.2999999999986,185.677949054978));
#88378=CARTESIAN_POINT('Ctrl Pts',(164.206821631529,55.2999999999996,185.162953213729));
#88379=CARTESIAN_POINT('Ctrl Pts',(165.213812236743,55.3000000000006,184.678945882486));
#88380=CARTESIAN_POINT('Ctrl Pts',(166.203152860742,55.2999999999984,184.163320140631));
#88381=CARTESIAN_POINT('Ctrl Pts',(167.172600012654,55.2999999999914,183.612061848847));
#88382=CARTESIAN_POINT('Ctrl Pts',(167.234668747626,55.299999999991,183.576767604343));
#88383=CARTESIAN_POINT('Ctrl Pts',(167.296655944075,55.2999999999905,183.541327311083));
#88384=CARTESIAN_POINT('Ctrl Pts',(167.358561016714,55.29999999999,183.505739922036));
#88385=CARTESIAN_POINT('Ctrl Pts',(168.39480559842,55.2999999999819,182.910033665581));
#88386=CARTESIAN_POINT('Ctrl Pts',(169.407908306295,55.299999999996,182.272890824595));
#88387=CARTESIAN_POINT('Ctrl Pts',(170.394543441111,55.2999999999993,181.588329526098));
#88388=CARTESIAN_POINT('Ctrl Pts',(170.521203856873,55.2999999999997,181.500448185142));
#88389=CARTESIAN_POINT('Ctrl Pts',(170.647428055806,55.3,181.411785408126));
#88390=CARTESIAN_POINT('Ctrl Pts',(170.773208999519,55.3,181.322328563753));
#88391=CARTESIAN_POINT('Ctrl Pts',(170.892813073087,55.3,181.237264780005));
#88392=CARTESIAN_POINT('Ctrl Pts',(171.01201767922,55.3,181.151481005919));
#88393=CARTESIAN_POINT('Ctrl Pts',(171.130802556229,55.3,181.064975842039));
#88394=CARTESIAN_POINT('Ctrl Pts',(171.50882619844,55.3,180.789679878921));
#88395=CARTESIAN_POINT('Ctrl Pts',(171.882642940618,55.3,180.507051762352));
#88396=CARTESIAN_POINT('Ctrl Pts',(172.252308618058,55.3,180.216507799462));
#88397=CARTESIAN_POINT('Ctrl Pts',(172.303960392832,55.3,180.175911357193));
#88398=CARTESIAN_POINT('Ctrl Pts',(172.355531085545,55.3,180.135160298557));
#88399=CARTESIAN_POINT('Ctrl Pts',(172.407020808966,55.3,180.094252958565));
#88400=CARTESIAN_POINT('Ctrl Pts',(172.455054775581,55.3,180.056091133778));
#88401=CARTESIAN_POINT('Ctrl Pts',(172.503007690529,55.3,180.017800247509));
#88402=CARTESIAN_POINT('Ctrl Pts',(172.550875974094,55.3,179.979382823621));
#88403=CARTESIAN_POINT('Ctrl Pts',(172.597530075614,55.3,179.941939860122));
#88404=CARTESIAN_POINT('Ctrl Pts',(172.644097657435,55.3,179.904381603449));
#88405=CARTESIAN_POINT('Ctrl Pts',(172.6905714067,55.3,179.866713791571));
#88406=CARTESIAN_POINT('Ctrl Pts',(173.036090102331,55.3,179.586664657738));
#88407=CARTESIAN_POINT('Ctrl Pts',(173.37649833556,55.3,179.300504249984));
#88408=CARTESIAN_POINT('Ctrl Pts',(173.710509895914,55.3,179.009174047778));
#88409=CARTESIAN_POINT('Ctrl Pts',(173.799924375868,55.3,178.931185314401));
#88410=CARTESIAN_POINT('Ctrl Pts',(173.888880288647,55.3,178.852825862511));
#88411=CARTESIAN_POINT('Ctrl Pts',(173.977352529315,55.3,178.77411328332));
#88412=CARTESIAN_POINT('Ctrl Pts',(174.086885478565,55.3,178.676663271014));
#88413=CARTESIAN_POINT('Ctrl Pts',(174.195746807261,55.3,178.578606701701));
#88414=CARTESIAN_POINT('Ctrl Pts',(174.303919095228,55.3,178.479961005701));
#88415=CARTESIAN_POINT('Ctrl Pts',(174.958585095774,55.3,177.882950583855));
#88416=CARTESIAN_POINT('Ctrl Pts',(175.588161561579,55.3,177.264237409506));
#88417=CARTESIAN_POINT('Ctrl Pts',(176.192889041399,55.3,176.624027678017));
#88418=CARTESIAN_POINT('Ctrl Pts',(176.801495030497,55.3,175.979711866572));
#88419=CARTESIAN_POINT('Ctrl Pts',(177.384932282356,55.3,175.313622824482));
#88420=CARTESIAN_POINT('Ctrl Pts',(177.943406015761,55.3,174.62593595727));
#88421=CARTESIAN_POINT('Ctrl Pts',(178.443543934614,55.3,174.010081964474));
#88422=CARTESIAN_POINT('Ctrl Pts',(178.923660583429,55.3,173.376906026298));
#88423=CARTESIAN_POINT('Ctrl Pts',(179.383876297428,55.3,172.726511192076));
#88424=CARTESIAN_POINT('Ctrl Pts',(179.775881961457,55.3,172.172513466411));
#88425=CARTESIAN_POINT('Ctrl Pts',(180.153586615474,55.3,171.606136536173));
#88426=CARTESIAN_POINT('Ctrl Pts',(180.517306782578,55.3,171.027671453042));
#88427=CARTESIAN_POINT('Ctrl Pts',(180.773257893905,55.3,170.620603618255));
#88428=CARTESIAN_POINT('Ctrl Pts',(181.022282246798,55.3,170.20742155264));
#88429=CARTESIAN_POINT('Ctrl Pts',(181.263216383822,55.3,169.7908638695));
#88430=CARTESIAN_POINT('Ctrl Pts',(181.364433858471,55.3,169.615866182357));
#88431=CARTESIAN_POINT('Ctrl Pts',(181.46422337679,55.2999999999999,169.44027295065));
#88432=CARTESIAN_POINT('Ctrl Pts',(181.562498312604,55.2999999999999,169.264287803902));
#88433=CARTESIAN_POINT('Ctrl Pts',(181.963798726816,55.2999999999999,168.545661923348));
#88434=CARTESIAN_POINT('Ctrl Pts',(182.341571888111,55.3,167.817934400603));
#88435=CARTESIAN_POINT('Ctrl Pts',(182.698078757659,55.3,167.081978998468));
#88436=CARTESIAN_POINT('Ctrl Pts',(182.93109709914,55.3,166.600947293731));
#88437=CARTESIAN_POINT('Ctrl Pts',(183.155030282405,55.3,166.116400730355));
#88438=CARTESIAN_POINT('Ctrl Pts',(183.370511496512,55.3,165.628584399066));
#88439=CARTESIAN_POINT('Ctrl Pts',(183.755753078273,55.3,164.756456701743));
#88440=CARTESIAN_POINT('Ctrl Pts',(184.114155490382,55.3,163.873945121211));
#88441=CARTESIAN_POINT('Ctrl Pts',(184.448595318293,55.3,162.982163050726));
#88442=CARTESIAN_POINT('Ctrl Pts',(184.791126490202,55.3,162.068805453339));
#88443=CARTESIAN_POINT('Ctrl Pts',(185.108521565696,55.3,161.145723431531));
#88444=CARTESIAN_POINT('Ctrl Pts',(185.403902175355,55.3,160.21412492318));
#88445=CARTESIAN_POINT('Ctrl Pts',(185.613942848109,55.3,159.551679349462));
#88446=CARTESIAN_POINT('Ctrl Pts',(185.812852754154,55.3,158.884927731768));
#88447=CARTESIAN_POINT('Ctrl Pts',(186.001763361621,55.3,158.21430775209));
#88448=CARTESIAN_POINT('Ctrl Pts',(186.02001879619,55.3,158.149502184398));
#88449=CARTESIAN_POINT('Ctrl Pts',(186.038180866162,55.3,158.084660468995));
#88450=CARTESIAN_POINT('Ctrl Pts',(186.056250572068,55.3,158.01978308872));
#88451=CARTESIAN_POINT('Ctrl Pts',(186.24876776852,55.3,157.328570324747));
#88452=CARTESIAN_POINT('Ctrl Pts',(186.430890225782,55.3,156.63235380753));
#88453=CARTESIAN_POINT('Ctrl Pts',(186.603184808282,55.3,155.933322134126));
#88454=CARTESIAN_POINT('Ctrl Pts',(186.726566943441,55.3,155.43273750078));
#88455=CARTESIAN_POINT('Ctrl Pts',(186.8449092848,55.3,154.930709442874));
#88456=CARTESIAN_POINT('Ctrl Pts',(186.958421359116,55.3,154.428044900815));
#88457=CARTESIAN_POINT('Ctrl Pts',(186.984076143135,55.3,154.314438041474));
#88458=CARTESIAN_POINT('Ctrl Pts',(187.009484234522,55.3,154.20079852715));
#88459=CARTESIAN_POINT('Ctrl Pts',(187.034647948172,55.3,154.087136197122));
#88460=CARTESIAN_POINT('Ctrl Pts',(187.249235230063,55.3,153.117863903177));
#88461=CARTESIAN_POINT('Ctrl Pts',(187.446091592081,55.2999999999899,152.147366177988));
#88462=CARTESIAN_POINT('Ctrl Pts',(187.627848642994,55.2999999999872,151.175802209577));
#88463=CARTESIAN_POINT('Ctrl Pts',(187.693091728517,55.2999999999863,150.8270518818));
#88464=CARTESIAN_POINT('Ctrl Pts',(187.756389466396,55.2999999999861,150.478163958403));
#88465=CARTESIAN_POINT('Ctrl Pts',(187.817864007364,55.2999999999881,150.129146500694));
#88466=CARTESIAN_POINT('Ctrl Pts',(188.069630152066,55.2999999999964,148.699761614247));
#88467=CARTESIAN_POINT('Ctrl Pts',(188.291104411737,55.2999999999992,147.268244191048));
#88468=CARTESIAN_POINT('Ctrl Pts',(188.488029524791,55.2999999999999,145.834998434922));
#88469=CARTESIAN_POINT('Ctrl Pts',(188.654658802898,55.3000000000006,144.622249578312));
#88470=CARTESIAN_POINT('Ctrl Pts',(188.803712719525,55.2999999999995,143.408263343521));
#88471=CARTESIAN_POINT('Ctrl Pts',(188.938699247615,55.2999999999996,142.193285856766));
#88472=CARTESIAN_POINT('Ctrl Pts',(189.136760801143,55.2999999999999,140.410587005753));
#88473=CARTESIAN_POINT('Ctrl Pts',(189.304299717647,55.2999999999999,138.625739912856));
#88474=CARTESIAN_POINT('Ctrl Pts',(189.448306949797,55.3,136.839236134823));
#88475=CARTESIAN_POINT('Ctrl Pts',(189.518148375124,55.3,135.972807634335));
#88476=CARTESIAN_POINT('Ctrl Pts',(189.582455728296,55.3,135.105989526119));
#88477=CARTESIAN_POINT('Ctrl Pts',(189.642030732453,55.3,134.238837995224));
#88478=CARTESIAN_POINT('Ctrl Pts',(189.792507914843,55.3,132.048548276901));
#88479=CARTESIAN_POINT('Ctrl Pts',(189.91260648438,55.3,129.856119556288));
#88480=CARTESIAN_POINT('Ctrl Pts',(190.010856013085,55.3,127.662152697902));
#88481=CARTESIAN_POINT('Ctrl Pts',(190.031601906391,55.3,127.198885311674));
#88482=CARTESIAN_POINT('Ctrl Pts',(190.051373807095,55.3,126.735549363847));
#88483=CARTESIAN_POINT('Ctrl Pts',(190.070252291175,55.3,126.272150491645));
#88484=CARTESIAN_POINT('Ctrl Pts',(190.155978348671,55.3,124.167884164185));
#88485=CARTESIAN_POINT('Ctrl Pts',(190.223186981995,55.3,122.062313754707));
#88486=CARTESIAN_POINT('Ctrl Pts',(190.277034501585,55.3,119.955802788295));
#88487=CARTESIAN_POINT('Ctrl Pts',(190.291163140251,55.3,119.403091493176));
#88488=CARTESIAN_POINT('Ctrl Pts',(190.304372045238,55.3,118.850315409215));
#88489=CARTESIAN_POINT('Ctrl Pts',(190.316754563799,55.3,118.297481238445));
#88490=CARTESIAN_POINT('Ctrl Pts',(190.397155299449,55.3,114.707882418131));
#88491=CARTESIAN_POINT('Ctrl Pts',(190.443516406214,55.3,111.115886118275));
#88492=CARTESIAN_POINT('Ctrl Pts',(190.471166981729,55.3,107.522572589343));
#88493=CARTESIAN_POINT('Ctrl Pts',(190.484470219953,55.3,105.793758450732));
#88494=CARTESIAN_POINT('Ctrl Pts',(190.493443302223,55.3,104.064639447949));
#88495=CARTESIAN_POINT('Ctrl Pts',(190.499797482064,55.3,102.335336081499));
#88496=CARTESIAN_POINT('Origin',(-122.710817715584,2.44173312008429,40.));
#88497=CARTESIAN_POINT('',(190.,55.3,40.));
#88498=CARTESIAN_POINT('',(-190.,55.3,40.));
#88499=CARTESIAN_POINT('',(-190.5,55.3,40.));
#88500=CARTESIAN_POINT('',(-190.,58.2999999999999,40.));
#88501=CARTESIAN_POINT('',(-190.,58.8,40.));
#88502=CARTESIAN_POINT('',(190.,58.3,40.));
#88503=CARTESIAN_POINT('',(190.5,58.3,40.));
#88504=CARTESIAN_POINT('',(190.,54.8,40.));
#88505=CARTESIAN_POINT('Origin',(-190.5,58.8,211.4));
#88506=CARTESIAN_POINT('',(-190.5,58.2999999999999,40.5));
#88507=CARTESIAN_POINT('',(-190.5,58.2999999999999,211.4));
#88508=CARTESIAN_POINT('',(-190.5,55.3,40.5));
#88509=CARTESIAN_POINT('',(-190.5,54.8,40.5));
#88510=CARTESIAN_POINT('',(-190.5,55.3,211.4));
#88511=CARTESIAN_POINT('Origin',(190.5,58.8,211.4));
#88512=CARTESIAN_POINT('',(190.5,55.3,40.5));
#88513=CARTESIAN_POINT('',(190.5,58.3,40.5));
#88514=CARTESIAN_POINT('',(190.5,58.8,40.5));
#88515=CARTESIAN_POINT('',(190.5,58.3,211.4));
#88516=CARTESIAN_POINT('',(190.5,55.3,211.4));
#88517=CARTESIAN_POINT('Ctrl Pts',(1.19489048671551E-14,54.8498893695668,
195.717716375983));
#88518=CARTESIAN_POINT('Ctrl Pts',(1.20290037631083E-14,54.9864286189535,
196.));
#88519=CARTESIAN_POINT('Ctrl Pts',(1.20290037631083E-14,55.3,196.));
#88520=CARTESIAN_POINT('Ctrl Pts',(10.7116410653504,54.8498893695294,195.717716376117));
#88521=CARTESIAN_POINT('Ctrl Pts',(10.7114086955983,54.9864286188836,196.000000000093));
#88522=CARTESIAN_POINT('Ctrl Pts',(10.7114086955983,55.3,196.));
#88523=CARTESIAN_POINT('Ctrl Pts',(21.4234737060142,54.8498893695169,195.732634823405));
#88524=CARTESIAN_POINT('Ctrl Pts',(21.4231418325433,54.9864286188603,196.014918332448));
#88525=CARTESIAN_POINT('Ctrl Pts',(21.4231418325433,55.3,196.014918332428));
#88526=CARTESIAN_POINT('Ctrl Pts',(42.8474989205484,54.8498893696167,195.741680919933));
#88527=CARTESIAN_POINT('Ctrl Pts',(42.8475924107395,54.9864286190467,196.023964608597));
#88528=CARTESIAN_POINT('Ctrl Pts',(42.8475924107395,55.3,196.023964608617));
#88529=CARTESIAN_POINT('Ctrl Pts',(53.5596882551516,54.8498893695668,195.737610334586));
#88530=CARTESIAN_POINT('Ctrl Pts',(53.560285285152,54.9864286189535,196.01989589653));
#88531=CARTESIAN_POINT('Ctrl Pts',(53.5602852851508,55.3,196.019895896344));
#88532=CARTESIAN_POINT('Ctrl Pts',(69.6282490087062,54.8498893695668,195.635065826431));
#88533=CARTESIAN_POINT('Ctrl Pts',(69.6306526068224,54.9864286189535,195.917339859554));
#88534=CARTESIAN_POINT('Ctrl Pts',(69.630652606823,55.3,195.917339859647));
#88535=CARTESIAN_POINT('Ctrl Pts',(74.9844823357142,54.8498893695756,195.584239709646));
#88536=CARTESIAN_POINT('Ctrl Pts',(74.9876678041973,54.986428618963,195.866507396292));
#88537=CARTESIAN_POINT('Ctrl Pts',(74.9876678041967,55.2999999999628,195.866507396253));
#88538=CARTESIAN_POINT('Ctrl Pts',(85.6970648621475,54.849889369558,195.422645953774));
#88539=CARTESIAN_POINT('Ctrl Pts',(85.7023946292896,54.9864286189441,195.704881294858));
#88540=CARTESIAN_POINT('Ctrl Pts',(85.7023946292902,55.3000000000371,195.704881294897));
#88541=CARTESIAN_POINT('Ctrl Pts',(91.054003880559,54.8498893696168,195.312212356202));
#88542=CARTESIAN_POINT('Ctrl Pts',(91.0606918125482,54.9864286190468,195.594422789953));
#88543=CARTESIAN_POINT('Ctrl Pts',(91.0606918125484,55.3,195.594422789964));
#88544=CARTESIAN_POINT('Ctrl Pts',(101.765522641295,54.8498893695169,194.988214353708));
#88545=CARTESIAN_POINT('Ctrl Pts',(101.775903721111,54.9864286188603,195.270313078475));
#88546=CARTESIAN_POINT('Ctrl Pts',(101.77590372111,55.3,195.270313078465));
#88547=CARTESIAN_POINT('Ctrl Pts',(107.117519783562,54.8498893695382,194.77546778461));
#88548=CARTESIAN_POINT('Ctrl Pts',(107.130224336095,54.9864286188931,195.057483582449));
#88549=CARTESIAN_POINT('Ctrl Pts',(107.130224336101,55.2999999999628,195.057483582545));
#88550=CARTESIAN_POINT('Ctrl Pts',(117.808401320513,54.8498893695954,194.172165716499));
#88551=CARTESIAN_POINT('Ctrl Pts',(117.827505515449,54.9864286190139,194.453820373037));
#88552=CARTESIAN_POINT('Ctrl Pts',(117.827505515444,55.3000000000371,194.453820372941));
#88553=CARTESIAN_POINT('Ctrl Pts',(123.147415580818,54.8498893695419,193.783493005426));
#88554=CARTESIAN_POINT('Ctrl Pts',(123.170566875688,54.986428618907,194.064885467392));
#88555=CARTESIAN_POINT('Ctrl Pts',(123.170566875683,55.3,194.06488546734));
#88556=CARTESIAN_POINT('Ctrl Pts',(131.138417142893,54.8498893695793,192.960422151946));
#88557=CARTESIAN_POINT('Ctrl Pts',(131.170224675439,54.9864286189768,193.240923023955));
#88558=CARTESIAN_POINT('Ctrl Pts',(131.170224675442,55.3,193.240923023981));
#88559=CARTESIAN_POINT('Ctrl Pts',(133.799118380507,54.8498893695668,192.645399766939));
#88560=CARTESIAN_POINT('Ctrl Pts',(133.834251546586,54.9864286189535,192.925517262466));
#88561=CARTESIAN_POINT('Ctrl Pts',(133.834251546587,55.3,192.925517262471));
#88562=CARTESIAN_POINT('Ctrl Pts',(137.784023815075,54.8498893695668,192.08795320905));
#88563=CARTESIAN_POINT('Ctrl Pts',(137.825118822477,54.9864286189535,192.367236705379));
#88564=CARTESIAN_POINT('Ctrl Pts',(137.825118822477,55.3,192.367236705376));
#88565=CARTESIAN_POINT('Ctrl Pts',(139.111294699818,54.8498893695628,191.887891561296));
#88566=CARTESIAN_POINT('Ctrl Pts',(139.154540611869,54.9864286189442,192.166853050329));
#88567=CARTESIAN_POINT('Ctrl Pts',(139.154540611864,55.2999999999907,192.1668530503));
#88568=CARTESIAN_POINT('Ctrl Pts',(141.763387800952,54.8498893695709,191.453798635637));
#88569=CARTESIAN_POINT('Ctrl Pts',(141.81133638108,54.9864286189629,191.731990394956));
#88570=CARTESIAN_POINT('Ctrl Pts',(141.811336381084,55.3000000000093,191.731990394986));
#88571=CARTESIAN_POINT('Ctrl Pts',(143.089104272173,54.8498893695493,191.219584409738));
#88572=CARTESIAN_POINT('Ctrl Pts',(143.139606665644,54.9864286189174,191.497328231536));
#88573=CARTESIAN_POINT('Ctrl Pts',(143.139606665632,55.2999999999813,191.497328231471));
#88574=CARTESIAN_POINT('Ctrl Pts',(147.049181964921,54.8498893696018,190.458254343683));
#88575=CARTESIAN_POINT('Ctrl Pts',(147.108057529376,54.9864286190258,190.734388412604));
#88576=CARTESIAN_POINT('Ctrl Pts',(147.108057529402,55.3000000000372,190.734388412735));
#88577=CARTESIAN_POINT('Ctrl Pts',(149.669629595343,54.8498893695668,189.873067582401));
#88578=CARTESIAN_POINT('Ctrl Pts',(149.735031156397,54.9864286189535,190.147792646745));
#88579=CARTESIAN_POINT('Ctrl Pts',(149.73503115636,55.2999999999999,190.147792646608));
#88580=CARTESIAN_POINT('Ctrl Pts',(153.557975830725,54.8498893695668,188.827269622761));
#88581=CARTESIAN_POINT('Ctrl Pts',(153.635250053096,54.9864286189535,189.098801451777));
#88582=CARTESIAN_POINT('Ctrl Pts',(153.635250053114,55.2999999999999,189.098801451845));
#88583=CARTESIAN_POINT('Ctrl Pts',(154.846981325738,54.8498893695781,188.450444611742));
#88584=CARTESIAN_POINT('Ctrl Pts',(154.928562946898,54.986428618978,188.720727975022));
#88585=CARTESIAN_POINT('Ctrl Pts',(154.928562946869,55.3000000000186,188.720727974942));
#88586=CARTESIAN_POINT('Ctrl Pts',(157.407706254429,54.8498893695556,187.628155140046));
#88587=CARTESIAN_POINT('Ctrl Pts',(157.49873505085,54.9864286189291,187.895404865325));
#88588=CARTESIAN_POINT('Ctrl Pts',(157.498735050879,55.2999999999814,187.895404865405));
#88589=CARTESIAN_POINT('Ctrl Pts',(158.680831044999,54.8498893695443,187.182182108568));
#88590=CARTESIAN_POINT('Ctrl Pts',(158.777006808679,54.9864286189044,187.447644908267));
#88591=CARTESIAN_POINT('Ctrl Pts',(158.777006808638,55.2999999999626,187.447644908161));
#88592=CARTESIAN_POINT('Ctrl Pts',(162.459418845047,54.8498893696119,185.721362298639));
#88593=CARTESIAN_POINT('Ctrl Pts',(162.572437434659,54.9864286190517,185.980313582784));
#88594=CARTESIAN_POINT('Ctrl Pts',(162.572437434741,55.3000000000747,185.980313582995));
#88595=CARTESIAN_POINT('Ctrl Pts',(164.895888522176,54.849889369586,184.595853659769));
#88596=CARTESIAN_POINT('Ctrl Pts',(165.021947502581,54.9864286189963,184.848989685788));
#88597=CARTESIAN_POINT('Ctrl Pts',(165.021947502437,55.300000000037,184.848989685601));
#88598=CARTESIAN_POINT('Ctrl Pts',(168.378867687188,54.8498893695572,182.593592304728));
#88599=CARTESIAN_POINT('Ctrl Pts',(168.526867773781,54.9864286189321,182.83411504016));
#88600=CARTESIAN_POINT('Ctrl Pts',(168.526867773853,55.2999999999815,182.834115040254));
#88601=CARTESIAN_POINT('Ctrl Pts',(169.511081787078,54.8498893695574,181.873572185375));
#88602=CARTESIAN_POINT('Ctrl Pts',(169.66677678621,54.986428618936,182.109235796402));
#88603=CARTESIAN_POINT('Ctrl Pts',(169.666776786129,55.3,182.109235796287));
#88604=CARTESIAN_POINT('Ctrl Pts',(171.158864505137,54.8498893695715,180.701650287951));
#88605=CARTESIAN_POINT('Ctrl Pts',(171.326425106174,54.9864286189623,180.928874947428));
#88606=CARTESIAN_POINT('Ctrl Pts',(171.326425106214,55.3,180.928874947486));
#88607=CARTESIAN_POINT('Ctrl Pts',(171.699692855963,54.8498893695652,180.295680572782));
#88608=CARTESIAN_POINT('Ctrl Pts',(171.871260701908,54.9864286189506,180.519901406498));
#88609=CARTESIAN_POINT('Ctrl Pts',(171.871260701868,55.3,180.51990140644));
#88610=CARTESIAN_POINT('Ctrl Pts',(172.763157385062,54.8498893695684,179.45078372375));
#88611=CARTESIAN_POINT('Ctrl Pts',(172.942780916024,54.9864286189565,179.668604510632));
#88612=CARTESIAN_POINT('Ctrl Pts',(172.942780916064,55.3,179.668604510689));
#88613=CARTESIAN_POINT('Ctrl Pts',(173.284486233779,54.8498893695692,179.012714799304));
#88614=CARTESIAN_POINT('Ctrl Pts',(173.468148508341,54.9864286189579,179.227145347657));
#88615=CARTESIAN_POINT('Ctrl Pts',(173.468148508335,55.3,179.227145347651));
#88616=CARTESIAN_POINT('Ctrl Pts',(175.810652663565,54.8498893695574,176.76521802901));
#88617=CARTESIAN_POINT('Ctrl Pts',(176.014168613212,54.986428618936,176.961985025973));
#88618=CARTESIAN_POINT('Ctrl Pts',(176.014168613234,55.3,176.961985025999));
#88619=CARTESIAN_POINT('Ctrl Pts',(177.597042024351,54.8498893695856,174.763030220158));
#88620=CARTESIAN_POINT('Ctrl Pts',(177.815415056872,54.9864286189885,174.94312191924));
#88621=CARTESIAN_POINT('Ctrl Pts',(177.81541505695,55.3,174.943121919295));
#88622=CARTESIAN_POINT('Ctrl Pts',(179.542546567764,54.8498893695622,172.013567161068));
#88623=CARTESIAN_POINT('Ctrl Pts',(179.775991607566,54.9864286189448,172.172358510285));
#88624=CARTESIAN_POINT('Ctrl Pts',(179.775991607547,55.3,172.172358510271));
#88625=CARTESIAN_POINT('Ctrl Pts',(179.917402670385,54.8498893695668,171.451447836108));
#88626=CARTESIAN_POINT('Ctrl Pts',(180.153696573191,54.9864286189535,171.605961657991));
#88627=CARTESIAN_POINT('Ctrl Pts',(180.153696573218,55.3,171.605961658008));
#88628=CARTESIAN_POINT('Ctrl Pts',(180.639269900445,54.8498893695668,170.303381204245));
#88629=CARTESIAN_POINT('Ctrl Pts',(180.880916991964,54.9864286189535,170.449381248092));
#88630=CARTESIAN_POINT('Ctrl Pts',(180.880916991938,55.3,170.449381248076));
#88631=CARTESIAN_POINT('Ctrl Pts',(180.986269545301,54.8498893695668,169.71719072451));
#88632=CARTESIAN_POINT('Ctrl Pts',(181.230420402754,54.9864286189535,169.858953973853));
#88633=CARTESIAN_POINT('Ctrl Pts',(181.230420402816,55.3,169.858953973888));
#88634=CARTESIAN_POINT('Ctrl Pts',(181.9755782218,54.8498893695668,167.945593204617));
#88635=CARTESIAN_POINT('Ctrl Pts',(182.226654132303,54.9864286189535,168.074955463999));
#88636=CARTESIAN_POINT('Ctrl Pts',(182.226654132179,55.3,168.07495546393));
#88637=CARTESIAN_POINT('Ctrl Pts',(182.570885742225,54.8498893695668,166.740197827949));
#88638=CARTESIAN_POINT('Ctrl Pts',(182.825829796685,54.9864286189535,166.86166000408));
#88639=CARTESIAN_POINT('Ctrl Pts',(182.825829796816,55.3,166.861660004138));
#88640=CARTESIAN_POINT('Ctrl Pts',(184.195121388266,54.8498893695668,163.063178107394));
#88641=CARTESIAN_POINT('Ctrl Pts',(184.459874896166,54.9864286189535,163.162433189036));
#88642=CARTESIAN_POINT('Ctrl Pts',(184.459874895903,55.3,163.16243318892));
#88643=CARTESIAN_POINT('Ctrl Pts',(185.06372001807,54.8498893695668,160.531273278361));
#88644=CARTESIAN_POINT('Ctrl Pts',(185.332658084462,54.9864286189535,160.617765878982));
#88645=CARTESIAN_POINT('Ctrl Pts',(185.332658084646,55.3,160.617765879034));
#88646=CARTESIAN_POINT('Ctrl Pts',(186.144616122717,54.8498893695668,156.650429397757));
#88647=CARTESIAN_POINT('Ctrl Pts',(186.418046815871,54.9864286189535,156.720791693588));
#88648=CARTESIAN_POINT('Ctrl Pts',(186.418046815779,55.3,156.720791693563));
#88649=CARTESIAN_POINT('Ctrl Pts',(186.46824053002,54.8498893695543,155.339625317485));
#88650=CARTESIAN_POINT('Ctrl Pts',(186.742866764419,54.9864286189301,155.405086705306));
#88651=CARTESIAN_POINT('Ctrl Pts',(186.742866764507,55.3,155.405086705325));
#88652=CARTESIAN_POINT('Ctrl Pts',(187.049835163757,54.8498893695793,152.712612385649));
#88653=CARTESIAN_POINT('Ctrl Pts',(187.326429131926,54.9864286189768,152.769185688938));
#88654=CARTESIAN_POINT('Ctrl Pts',(187.326429131838,55.3,152.769185688918));
#88655=CARTESIAN_POINT('Ctrl Pts',(187.307891131261,54.8498893695494,151.397166218267));
#88656=CARTESIAN_POINT('Ctrl Pts',(187.585258126244,54.9864286189176,151.449750314472));
#88657=CARTESIAN_POINT('Ctrl Pts',(187.585258126311,55.2999999999814,151.449750314484));
#88658=CARTESIAN_POINT('Ctrl Pts',(188.00379723173,54.8498893696016,147.446207430077));
#88659=CARTESIAN_POINT('Ctrl Pts',(188.283075769604,54.9864286190254,147.487938873138));
#88660=CARTESIAN_POINT('Ctrl Pts',(188.283075769471,55.300000000037,147.487938873115));
#88661=CARTESIAN_POINT('Ctrl Pts',(188.364385942478,54.8498893695668,144.806133531479));
#88662=CARTESIAN_POINT('Ctrl Pts',(188.644410165646,54.9864286189535,144.842102846927));
#88663=CARTESIAN_POINT('Ctrl Pts',(188.644410165762,55.3,144.84210284694));
#88664=CARTESIAN_POINT('Ctrl Pts',(188.951897791745,54.8498893695668,139.51809716399));
#88665=CARTESIAN_POINT('Ctrl Pts',(189.232988329585,54.9864286189535,139.544468866606));
#88666=CARTESIAN_POINT('Ctrl Pts',(189.232988329468,55.3,139.544468866593));
#88667=CARTESIAN_POINT('Ctrl Pts',(189.178308705455,54.8498893695668,136.870102382931));
#88668=CARTESIAN_POINT('Ctrl Pts',(189.45970916863,54.9864286189535,136.892642646069));
#88669=CARTESIAN_POINT('Ctrl Pts',(189.459709168719,55.3,136.892642646075));
#88670=CARTESIAN_POINT('Ctrl Pts',(189.542513180321,54.8498893695668,131.568877948139));
#88671=CARTESIAN_POINT('Ctrl Pts',(189.824352296276,54.9864286189535,131.585033344378));
#88672=CARTESIAN_POINT('Ctrl Pts',(189.824352296186,55.3,131.585033344372));
#88673=CARTESIAN_POINT('Ctrl Pts',(189.68004124865,54.8498893695668,128.915632750363));
#88674=CARTESIAN_POINT('Ctrl Pts',(189.962004740436,54.9864286189535,128.929238460971));
#88675=CARTESIAN_POINT('Ctrl Pts',(189.962004740445,55.3,128.929238460971));
#88676=CARTESIAN_POINT('Ctrl Pts',(189.89636400371,54.8498893695668,123.605687296072));
#88677=CARTESIAN_POINT('Ctrl Pts',(190.178499841913,54.9864286189535,123.615062522318));
#88678=CARTESIAN_POINT('Ctrl Pts',(190.178499841904,55.3,123.615062522318));
#88679=CARTESIAN_POINT('Ctrl Pts',(189.975011236078,54.8498893695668,120.9489786286));
#88680=CARTESIAN_POINT('Ctrl Pts',(190.257193263767,54.9864286189535,120.956675467105));
#88681=CARTESIAN_POINT('Ctrl Pts',(190.257193263798,55.3,120.956675467117));
#88682=CARTESIAN_POINT('Ctrl Pts',(190.155938877336,54.8498893695668,112.871221107224));
#88683=CARTESIAN_POINT('Ctrl Pts',(190.438214558407,54.9864286189535,112.874736662693));
#88684=CARTESIAN_POINT('Ctrl Pts',(190.438214558344,55.3,112.874736662668));
#88685=CARTESIAN_POINT('Ctrl Pts',(190.199675585056,54.8498893695475,107.446717574517));
#88686=CARTESIAN_POINT('Ctrl Pts',(190.481953816303,54.9864286189174,107.448676238389));
#88687=CARTESIAN_POINT('Ctrl Pts',(190.481953816244,55.3,107.448676238409));
#88688=CARTESIAN_POINT('Ctrl Pts',(190.218638436563,54.849889369568,102.021063856015));
#88689=CARTESIAN_POINT('Ctrl Pts',(190.500920367765,54.9864286189556,102.022043932952));
#88690=CARTESIAN_POINT('Ctrl Pts',(190.500920367768,55.3,102.022043932951));
#88691=CARTESIAN_POINT('',(119.410706527861,54.8500000000013,194.026226514646));
#88692=CARTESIAN_POINT('',(1.20290037631083E-14,54.8500000000093,195.717944947196));
#88693=CARTESIAN_POINT('Ctrl Pts',(119.410743668763,54.8500000000039,194.026733883575));
#88694=CARTESIAN_POINT('Ctrl Pts',(117.096090401041,54.8500000000093,194.196173327592));
#88695=CARTESIAN_POINT('Ctrl Pts',(114.779973647168,54.8500000000123,194.343293250508));
#88696=CARTESIAN_POINT('Ctrl Pts',(112.462973430155,54.8499999999998,194.474044958672));
#88697=CARTESIAN_POINT('Ctrl Pts',(110.006841798142,54.8499999999867,194.612648055902));
#88698=CARTESIAN_POINT('Ctrl Pts',(107.549690002739,54.8499999999751,194.732460623929));
#88699=CARTESIAN_POINT('Ctrl Pts',(105.091970605807,54.8499999999712,194.837192076906));
#88700=CARTESIAN_POINT('Ctrl Pts',(103.554266624083,54.8499999999688,194.902718667311));
#88701=CARTESIAN_POINT('Ctrl Pts',(102.0163496059,54.8499999999694,194.962341604715));
#88702=CARTESIAN_POINT('Ctrl Pts',(100.478225211469,54.8499999999746,195.016972545393));
#88703=CARTESIAN_POINT('Ctrl Pts',(99.122234956026,54.8499999999792,195.065134464853));
#88704=CARTESIAN_POINT('Ctrl Pts',(97.7660827406174,54.8499999999872,195.109416587705));
#88705=CARTESIAN_POINT('Ctrl Pts',(96.4097701715019,54.8499999999999,195.150441821658));
#88706=CARTESIAN_POINT('Ctrl Pts',(94.6308236322866,54.8500000000165,195.204250729445));
#88707=CARTESIAN_POINT('Ctrl Pts',(92.8518861601934,54.8500000000211,195.252366591768));
#88708=CARTESIAN_POINT('Ctrl Pts',(91.0729256581933,54.8500000000201,195.29559716179));
#88709=CARTESIAN_POINT('Ctrl Pts',(90.1129897448902,54.8500000000196,195.318924591865));
#88710=CARTESIAN_POINT('Ctrl Pts',(89.1530495490921,54.8500000000175,195.340829459218));
#88711=CARTESIAN_POINT('Ctrl Pts',(88.1930835376938,54.8500000000148,195.361438701481));
#88712=CARTESIAN_POINT('Ctrl Pts',(85.5757330912171,54.8500000000074,195.417629867416));
#88713=CARTESIAN_POINT('Ctrl Pts',(82.9582317068191,54.8499999999956,195.464188429785));
#88714=CARTESIAN_POINT('Ctrl Pts',(80.3407770464166,54.8499999999998,195.503671376904));
#88715=CARTESIAN_POINT('Ctrl Pts',(78.4437598294776,54.8500000000029,195.532286898538));
#88716=CARTESIAN_POINT('Ctrl Pts',(76.5466931771328,54.8500000000039,195.557143922092));
#88717=CARTESIAN_POINT('Ctrl Pts',(74.6495706553743,54.8500000000037,195.578833932771));
#88718=CARTESIAN_POINT('Ctrl Pts',(71.1904981133586,54.8500000000035,195.618381890013));
#88719=CARTESIAN_POINT('Ctrl Pts',(67.7313184321388,54.8500276561664,195.647457113546));
#88720=CARTESIAN_POINT('Ctrl Pts',(64.2720640515808,54.8500381138508,195.669554571807));
#88721=CARTESIAN_POINT('Ctrl Pts',(62.7549036160415,54.850042700384,195.679246079199));
#88722=CARTESIAN_POINT('Ctrl Pts',(61.2377288142738,54.8500439773173,195.687641278906));
#88723=CARTESIAN_POINT('Ctrl Pts',(59.7205427111412,54.8500381593574,195.694890495738));
#88724=CARTESIAN_POINT('Ctrl Pts',(50.5258276199189,54.8500029003453,195.738823460365));
#88725=CARTESIAN_POINT('Ctrl Pts',(41.3306706881903,54.8500518450573,195.741376041741));
#88726=CARTESIAN_POINT('Ctrl Pts',(32.1354861856875,54.8500356591211,195.737460054359));
#88727=CARTESIAN_POINT('Ctrl Pts',(31.3771645488717,54.8500343242762,195.737137105106));
#88728=CARTESIAN_POINT('Ctrl Pts',(30.6188427437782,54.8500325464933,195.736761144975));
#88729=CARTESIAN_POINT('Ctrl Pts',(29.8605210106052,54.8500302420968,195.736340981459));
#88730=CARTESIAN_POINT('Ctrl Pts',(19.9070136065305,54.849999995267,195.730826039073));
#88731=CARTESIAN_POINT('Ctrl Pts',(9.95351054027871,54.849999999965,195.717944947301));
#88732=CARTESIAN_POINT('Ctrl Pts',(1.20290037631102E-14,54.8500000000093,
195.717944947196));
#88733=CARTESIAN_POINT('',(123.142835173977,54.8703625774417,193.770443909236));
#88734=CARTESIAN_POINT('Ctrl Pts',(123.142835173977,54.8703625774417,193.770443909236));
#88735=CARTESIAN_POINT('Ctrl Pts',(121.899340181671,54.863377344104,193.863435857888));
#88736=CARTESIAN_POINT('Ctrl Pts',(120.654374052645,54.8500000000005,193.934853431518));
#88737=CARTESIAN_POINT('Ctrl Pts',(119.410687750229,54.85,194.025969999953));
#88738=CARTESIAN_POINT('',(127.218111007812,54.870362430323,193.399408941216));
#88739=CARTESIAN_POINT('Ctrl Pts',(127.218115807736,54.8703459680316,193.399454348143));
#88740=CARTESIAN_POINT('Ctrl Pts',(126.904655624744,54.8721034990734,193.433239035163));
#88741=CARTESIAN_POINT('Ctrl Pts',(126.589462087755,54.8733936915971,193.465799923233));
#88742=CARTESIAN_POINT('Ctrl Pts',(126.069842054209,54.8748466726111,193.517494280518));
#88743=CARTESIAN_POINT('Ctrl Pts',(125.863371183883,54.8752481439835,193.53751566446));
#88744=CARTESIAN_POINT('Ctrl Pts',(125.565865345439,54.8755920729016,193.565665507521));
#88745=CARTESIAN_POINT('Ctrl Pts',(125.474374710482,54.8756657856571,193.574226747018));
#88746=CARTESIAN_POINT('Ctrl Pts',(125.315939112259,54.8757392663103,193.588890198462));
#88747=CARTESIAN_POINT('Ctrl Pts',(125.2489457798,54.8757535671162,193.595040325144));
#88748=CARTESIAN_POINT('Ctrl Pts',(125.113301273444,54.8757490110628,193.607392178321));
#88749=CARTESIAN_POINT('Ctrl Pts',(125.044551562222,54.8757293328324,193.613600376908));
#88750=CARTESIAN_POINT('Ctrl Pts',(124.876641589548,54.8756381943028,193.628634589557));
#88751=CARTESIAN_POINT('Ctrl Pts',(124.777384795725,54.8755475890981,193.63741238751));
#88752=CARTESIAN_POINT('Ctrl Pts',(124.429631300409,54.87509793653,193.667777337326));
#88753=CARTESIAN_POINT('Ctrl Pts',(124.18023801191,54.8745385967918,193.688857592025));
#88754=CARTESIAN_POINT('Ctrl Pts',(123.669067795424,54.8728573299448,193.730536953319));
#88755=CARTESIAN_POINT('Ctrl Pts',(123.405543514086,54.8716993004467,193.751193535519));
#88756=CARTESIAN_POINT('Ctrl Pts',(123.14286640231,54.8702154555249,193.770850279654));
#88757=CARTESIAN_POINT('',(130.93851195015,54.8499999998387,192.9690053296));
#88758=CARTESIAN_POINT('Ctrl Pts',(130.938511950113,54.85,192.969005329269));
#88759=CARTESIAN_POINT('Ctrl Pts',(130.748438209165,54.8499991196594,192.990502729015));
#88760=CARTESIAN_POINT('Ctrl Pts',(130.558419310946,54.8503671322184,193.012402086984));
#88761=CARTESIAN_POINT('Ctrl Pts',(130.368421134895,54.8509960128742,193.034550306987));
#88762=CARTESIAN_POINT('Ctrl Pts',(130.248410110378,54.8513932409601,193.048540075883));
#88763=CARTESIAN_POINT('Ctrl Pts',(130.128408438622,54.8518944712188,193.062628779303));
#88764=CARTESIAN_POINT('Ctrl Pts',(130.008417669627,54.8524737295353,193.076774905918));
#88765=CARTESIAN_POINT('Ctrl Pts',(129.89218384073,54.8530348511332,193.090478113876));
#88766=CARTESIAN_POINT('Ctrl Pts',(129.775956712028,54.8536688413448,193.104236291091));
#88767=CARTESIAN_POINT('Ctrl Pts',(129.659732098805,54.8543528373223,193.118014480271));
#88768=CARTESIAN_POINT('Ctrl Pts',(129.60888383052,54.8546520855624,193.124042438037));
#88769=CARTESIAN_POINT('Ctrl Pts',(129.558036045364,54.8549609249045,193.130074240602));
#88770=CARTESIAN_POINT('Ctrl Pts',(129.507188402119,54.8552775416311,193.136107031175));
#88771=CARTESIAN_POINT('Ctrl Pts',(129.365399712784,54.8561604275981,193.152929471974));
#88772=CARTESIAN_POINT('Ctrl Pts',(129.223606656697,54.8571005169143,193.16976679798));
#88773=CARTESIAN_POINT('Ctrl Pts',(129.081819468307,54.8580660163222,193.18654630739));
#88774=CARTESIAN_POINT('Ctrl Pts',(128.857087329936,54.8595963291029,193.213141764098));
#88775=CARTESIAN_POINT('Ctrl Pts',(128.632345894176,54.8611886270791,193.23958486306));
#88776=CARTESIAN_POINT('Ctrl Pts',(128.407552504352,54.8627477135206,193.265688218895));
#88777=CARTESIAN_POINT('Ctrl Pts',(128.166437604382,54.8644200001108,193.293686853711));
#88778=CARTESIAN_POINT('Ctrl Pts',(127.925263358931,54.8660541928077,193.321294884794));
#88779=CARTESIAN_POINT('Ctrl Pts',(127.684011178606,54.867575440588,193.348250932464));
#88780=CARTESIAN_POINT('Ctrl Pts',(127.528742633054,54.8685545070983,193.365599693042));
#88781=CARTESIAN_POINT('Ctrl Pts',(127.3734424732,54.8694876782735,193.382677751082));
#88782=CARTESIAN_POINT('Ctrl Pts',(127.218111007812,54.870362430323,193.399408941216));
#88783=CARTESIAN_POINT('',(190.217744333281,54.85,102.334299700915));
#88784=CARTESIAN_POINT('Ctrl Pts',(190.217744333281,54.85,102.334299700915));
#88785=CARTESIAN_POINT('Ctrl Pts',(190.198438372667,54.8500000000001,107.588457360702));
#88786=CARTESIAN_POINT('Ctrl Pts',(190.154899230013,54.85,112.84243630191));
#88787=CARTESIAN_POINT('Ctrl Pts',(189.981234566109,54.8499999999999,120.721692135521));
#88788=CARTESIAN_POINT('Ctrl Pts',(189.90484649384,54.85,123.347975843259));
#88789=CARTESIAN_POINT('Ctrl Pts',(189.695312595311,54.85,128.595739803922));
#88790=CARTESIAN_POINT('Ctrl Pts',(189.562294604773,54.85,131.217600991548));
#88791=CARTESIAN_POINT('Ctrl Pts',(189.210995417379,54.85,136.455224502561));
#88792=CARTESIAN_POINT('Ctrl Pts',(188.992951237667,54.85,139.071003779748));
#88793=CARTESIAN_POINT('Ctrl Pts',(188.428934412368,54.85,144.293411630326));
#88794=CARTESIAN_POINT('Ctrl Pts',(188.082255525325,54.85,146.905440395189));
#88795=CARTESIAN_POINT('Ctrl Pts',(187.202193126973,54.85,152.075325431284));
#88796=CARTESIAN_POINT('Ctrl Pts',(186.669269532277,54.85,154.635271282323));
#88797=CARTESIAN_POINT('Ctrl Pts',(185.327632557779,54.85,159.680949962078));
#88798=CARTESIAN_POINT('Ctrl Pts',(184.519597931304,54.8499999999999,162.16686543837));
#88799=CARTESIAN_POINT('Ctrl Pts',(182.999398653294,54.85,165.812818448613));
#88800=CARTESIAN_POINT('Ctrl Pts',(182.437877250581,54.85,167.018905464543));
#88801=CARTESIAN_POINT('Ctrl Pts',(181.213923690437,54.85,169.351657826097));
#88802=CARTESIAN_POINT('Ctrl Pts',(180.550121170522,54.85,170.48259474114));
#88803=CARTESIAN_POINT('Ctrl Pts',(179.10880585684,54.85,172.666711676218));
#88804=CARTESIAN_POINT('Ctrl Pts',(178.331265907326,54.85,173.71987312672));
#88805=CARTESIAN_POINT('Ctrl Pts',(177.073364034008,54.85,175.23698326999));
#88806=CARTESIAN_POINT('Ctrl Pts',(176.638813994407,54.85,175.732258858291));
#88807=CARTESIAN_POINT('Ctrl Pts',(175.738392615775,54.85,176.701392031852));
#88808=CARTESIAN_POINT('Ctrl Pts',(175.271411249757,54.85,177.176171676685));
#88809=CARTESIAN_POINT('Ctrl Pts',(172.887512343756,54.8500000000001,179.467132277965));
#88810=CARTESIAN_POINT('Ctrl Pts',(170.80436878542,54.85,181.056284046568));
#88811=CARTESIAN_POINT('Ctrl Pts',(167.464200921113,54.85,183.141826753163));
#88812=CARTESIAN_POINT('Ctrl Pts',(166.313975611903,54.85,183.787918097031));
#88813=CARTESIAN_POINT('Ctrl Pts',(163.954209381834,54.8499999999999,184.990236396472));
#88814=CARTESIAN_POINT('Ctrl Pts',(162.757917664203,54.85,185.540014896745));
#88815=CARTESIAN_POINT('Ctrl Pts',(159.128777137195,54.85,187.063266469322));
#88816=CARTESIAN_POINT('Ctrl Pts',(156.656109556117,54.85,187.912054070198));
#88817=CARTESIAN_POINT('Ctrl Pts',(151.638015130561,54.85,189.38179645165));
#88818=CARTESIAN_POINT('Ctrl Pts',(149.092379741324,54.85,190.002098211036));
#88819=CARTESIAN_POINT('Ctrl Pts',(145.235296685317,54.8499999999999,190.811587895128));
#88820=CARTESIAN_POINT('Ctrl Pts',(143.942303135459,54.85,191.061144118388));
#88821=CARTESIAN_POINT('Ctrl Pts',(141.353031978865,54.8499999999999,191.524375610374));
#88822=CARTESIAN_POINT('Ctrl Pts',(140.055900136512,54.85,191.738245937891));
#88823=CARTESIAN_POINT('Ctrl Pts',(136.158198163361,54.85,192.33502571568));
#88824=CARTESIAN_POINT('Ctrl Pts',(133.551375018438,54.8499999999999,192.673483797853));
#88825=CARTESIAN_POINT('Ctrl Pts',(130.938511950113,54.8499999999999,192.969005329269));
#88826=CARTESIAN_POINT('Origin',(189.999800857363,55.3,102.333498885935));
#88827=CARTESIAN_POINT('Origin',(1.20290037631083E-14,55.3,195.5));
#88828=CARTESIAN_POINT('Ctrl Pts',(-190.217744333281,54.85,102.334299700914));
#88829=CARTESIAN_POINT('Ctrl Pts',(-190.499797482064,54.9866054968633,102.335336081498));
#88830=CARTESIAN_POINT('Ctrl Pts',(-190.499797482064,55.2999999999999,102.335336081498));
#88831=CARTESIAN_POINT('Ctrl Pts',(-190.197958800231,54.8499999999032,107.718974084326));
#88832=CARTESIAN_POINT('Ctrl Pts',(-190.480008298463,54.9866054967246,107.721003970568));
#88833=CARTESIAN_POINT('Ctrl Pts',(-190.480008298168,55.3000000002241,107.72100397055));
#88834=CARTESIAN_POINT('Ctrl Pts',(-190.15286634701,54.8499999999749,113.103225357617));
#88835=CARTESIAN_POINT('Ctrl Pts',(-190.434912437381,54.9866054968165,113.106828120184));
#88836=CARTESIAN_POINT('Ctrl Pts',(-190.434912437369,55.3,113.106828120207));
#88837=CARTESIAN_POINT('Ctrl Pts',(-189.969140380158,54.8500000000125,121.176659053989));
#88838=CARTESIAN_POINT('Ctrl Pts',(-190.251090404902,54.9866054968868,121.184483209885));
#88839=CARTESIAN_POINT('Ctrl Pts',(-190.251090404908,55.3,121.184483209874));
#88840=CARTESIAN_POINT('Ctrl Pts',(-189.888083875663,54.8500000000125,123.867306750675));
#88841=CARTESIAN_POINT('Ctrl Pts',(-190.169985811631,54.9866054968868,123.876850850686));
#88842=CARTESIAN_POINT('Ctrl Pts',(-190.16998581157,55.2999999999999,123.876850850684));
#88843=CARTESIAN_POINT('Ctrl Pts',(-189.66437067227,54.8499999999874,129.247010167646));
#88844=CARTESIAN_POINT('Ctrl Pts',(-189.946091720074,54.98660549684,129.260904144669));
#88845=CARTESIAN_POINT('Ctrl Pts',(-189.946091720136,55.2999999999999,129.260904144672));
#88846=CARTESIAN_POINT('Ctrl Pts',(-189.52188207134,54.8500000000226,131.936069993364));
#88847=CARTESIAN_POINT('Ctrl Pts',(-189.803472315591,54.9866054969124,131.952591176849));
#88848=CARTESIAN_POINT('Ctrl Pts',(-189.803472315518,55.3000000000373,131.952591176844));
#88849=CARTESIAN_POINT('Ctrl Pts',(-189.143122039148,54.8499999999774,137.311741597895));
#88850=CARTESIAN_POINT('Ctrl Pts',(-189.424246871058,54.9866054968143,137.334868293955));
#88851=CARTESIAN_POINT('Ctrl Pts',(-189.424246871131,55.2999999999626,137.33486829396));
#88852=CARTESIAN_POINT('Ctrl Pts',(-188.906813700382,54.849999999973,140.001224223251));
#88853=CARTESIAN_POINT('Ctrl Pts',(-189.18760824081,54.9866054968095,140.028330517394));
#88854=CARTESIAN_POINT('Ctrl Pts',(-189.187608240719,55.2999999999813,140.028330517384));
#88855=CARTESIAN_POINT('Ctrl Pts',(-188.292632756423,54.850000000027,145.362689351932));
#88856=CARTESIAN_POINT('Ctrl Pts',(-188.572283011556,54.9866054969172,145.399784634254));
#88857=CARTESIAN_POINT('Ctrl Pts',(-188.572283011647,55.3000000000187,145.399784634264));
#88858=CARTESIAN_POINT('Ctrl Pts',(-187.915655912286,54.8500000000144,148.031000011928));
#88859=CARTESIAN_POINT('Ctrl Pts',(-188.194503693629,54.9866054968937,148.07409498288));
#88860=CARTESIAN_POINT('Ctrl Pts',(-188.194503693513,55.3000000000186,148.074094982859));
#88861=CARTESIAN_POINT('Ctrl Pts',(-186.949354871226,54.8499999999856,153.329908463642));
#88862=CARTESIAN_POINT('Ctrl Pts',(-187.225465197805,54.986605496833,153.388014825406));
#88863=CARTESIAN_POINT('Ctrl Pts',(-187.225465197921,55.2999999999813,153.388014825428));
#88864=CARTESIAN_POINT('Ctrl Pts',(-186.360811154485,54.8500000000352,155.960659886914));
#88865=CARTESIAN_POINT('Ctrl Pts',(-186.635007346912,54.9866054969361,156.027789475615));
#88866=CARTESIAN_POINT('Ctrl Pts',(-186.635007346693,55.3000000000374,156.027789475552));
#88867=CARTESIAN_POINT('Ctrl Pts',(-185.233316992153,54.8499999999824,159.8632205481));
#88868=CARTESIAN_POINT('Ctrl Pts',(-185.502677893398,54.986605496827,159.947086381085));
#88869=CARTESIAN_POINT('Ctrl Pts',(-185.502677893508,55.2999999999813,159.947086381116));
#88870=CARTESIAN_POINT('Ctrl Pts',(-184.815825918778,54.8500000000041,161.156850396224));
#88871=CARTESIAN_POINT('Ctrl Pts',(-185.083234340623,54.9866054968727,161.246835918567));
#88872=CARTESIAN_POINT('Ctrl Pts',(-185.083234340539,55.3000000000093,161.246835918536));
#88873=CARTESIAN_POINT('Ctrl Pts',(-183.890842670928,54.8499999999959,163.694223718077));
#88874=CARTESIAN_POINT('Ctrl Pts',(-184.153426616934,54.986605496854,163.797443530319));
#88875=CARTESIAN_POINT('Ctrl Pts',(-184.153426617017,55.2999999999906,163.79744353035));
#88876=CARTESIAN_POINT('Ctrl Pts',(-183.382385037553,54.8500000000062,164.94156139573));
#88877=CARTESIAN_POINT('Ctrl Pts',(-183.642091434846,54.986605496875,165.051912885639));
#88878=CARTESIAN_POINT('Ctrl Pts',(-183.642091434722,55.3,165.051912885581));
#88879=CARTESIAN_POINT('Ctrl Pts',(-182.257242363085,54.8499999999937,167.38579265337));
#88880=CARTESIAN_POINT('Ctrl Pts',(-182.509961211219,54.9866054968517,167.511323717164));
#88881=CARTESIAN_POINT('Ctrl Pts',(-182.509961211343,55.3,167.511323717221));
#88882=CARTESIAN_POINT('Ctrl Pts',(-181.640539237098,54.8500000000066,168.58268067929));
#88883=CARTESIAN_POINT('Ctrl Pts',(-181.889144137789,54.9866054968791,168.716261729528));
#88884=CARTESIAN_POINT('Ctrl Pts',(-181.889144137688,55.3000000000186,168.71626172947));
#88885=CARTESIAN_POINT('Ctrl Pts',(-180.620975247538,54.8499999999967,170.333700945188));
#88886=CARTESIAN_POINT('Ctrl Pts',(-180.862291929361,54.9866054968555,170.479798933249));
#88887=CARTESIAN_POINT('Ctrl Pts',(-180.862291929412,55.2999999999906,170.479798933278));
#88888=CARTESIAN_POINT('Ctrl Pts',(-180.26535921273,54.8500000000008,170.90998258945));
#88889=CARTESIAN_POINT('Ctrl Pts',(-180.504061049894,54.9866054968648,171.06032459263));
#88890=CARTESIAN_POINT('Ctrl Pts',(-180.504061049845,55.3,171.060324592604));
#88891=CARTESIAN_POINT('Ctrl Pts',(-179.520306450127,54.8499999999992,172.046622354047));
#88892=CARTESIAN_POINT('Ctrl Pts',(-179.75339270956,54.9866054968619,172.205531386762));
#88893=CARTESIAN_POINT('Ctrl Pts',(-179.753392709609,55.3,172.205531386788));
#88894=CARTESIAN_POINT('Ctrl Pts',(-179.129400936759,54.8499999999992,172.608873025932));
#88895=CARTESIAN_POINT('Ctrl Pts',(-179.359474666008,54.9866054968619,172.772119981196));
#88896=CARTESIAN_POINT('Ctrl Pts',(-179.359474666011,55.3,172.772119981188));
#88897=CARTESIAN_POINT('Ctrl Pts',(-177.107977365711,54.8500000000031,175.346620158582));
#88898=CARTESIAN_POINT('Ctrl Pts',(-177.322213675783,54.9866054968692,175.53131677416));
#88899=CARTESIAN_POINT('Ctrl Pts',(-177.322213675773,55.3,175.531316774194));
#88900=CARTESIAN_POINT('Ctrl Pts',(-175.273059695142,54.8500000000093,177.307053577842));
#88901=CARTESIAN_POINT('Ctrl Pts',(-175.472027446834,54.9866054968808,177.508051660724));
#88902=CARTESIAN_POINT('Ctrl Pts',(-175.472027446897,55.3,177.508051660799));
#88903=CARTESIAN_POINT('Ctrl Pts',(-172.213531513844,54.8499999999953,179.919041531276));
#88904=CARTESIAN_POINT('Ctrl Pts',(-172.388751139953,54.9866054968547,180.140313922478));
#88905=CARTESIAN_POINT('Ctrl Pts',(-172.388751139921,55.3,180.140313922441));
#88906=CARTESIAN_POINT('Ctrl Pts',(-171.14287675774,54.8500000000066,180.735334590373));
#88907=CARTESIAN_POINT('Ctrl Pts',(-171.310063503819,54.9866054968792,180.962699537817));
#88908=CARTESIAN_POINT('Ctrl Pts',(-171.310063503861,55.3000000000187,180.96269953789));
#88909=CARTESIAN_POINT('Ctrl Pts',(-169.465738000691,54.8499999999967,181.883222248313));
#88910=CARTESIAN_POINT('Ctrl Pts',(-169.621105252464,54.9866054968555,182.11867683742));
#88911=CARTESIAN_POINT('Ctrl Pts',(-169.621105252443,55.2999999999906,182.118676837383));
#88912=CARTESIAN_POINT('Ctrl Pts',(-168.893167994943,54.85,182.254113120666));
#88913=CARTESIAN_POINT('Ctrl Pts',(-169.04462193827,54.9866054968634,182.492098102623));
#88914=CARTESIAN_POINT('Ctrl Pts',(-169.04462193831,55.3,182.492098102688));
#88915=CARTESIAN_POINT('Ctrl Pts',(-167.734522038227,54.85,182.965862918278));
#88916=CARTESIAN_POINT('Ctrl Pts',(-167.87833659147,54.9866054968634,183.208540735198));
#88917=CARTESIAN_POINT('Ctrl Pts',(-167.87833659143,55.3,183.208540735133));
#88918=CARTESIAN_POINT('Ctrl Pts',(-167.149001871247,54.8499999999969,183.306536007332));
#88919=CARTESIAN_POINT('Ctrl Pts',(-167.289093057181,54.9866054968575,183.551375891323));
#88920=CARTESIAN_POINT('Ctrl Pts',(-167.289093057217,55.3,183.551375891388));
#88921=CARTESIAN_POINT('Ctrl Pts',(-164.193287616351,54.8500000000125,184.940751128666));
#88922=CARTESIAN_POINT('Ctrl Pts',(-164.315307422436,54.9866054968868,185.195582682745));
#88923=CARTESIAN_POINT('Ctrl Pts',(-164.315307422292,55.3,185.195582682486));
#88924=CARTESIAN_POINT('Ctrl Pts',(-161.739738382499,54.85,186.029085306811));
#88925=CARTESIAN_POINT('Ctrl Pts',(-161.84912521402,54.9866054968633,186.289321051958));
#88926=CARTESIAN_POINT('Ctrl Pts',(-161.849125214096,55.2999999999999,186.289321052161));
#88927=CARTESIAN_POINT('Ctrl Pts',(-157.968227272373,54.85,187.435958843901));
#88928=CARTESIAN_POINT('Ctrl Pts',(-158.061401990388,54.9866054968633,187.702242136645));
#88929=CARTESIAN_POINT('Ctrl Pts',(-158.06140199035,55.2999999999999,187.702242136544));
#88930=CARTESIAN_POINT('Ctrl Pts',(-156.695660864883,54.8500000000162,187.866859457223));
#88931=CARTESIAN_POINT('Ctrl Pts',(-156.783872375767,54.9866054969007,188.134808550894));
#88932=CARTESIAN_POINT('Ctrl Pts',(-156.783872375788,55.3000000000372,188.134808550961));
#88933=CARTESIAN_POINT('Ctrl Pts',(-154.124815734453,54.8499999999838,188.665095072689));
#88934=CARTESIAN_POINT('Ctrl Pts',(-154.203880012405,54.9866054968261,188.935884340155));
#88935=CARTESIAN_POINT('Ctrl Pts',(-154.203880012384,55.2999999999627,188.935884340088));
#88936=CARTESIAN_POINT('Ctrl Pts',(-152.824031066258,54.8500000000135,189.033044232236));
#88937=CARTESIAN_POINT('Ctrl Pts',(-152.898903324984,54.9866054968902,189.305009231248));
#88938=CARTESIAN_POINT('Ctrl Pts',(-152.898903325004,55.3000000000093,189.305009231326));
#88939=CARTESIAN_POINT('Ctrl Pts',(-148.908007282254,54.849999999973,190.052058242771));
#88940=CARTESIAN_POINT('Ctrl Pts',(-148.971352624573,54.9866054968096,190.32702273555));
#88941=CARTESIAN_POINT('Ctrl Pts',(-148.971352624532,55.2999999999813,190.327022735394));
#88942=CARTESIAN_POINT('Ctrl Pts',(-146.287439493149,54.8499999999776,190.618021136898));
#88943=CARTESIAN_POINT('Ctrl Pts',(-146.344500438236,54.9866054968147,190.894297995684));
#88944=CARTESIAN_POINT('Ctrl Pts',(-146.344500438254,55.2999999999629,190.894297995781));
#88945=CARTESIAN_POINT('Ctrl Pts',(-141.032967318856,54.8500000000224,191.597641496055));
#88946=CARTESIAN_POINT('Ctrl Pts',(-141.079295090532,54.986605496912,191.875919399702));
#88947=CARTESIAN_POINT('Ctrl Pts',(-141.079295090514,55.300000000037,191.875919399605));
#88948=CARTESIAN_POINT('Ctrl Pts',(-138.399009626471,54.8500000000471,192.010708935057));
#88949=CARTESIAN_POINT('Ctrl Pts',(-138.440892704756,54.9866054969581,192.289663795972));
#88950=CARTESIAN_POINT('Ctrl Pts',(-138.44089270476,55.3000000000369,192.289663796002));
#88951=CARTESIAN_POINT('Ctrl Pts',(-133.121607451461,54.8499999999529,192.729240056066));
#88952=CARTESIAN_POINT('Ctrl Pts',(-133.155827195463,54.9866054967686,193.009238298489));
#88953=CARTESIAN_POINT('Ctrl Pts',(-133.155827195459,55.2999999999631,193.009238298459));
#88954=CARTESIAN_POINT('Ctrl Pts',(-130.47813816516,54.849999999992,193.034416151033));
#88955=CARTESIAN_POINT('Ctrl Pts',(-130.509142871666,54.9866054968449,193.314776001578));
#88956=CARTESIAN_POINT('Ctrl Pts',(-130.509142871667,55.2999999999815,193.31477600159));
#88957=CARTESIAN_POINT('Ctrl Pts',(-122.537325370419,54.8500000000161,193.832649170543));
#88958=CARTESIAN_POINT('Ctrl Pts',(-122.559948354902,54.9866054969003,194.11385157553));
#88959=CARTESIAN_POINT('Ctrl Pts',(-122.559948354899,55.3000000000369,194.113851575506));
#88960=CARTESIAN_POINT('Ctrl Pts',(-117.229788845083,54.8499999999913,194.210877457251));
#88961=CARTESIAN_POINT('Ctrl Pts',(-117.248473697759,54.986605496854,194.492330262601));
#88962=CARTESIAN_POINT('Ctrl Pts',(-117.248473697781,55.3000000000369,194.492330262574));
#88963=CARTESIAN_POINT('Ctrl Pts',(-106.599582434858,54.8500000000087,194.798457441269));
#88964=CARTESIAN_POINT('Ctrl Pts',(-106.612030995843,54.9866054968727,195.080254954912));
#88965=CARTESIAN_POINT('Ctrl Pts',(-106.612030995821,55.299999999963,195.08025495494));
#88966=CARTESIAN_POINT('Ctrl Pts',(-101.276765722829,54.85,195.006073597426));
#88967=CARTESIAN_POINT('Ctrl Pts',(-101.286942967898,54.9866054968634,195.287950777376));
#88968=CARTESIAN_POINT('Ctrl Pts',(-101.286942967899,55.3,195.28795077739));
#88969=CARTESIAN_POINT('Ctrl Pts',(-90.6222412308268,54.85,195.32239623046));
#88970=CARTESIAN_POINT('Ctrl Pts',(-90.6288044985487,54.9866054968634,195.604380705992));
#88971=CARTESIAN_POINT('Ctrl Pts',(-90.6288044985483,55.3,195.604380705979));
#88972=CARTESIAN_POINT('Ctrl Pts',(-85.2899196297656,54.849999999959,195.430398920617));
#88973=CARTESIAN_POINT('Ctrl Pts',(-85.2951502477932,54.98660549678,195.712407433009));
#88974=CARTESIAN_POINT('Ctrl Pts',(-85.295150247793,55.299999999963,195.712407432997));
#88975=CARTESIAN_POINT('Ctrl Pts',(-74.628059287452,54.8500000000409,195.588359025636));
#88976=CARTESIAN_POINT('Ctrl Pts',(-74.6311852892752,54.9866054969467,195.870398718805));
#88977=CARTESIAN_POINT('Ctrl Pts',(-74.6311852892754,55.3000000000369,195.870398718817));
#88978=CARTESIAN_POINT('Ctrl Pts',(-69.2972283472756,54.85,195.6380334407));
#88979=CARTESIAN_POINT('Ctrl Pts',(-69.2995860602678,54.9866054968634,195.920079260338));
#88980=CARTESIAN_POINT('Ctrl Pts',(-69.2995860602679,55.3,195.920079260345));
#88981=CARTESIAN_POINT('Ctrl Pts',(-53.3049437790784,54.85,195.73815589255));
#88982=CARTESIAN_POINT('Ctrl Pts',(-53.3055258119786,54.9866054968634,196.02021282908));
#88983=CARTESIAN_POINT('Ctrl Pts',(-53.3055258119785,55.3,196.020212829065));
#88984=CARTESIAN_POINT('Ctrl Pts',(-42.6436940741756,54.85,195.741936415933));
#88985=CARTESIAN_POINT('Ctrl Pts',(-42.6437804403081,54.9866054968634,196.023991532525));
#88986=CARTESIAN_POINT('Ctrl Pts',(-42.6437804403082,55.3,196.023991532478));
#88987=CARTESIAN_POINT('Ctrl Pts',(-21.3215695785207,54.85,195.732705751546));
#88988=CARTESIAN_POINT('Ctrl Pts',(-21.321239000773,54.9866054968634,196.014760687738));
#88989=CARTESIAN_POINT('Ctrl Pts',(-21.3212390007729,55.3,196.014760687785));
#88990=CARTESIAN_POINT('Ctrl Pts',(-10.6607012638122,54.8499999999627,195.71794494731));
#88991=CARTESIAN_POINT('Ctrl Pts',(-10.6604701165162,54.9866054967938,196.000000000093));
#88992=CARTESIAN_POINT('Ctrl Pts',(-10.6604701165162,55.3,196.));
#88993=CARTESIAN_POINT('Ctrl Pts',(1.20290037631083E-14,54.85,195.717944947177));
#88994=CARTESIAN_POINT('Ctrl Pts',(1.20290037631083E-14,54.9866054968634,
196.));
#88995=CARTESIAN_POINT('Ctrl Pts',(1.20290037631083E-14,55.3,196.));
#88996=CARTESIAN_POINT('',(-190.217744333281,54.85,102.334299700914));
#88997=CARTESIAN_POINT('Ctrl Pts',(8.09400652964437E-15,54.8500000000093,
195.717944947196));
#88998=CARTESIAN_POINT('Ctrl Pts',(-10.6608823663659,54.8499999999628,195.71794494731));
#88999=CARTESIAN_POINT('Ctrl Pts',(-21.3217703135716,54.8500173325644,195.732741622938));
#89000=CARTESIAN_POINT('Ctrl Pts',(-31.9826318183453,54.8500089537298,195.737339569908));
#89001=CARTESIAN_POINT('Ctrl Pts',(-32.0538745521929,54.850008897737,195.737370296347));
#89002=CARTESIAN_POINT('Ctrl Pts',(-32.1251172845683,54.8500088405961,195.737400645486));
#89003=CARTESIAN_POINT('Ctrl Pts',(-32.1963600154795,54.8500087822941,195.737430601013));
#89004=CARTESIAN_POINT('Ctrl Pts',(-42.7864993946942,54.8500001157824,195.741883451166));
#89005=CARTESIAN_POINT('Ctrl Pts',(-53.376605619207,54.8500178679623,195.737744132389));
#89006=CARTESIAN_POINT('Ctrl Pts',(-63.966466909668,54.8500065855881,195.671421188064));
#89007=CARTESIAN_POINT('Ctrl Pts',(-64.1084275988407,54.850006434344,195.670532106458));
#89008=CARTESIAN_POINT('Ctrl Pts',(-64.2503882446953,54.8500062778827,195.669631454805));
#89009=CARTESIAN_POINT('Ctrl Pts',(-64.3923488470745,54.8500061160708,195.668718987262));
#89010=CARTESIAN_POINT('Ctrl Pts',(-69.5813056237556,54.8500002015057,195.635366391111));
#89011=CARTESIAN_POINT('Ctrl Pts',(-74.7702705239252,54.8500177709199,195.586288797379));
#89012=CARTESIAN_POINT('Ctrl Pts',(-79.9589897750587,54.8500103466269,195.509400332601));
#89013=CARTESIAN_POINT('Ctrl Pts',(-80.1359326075558,54.8500100934478,195.506778324725));
#89014=CARTESIAN_POINT('Ctrl Pts',(-80.3128765776078,54.850009811204,195.504124288698));
#89015=CARTESIAN_POINT('Ctrl Pts',(-80.4898214380652,54.8500094979738,195.501437448281));
#89016=CARTESIAN_POINT('Ctrl Pts',(-84.2161548089894,54.8500029015686,195.444854493121));
#89017=CARTESIAN_POINT('Ctrl Pts',(-87.9419352769354,54.8500219794238,195.373821829301));
#89018=CARTESIAN_POINT('Ctrl Pts',(-91.6663092609427,54.8500269293056,195.281029095046));
#89019=CARTESIAN_POINT('Ctrl Pts',(-93.0942640584976,54.8500288271299,195.245451617964));
#89020=CARTESIAN_POINT('Ctrl Pts',(-94.5220120877842,54.8500286476275,195.20667493315));
#89021=CARTESIAN_POINT('Ctrl Pts',(-95.9495049562082,54.8500241474107,195.164284743112));
#89022=CARTESIAN_POINT('Ctrl Pts',(-96.160010222454,54.8500234837861,195.158033672835));
#89023=CARTESIAN_POINT('Ctrl Pts',(-96.3705108978206,54.8500227262081,195.151705119376));
#89024=CARTESIAN_POINT('Ctrl Pts',(-96.5810070229234,54.850021867489,195.145296789444));
#89025=CARTESIAN_POINT('Ctrl Pts',(-100.153755735135,54.8500072924569,195.036528266986));
#89026=CARTESIAN_POINT('Ctrl Pts',(-103.725065610368,54.8500509518181,194.904965551832));
#89027=CARTESIAN_POINT('Ctrl Pts',(-107.294222030251,54.8500655366034,194.739296744632));
#89028=CARTESIAN_POINT('Ctrl Pts',(-108.834799786133,54.8500718319273,194.667788060453));
#89029=CARTESIAN_POINT('Ctrl Pts',(-110.374976159483,54.8500727069131,194.589924501481));
#89030=CARTESIAN_POINT('Ctrl Pts',(-111.914692604448,54.8500611385557,194.50479344714));
#89031=CARTESIAN_POINT('Ctrl Pts',(-112.160365253972,54.8500592927425,194.491210185271));
#89032=CARTESIAN_POINT('Ctrl Pts',(-112.40602650628,54.8500571301813,194.477445607957));
#89033=CARTESIAN_POINT('Ctrl Pts',(-112.65167584228,54.8500546224071,194.46349276727));
#89034=CARTESIAN_POINT('Ctrl Pts',(-115.322724624506,54.8500273543214,194.311777648746));
#89035=CARTESIAN_POINT('Ctrl Pts',(-117.992372106993,54.8500268152894,194.137946722465));
#89036=CARTESIAN_POINT('Ctrl Pts',(-120.660060774621,54.8500287491632,193.933064820058));
#89037=CARTESIAN_POINT('Ctrl Pts',(-123.052153184648,54.8500304832505,193.749349062801));
#89038=CARTESIAN_POINT('Ctrl Pts',(-125.442670690351,54.8500342081856,193.540666594926));
#89039=CARTESIAN_POINT('Ctrl Pts',(-127.83120520213,54.8500224481125,193.300539935285));
#89040=CARTESIAN_POINT('Ctrl Pts',(-128.116308822552,54.8500210443901,193.271877598741));
#89041=CARTESIAN_POINT('Ctrl Pts',(-128.401383566503,54.8500194200674,193.242760058163));
#89042=CARTESIAN_POINT('Ctrl Pts',(-128.686428059558,54.8500175454592,193.213168377398));
#89043=CARTESIAN_POINT('Ctrl Pts',(-130.749050770458,54.8500039805263,192.999038744005));
#89044=CARTESIAN_POINT('Ctrl Pts',(-132.810104968374,54.850025848303,192.760185452714));
#89045=CARTESIAN_POINT('Ctrl Pts',(-134.869143324983,54.8500268298807,192.489305956972));
#89046=CARTESIAN_POINT('Ctrl Pts',(-135.166243246818,54.8500269715132,192.450220586486));
#89047=CARTESIAN_POINT('Ctrl Pts',(-135.463301170148,54.8500266782594,192.41046835331));
#89048=CARTESIAN_POINT('Ctrl Pts',(-135.760315719154,54.8500257809353,192.370027231952));
#89049=CARTESIAN_POINT('Ctrl Pts',(-136.067578585864,54.8500248526495,192.328190712754));
#89050=CARTESIAN_POINT('Ctrl Pts',(-136.374795369895,54.8500232778804,192.285620846307));
#89051=CARTESIAN_POINT('Ctrl Pts',(-136.681963465636,54.8500208694187,192.242280665229));
#89052=CARTESIAN_POINT('Ctrl Pts',(-137.619433940555,54.8500135188449,192.11000735722));
#89053=CARTESIAN_POINT('Ctrl Pts',(-138.556477977294,54.8500184166363,191.970592697317));
#89054=CARTESIAN_POINT('Ctrl Pts',(-139.49227471986,54.8500261469767,191.823104689008));
#89055=CARTESIAN_POINT('Ctrl Pts',(-140.361449919136,54.8500333269763,191.686116694519));
#89056=CARTESIAN_POINT('Ctrl Pts',(-141.229549084268,54.8500429514451,191.542163698025));
#89057=CARTESIAN_POINT('Ctrl Pts',(-142.095917433607,54.850047472919,191.390543532221));
#89058=CARTESIAN_POINT('Ctrl Pts',(-142.618028305764,54.8500501977539,191.299170691714));
#89059=CARTESIAN_POINT('Ctrl Pts',(-143.139510640945,54.8500510690445,191.20501418281));
#89060=CARTESIAN_POINT('Ctrl Pts',(-143.660221729556,54.8500484348223,191.107929600065));
#89061=CARTESIAN_POINT('Ctrl Pts',(-143.986659753988,54.8500467834069,191.047066484055));
#89062=CARTESIAN_POINT('Ctrl Pts',(-144.312795498642,54.850043754279,190.985061831075));
#89063=CARTESIAN_POINT('Ctrl Pts',(-144.638591532731,54.8500389409188,190.921854313299));
#89064=CARTESIAN_POINT('Ctrl Pts',(-145.864982398198,54.8500208220335,190.683922864423));
#89065=CARTESIAN_POINT('Ctrl Pts',(-147.086704129731,54.8500111358652,190.428986178105));
#89066=CARTESIAN_POINT('Ctrl Pts',(-148.303814497845,54.8500062423224,190.153475973731));
#89067=CARTESIAN_POINT('Ctrl Pts',(-149.379024500777,54.8500019193077,189.910086930786));
#89068=CARTESIAN_POINT('Ctrl Pts',(-150.45063586881,54.8500013371218,189.650643680963));
#89069=CARTESIAN_POINT('Ctrl Pts',(-151.518690840111,54.8500019909062,189.372719547259));
#89070=CARTESIAN_POINT('Ctrl Pts',(-151.840538674191,54.8500021879176,189.288969850029));
#89071=CARTESIAN_POINT('Ctrl Pts',(-152.161936727543,54.8500024971687,189.203546240927));
#89072=CARTESIAN_POINT('Ctrl Pts',(-152.482731128704,54.8500028501313,189.116409021106));
#89073=CARTESIAN_POINT('Ctrl Pts',(-153.059659884567,54.8500034849125,188.959698156955));
#89074=CARTESIAN_POINT('Ctrl Pts',(-153.635450160572,54.8500037883794,188.797226731405));
#89075=CARTESIAN_POINT('Ctrl Pts',(-154.209635529004,54.8500037516326,188.628574338648));
#89076=CARTESIAN_POINT('Ctrl Pts',(-154.610676144961,54.8500037259667,188.510778826619));
#89077=CARTESIAN_POINT('Ctrl Pts',(-155.010933537627,54.8500035343333,188.389967202185));
#89078=CARTESIAN_POINT('Ctrl Pts',(-155.41024024276,54.8500031737061,188.265983522997));
#89079=CARTESIAN_POINT('Ctrl Pts',(-155.722702261715,54.8500028915113,188.168964889905));
#89080=CARTESIAN_POINT('Ctrl Pts',(-156.034729938686,54.850002505833,188.069967506862));
#89081=CARTESIAN_POINT('Ctrl Pts',(-156.346359438258,54.850002015223,187.968862642223));
#89082=CARTESIAN_POINT('Ctrl Pts',(-156.829044177179,54.8500012553143,187.81226073111));
#89083=CARTESIAN_POINT('Ctrl Pts',(-157.310905250608,54.8500072780007,187.650569111632));
#89084=CARTESIAN_POINT('Ctrl Pts',(-157.791044491721,54.8500142606259,187.483641634521));
#89085=CARTESIAN_POINT('Ctrl Pts',(-158.236870292617,54.8500207442335,187.328643730158));
#89086=CARTESIAN_POINT('Ctrl Pts',(-158.681211585458,54.8500280556456,187.169131631849));
#89087=CARTESIAN_POINT('Ctrl Pts',(-159.123367174125,54.8500315308054,187.005034533807));
#89088=CARTESIAN_POINT('Ctrl Pts',(-159.157398132692,54.8500317982746,186.99240463228));
#89089=CARTESIAN_POINT('Ctrl Pts',(-159.191416152949,54.8500320430176,186.979747594348));
#89090=CARTESIAN_POINT('Ctrl Pts',(-159.225420919937,54.8500322629076,186.967063399997));
#89091=CARTESIAN_POINT('Ctrl Pts',(-159.535627988313,54.8500342688443,186.851352366136));
#89092=CARTESIAN_POINT('Ctrl Pts',(-159.844743764922,54.8500342064119,186.7334078408));
#89093=CARTESIAN_POINT('Ctrl Pts',(-160.152517177576,54.8500304615589,186.613187307355));
#89094=CARTESIAN_POINT('Ctrl Pts',(-160.837757657589,54.8500221238508,186.345522939161));
#89095=CARTESIAN_POINT('Ctrl Pts',(-161.516997750355,54.8500160688841,186.066368496853));
#89096=CARTESIAN_POINT('Ctrl Pts',(-162.189598467762,54.8500116711269,185.774498421334));
#89097=CARTESIAN_POINT('Ctrl Pts',(-162.851405567252,54.8500073439431,185.487312155979));
#89098=CARTESIAN_POINT('Ctrl Pts',(-163.506784615461,54.8500046212496,185.187814946701));
#89099=CARTESIAN_POINT('Ctrl Pts',(-164.155145741996,54.8500029079638,184.874885718999));
#89100=CARTESIAN_POINT('Ctrl Pts',(-164.790397041045,54.8500012293207,184.568283903634));
#89101=CARTESIAN_POINT('Ctrl Pts',(-165.418911321688,54.8500005197017,184.248787686258));
#89102=CARTESIAN_POINT('Ctrl Pts',(-166.040152646954,54.8500002197043,183.915389170481));
#89103=CARTESIAN_POINT('Ctrl Pts',(-166.213290015513,54.8500001360962,183.822472393449));
#89104=CARTESIAN_POINT('Ctrl Pts',(-166.385862599876,54.8500000843048,183.728476092638));
#89105=CARTESIAN_POINT('Ctrl Pts',(-166.55785907244,54.8500000522222,183.633379125962));
#89106=CARTESIAN_POINT('Ctrl Pts',(-166.837832170401,54.8499999999985,183.478581809656));
#89107=CARTESIAN_POINT('Ctrl Pts',(-167.116264884686,54.8499999999984,183.320836486654));
#89108=CARTESIAN_POINT('Ctrl Pts',(-167.393094984824,54.8499999999988,183.160022261953));
#89109=CARTESIAN_POINT('Ctrl Pts',(-167.685523875221,54.8499999999991,182.990146496039));
#89110=CARTESIAN_POINT('Ctrl Pts',(-167.975956522574,54.8499999999999,182.816972220691));
#89111=CARTESIAN_POINT('Ctrl Pts',(-168.264823575429,54.8500000866495,182.640056525926));
#89112=CARTESIAN_POINT('Ctrl Pts',(-168.281169085329,54.8500000915526,182.630045771111));
#89113=CARTESIAN_POINT('Ctrl Pts',(-168.297509577167,54.8500000967331,182.620023023886));
#89114=CARTESIAN_POINT('Ctrl Pts',(-168.313845127043,54.8500001022067,182.609988199285));
#89115=CARTESIAN_POINT('Ctrl Pts',(-168.602860109673,54.8500001990484,182.432448129943));
#89116=CARTESIAN_POINT('Ctrl Pts',(-168.890192672684,54.8500003876472,182.251177618191));
#89117=CARTESIAN_POINT('Ctrl Pts',(-169.175478680366,54.850000754949,182.066258513183));
#89118=CARTESIAN_POINT('Ctrl Pts',(-169.437780750684,54.8500010926593,181.896237331706));
#89119=CARTESIAN_POINT('Ctrl Pts',(-169.698353639928,54.8500015814379,181.723130682223));
#89120=CARTESIAN_POINT('Ctrl Pts',(-169.956876365831,54.8500022888712,181.546974119049));
#89121=CARTESIAN_POINT('Ctrl Pts',(-169.979529142198,54.8500023508592,181.531538589282));
#89122=CARTESIAN_POINT('Ctrl Pts',(-170.002166146793,54.8500024145262,181.516079628883));
#89123=CARTESIAN_POINT('Ctrl Pts',(-170.024787145037,54.8500024799174,181.500597254396));
#89124=CARTESIAN_POINT('Ctrl Pts',(-170.276030180198,54.8500032061933,181.32864026489));
#89125=CARTESIAN_POINT('Ctrl Pts',(-170.52563717389,54.8500041451709,181.153591409795));
#89126=CARTESIAN_POINT('Ctrl Pts',(-170.773852761769,54.8500053591626,180.975118583254));
#89127=CARTESIAN_POINT('Ctrl Pts',(-170.997400265556,54.8500064525057,180.814382687463));
#89128=CARTESIAN_POINT('Ctrl Pts',(-171.219836911137,54.8500072970219,180.65084691465));
#89129=CARTESIAN_POINT('Ctrl Pts',(-171.4405992899,54.8500076440165,180.484811934086));
#89130=CARTESIAN_POINT('Ctrl Pts',(-171.658857749817,54.8500079870754,180.320660146299));
#89131=CARTESIAN_POINT('Ctrl Pts',(-171.875479669646,54.8500078438299,180.154065488974));
#89132=CARTESIAN_POINT('Ctrl Pts',(-172.089955276584,54.8500069739881,179.985355854544));
#89133=CARTESIAN_POINT('Ctrl Pts',(-172.190228162052,54.8500065673145,179.906479743213));
#89134=CARTESIAN_POINT('Ctrl Pts',(-172.290032406048,54.8500060018222,179.827141877461));
#89135=CARTESIAN_POINT('Ctrl Pts',(-172.389318587393,54.8500052529633,179.747378636735));
#89136=CARTESIAN_POINT('Ctrl Pts',(-172.674702066623,54.8500031004787,179.518110969828));
#89137=CARTESIAN_POINT('Ctrl Pts',(-172.956068640285,54.8500017378943,179.285125620791));
#89138=CARTESIAN_POINT('Ctrl Pts',(-173.233384096643,54.8500073519304,179.048390424515));
#89139=CARTESIAN_POINT('Ctrl Pts',(-173.467638136679,54.8500120942215,178.848415360469));
#89140=CARTESIAN_POINT('Ctrl Pts',(-173.698981502201,54.8500218139805,178.645743109414));
#89141=CARTESIAN_POINT('Ctrl Pts',(-173.927415809643,54.8500402477035,178.440378355981));
#89142=CARTESIAN_POINT('Ctrl Pts',(-174.411601717874,54.8500793195445,178.005090326029));
#89143=CARTESIAN_POINT('Ctrl Pts',(-174.882407081437,54.8500970763827,177.557823667813));
#89144=CARTESIAN_POINT('Ctrl Pts',(-175.340006494809,54.8501017502797,177.098439362564));
#89145=CARTESIAN_POINT('Ctrl Pts',(-175.794576229559,54.8501063932317,176.642096553368));
#89146=CARTESIAN_POINT('Ctrl Pts',(-176.236114350063,54.850098130278,176.173796068497));
#89147=CARTESIAN_POINT('Ctrl Pts',(-176.664760320395,54.850085069284,175.693361571846));
#89148=CARTESIAN_POINT('Ctrl Pts',(-177.089022890663,54.8500721418538,175.217840072748));
#89149=CARTESIAN_POINT('Ctrl Pts',(-177.500655675424,54.8500545155468,174.730431470717));
#89150=CARTESIAN_POINT('Ctrl Pts',(-177.899762155142,54.8500400462237,174.230925044469));
#89151=CARTESIAN_POINT('Ctrl Pts',(-178.181106114092,54.8500298462974,173.878805691306));
#89152=CARTESIAN_POINT('Ctrl Pts',(-178.45622468802,54.8500212147052,173.520673709915));
#89153=CARTESIAN_POINT('Ctrl Pts',(-178.725144291181,54.8500168999681,173.156443177018));
#89154=CARTESIAN_POINT('Ctrl Pts',(-178.900331371547,54.8500140891421,172.919166002398));
#89155=CARTESIAN_POINT('Ctrl Pts',(-179.072930945669,54.8500131102433,172.679236747959));
#89156=CARTESIAN_POINT('Ctrl Pts',(-179.242558922419,54.8500147234712,172.437343705895));
#89157=CARTESIAN_POINT('Ctrl Pts',(-179.409540825703,54.8500163115338,172.199224019927));
#89158=CARTESIAN_POINT('Ctrl Pts',(-179.574369077232,54.8500137889583,171.958134845391));
#89159=CARTESIAN_POINT('Ctrl Pts',(-179.736323660477,54.8500104070973,171.715126362041));
#89160=CARTESIAN_POINT('Ctrl Pts',(-179.788806911429,54.8500093111662,171.636376659751));
#89161=CARTESIAN_POINT('Ctrl Pts',(-179.840988586092,54.8500081249988,171.557425766626));
#89162=CARTESIAN_POINT('Ctrl Pts',(-179.892844848329,54.8500069592319,171.478310348672));
#89163=CARTESIAN_POINT('Ctrl Pts',(-180.05189632116,54.850003383638,171.235650673513));
#89164=CARTESIAN_POINT('Ctrl Pts',(-180.208151077888,54.8499999999998,170.991096913461));
#89165=CARTESIAN_POINT('Ctrl Pts',(-180.361429505763,54.8499999999993,170.745090323767));
#89166=CARTESIAN_POINT('Ctrl Pts',(-180.566661136845,54.8499999999987,170.415700634953));
#89167=CARTESIAN_POINT('Ctrl Pts',(-180.766380808872,54.8500000984341,170.083978833131));
#89168=CARTESIAN_POINT('Ctrl Pts',(-180.96083020235,54.8500001634391,169.750027693026));
#89169=CARTESIAN_POINT('Ctrl Pts',(-181.105064833824,54.8500002116571,169.50231635404));
#89170=CARTESIAN_POINT('Ctrl Pts',(-181.24640142172,54.8500002414793,169.253379552386));
#89171=CARTESIAN_POINT('Ctrl Pts',(-181.384934465216,54.8500001990872,169.003256361499));
#89172=CARTESIAN_POINT('Ctrl Pts',(-181.776611235903,54.8500000792315,168.296078916981));
#89173=CARTESIAN_POINT('Ctrl Pts',(-182.145884496243,54.8500012930554,167.579420745079));
#89174=CARTESIAN_POINT('Ctrl Pts',(-182.494841975545,54.8500020250206,166.854169935699));
#89175=CARTESIAN_POINT('Ctrl Pts',(-182.605177175342,54.8500022564572,166.624856343923));
#89176=CARTESIAN_POINT('Ctrl Pts',(-182.713480983087,54.8500024397198,166.394683554933));
#89177=CARTESIAN_POINT('Ctrl Pts',(-182.819818421831,54.8500025174166,166.163679197984));
#89178=CARTESIAN_POINT('Ctrl Pts',(-182.935798630709,54.850002602159,165.911727167849));
#89179=CARTESIAN_POINT('Ctrl Pts',(-183.049440450245,54.8500025613201,165.658786155025));
#89180=CARTESIAN_POINT('Ctrl Pts',(-183.160821296697,54.8500023204387,165.404887883679));
#89181=CARTESIAN_POINT('Ctrl Pts',(-183.365125754767,54.8500018785932,164.939165541063));
#89182=CARTESIAN_POINT('Ctrl Pts',(-183.561639829366,54.8500055588454,164.470674968065));
#89183=CARTESIAN_POINT('Ctrl Pts',(-183.750988391072,54.8500111929849,163.999314478622));
#89184=CARTESIAN_POINT('Ctrl Pts',(-183.947592530409,54.850017043017,163.509892100606));
#89185=CARTESIAN_POINT('Ctrl Pts',(-184.136471310677,54.8500249997458,163.017375565003));
#89186=CARTESIAN_POINT('Ctrl Pts',(-184.318273619788,54.8500326353226,162.521628197236));
#89187=CARTESIAN_POINT('Ctrl Pts',(-184.330012024327,54.8500331283278,162.489619345532));
#89188=CARTESIAN_POINT('Ctrl Pts',(-184.341720911643,54.8500336199935,162.457597017546));
#89189=CARTESIAN_POINT('Ctrl Pts',(-184.353400449796,54.8500341096657,162.425561173513));
#89190=CARTESIAN_POINT('Ctrl Pts',(-184.543743154348,54.8500420899082,161.903469536315));
#89191=CARTESIAN_POINT('Ctrl Pts',(-184.726458531671,54.8500495408636,161.377181095366));
#89192=CARTESIAN_POINT('Ctrl Pts',(-184.901911923505,54.8500536313765,160.847476946169));
#89193=CARTESIAN_POINT('Ctrl Pts',(-185.083025533198,54.8500578538514,160.300684265064));
#89194=CARTESIAN_POINT('Ctrl Pts',(-185.256401042875,54.8500584951217,159.750250429398));
#89195=CARTESIAN_POINT('Ctrl Pts',(-185.422386623896,54.8500524422723,159.197025985645));
#89196=CARTESIAN_POINT('Ctrl Pts',(-185.48573987968,54.8500501320251,158.985871682508));
#89197=CARTESIAN_POINT('Ctrl Pts',(-185.548016034937,54.8500468466359,158.774310881095));
#89198=CARTESIAN_POINT('Ctrl Pts',(-185.60923249047,54.8500424133448,158.562391294959));
#89199=CARTESIAN_POINT('Ctrl Pts',(-185.679701723209,54.8500373099683,158.318440375111));
#89200=CARTESIAN_POINT('Ctrl Pts',(-185.748797650257,54.8500306854296,158.074012769126));
#89201=CARTESIAN_POINT('Ctrl Pts',(-185.816571022676,54.8500222767591,157.829073160196));
#89202=CARTESIAN_POINT('Ctrl Pts',(-185.918406796886,54.8500096419523,157.461028693464));
#89203=CARTESIAN_POINT('Ctrl Pts',(-186.017319103435,54.8500041741207,157.091670527571));
#89204=CARTESIAN_POINT('Ctrl Pts',(-186.113234906169,54.8500018069331,156.721804640251));
#89205=CARTESIAN_POINT('Ctrl Pts',(-186.186449970179,54.8499999999964,156.439476245519));
#89206=CARTESIAN_POINT('Ctrl Pts',(-186.257920283618,54.8500000000129,156.156852248164));
#89207=CARTESIAN_POINT('Ctrl Pts',(-186.327633325725,54.8500000000123,155.874294898771));
#89208=CARTESIAN_POINT('Ctrl Pts',(-186.488674327249,54.8500000000109,155.221571718727));
#89209=CARTESIAN_POINT('Ctrl Pts',(-186.640602570786,54.8500000000075,154.568170282113));
#89210=CARTESIAN_POINT('Ctrl Pts',(-186.784395313844,54.8500000000042,153.914165865284));
#89211=CARTESIAN_POINT('Ctrl Pts',(-186.967585480598,54.8500000000001,153.080972370057));
#89212=CARTESIAN_POINT('Ctrl Pts',(-187.137593562521,54.8500103689392,152.246804668101));
#89213=CARTESIAN_POINT('Ctrl Pts',(-187.296351738213,54.8500156959195,151.411830799846));
#89214=CARTESIAN_POINT('Ctrl Pts',(-187.342692041962,54.8500172508245,151.168108279678));
#89215=CARTESIAN_POINT('Ctrl Pts',(-187.388073498977,54.8500183760775,150.924317036446));
#89216=CARTESIAN_POINT('Ctrl Pts',(-187.43254334808,54.8500186882901,150.680461159443));
#89217=CARTESIAN_POINT('Ctrl Pts',(-187.474893892218,54.8500189856236,150.448226751392));
#89218=CARTESIAN_POINT('Ctrl Pts',(-187.516411642212,54.850018545554,150.21593254165));
#89219=CARTESIAN_POINT('Ctrl Pts',(-187.557122720677,54.8500170370286,149.983579406153));
#89220=CARTESIAN_POINT('Ctrl Pts',(-187.723025465295,54.8500108895986,149.036711272131));
#89221=CARTESIAN_POINT('Ctrl Pts',(-187.87557598185,54.850011114299,148.08892712507));
#89222=CARTESIAN_POINT('Ctrl Pts',(-188.016548444847,54.8500131636224,147.140288699541));
#89223=CARTESIAN_POINT('Ctrl Pts',(-188.165405941458,54.8500153275708,146.138589940715));
#89224=CARTESIAN_POINT('Ctrl Pts',(-188.301353764444,54.8500195263539,145.135938648905));
#89225=CARTESIAN_POINT('Ctrl Pts',(-188.426422471049,54.8500204062576,144.132398367695));
#89226=CARTESIAN_POINT('Ctrl Pts',(-188.486651809581,54.8500208299929,143.649123462496));
#89227=CARTESIAN_POINT('Ctrl Pts',(-188.544357357385,54.8500204840077,143.165642262192));
#89228=CARTESIAN_POINT('Ctrl Pts',(-188.599761728483,54.850018770448,142.681961197956));
#89229=CARTESIAN_POINT('Ctrl Pts',(-188.622338005758,54.8500180722034,142.48486992876));
#89230=CARTESIAN_POINT('Ctrl Pts',(-188.644527321077,54.8500171468879,142.287765317132));
#89231=CARTESIAN_POINT('Ctrl Pts',(-188.666339692097,54.8500159540699,142.090649333442));
#89232=CARTESIAN_POINT('Ctrl Pts',(-188.793874655865,54.850008979771,140.938129975725));
#89233=CARTESIAN_POINT('Ctrl Pts',(-188.90862770106,54.8500087186653,139.78461609317));
#89234=CARTESIAN_POINT('Ctrl Pts',(-189.012550625685,54.8500098332402,138.63033201508));
#89235=CARTESIAN_POINT('Ctrl Pts',(-189.132704196567,54.8500111218891,137.295772250766));
#89236=CARTESIAN_POINT('Ctrl Pts',(-189.238379958311,54.8500142498538,135.960182025919));
#89237=CARTESIAN_POINT('Ctrl Pts',(-189.332524646315,54.8500109691833,134.623907387355));
#89238=CARTESIAN_POINT('Ctrl Pts',(-189.343237480957,54.850010595872,134.471851126477));
#89239=CARTESIAN_POINT('Ctrl Pts',(-189.353801068778,54.8500101395807,134.319776825197));
#89240=CARTESIAN_POINT('Ctrl Pts',(-189.364218337543,54.8500095881607,134.167683191866));
#89241=CARTESIAN_POINT('Ctrl Pts',(-189.493454219205,54.8500027472846,132.280820594396));
#89242=CARTESIAN_POINT('Ctrl Pts',(-189.600125024046,54.8500055486022,130.392311238613));
#89243=CARTESIAN_POINT('Ctrl Pts',(-189.689765383739,54.850006017259,128.50255729975));
#89244=CARTESIAN_POINT('Ctrl Pts',(-189.720518645157,54.8500061780429,127.854232180394));
#89245=CARTESIAN_POINT('Ctrl Pts',(-189.749267897846,54.8500060642914,127.205760606272));
#89246=CARTESIAN_POINT('Ctrl Pts',(-189.776237985562,54.8500051925039,126.557158904599));
#89247=CARTESIAN_POINT('Ctrl Pts',(-189.780843967841,54.850005043619,126.446389967722));
#89248=CARTESIAN_POINT('Ctrl Pts',(-189.785397775027,54.8500048726252,126.335617228642));
#89249=CARTESIAN_POINT('Ctrl Pts',(-189.789900160442,54.8500046771144,126.224840759492));
#89250=CARTESIAN_POINT('Ctrl Pts',(-189.883899653494,54.8500005952975,123.912081858822));
#89251=CARTESIAN_POINT('Ctrl Pts',(-189.955534459011,54.8500116062881,121.597690348618));
#89252=CARTESIAN_POINT('Ctrl Pts',(-190.011686299581,54.8500111214795,119.282167861307));
#89253=CARTESIAN_POINT('Ctrl Pts',(-190.01812560416,54.8500110658833,119.016631515502));
#89254=CARTESIAN_POINT('Ctrl Pts',(-190.0243613518,54.8500108591021,118.751080301671));
#89255=CARTESIAN_POINT('Ctrl Pts',(-190.030403961542,54.8500104610399,118.485514979907));
#89256=CARTESIAN_POINT('Ctrl Pts',(-190.032047390757,54.8500103527776,118.413288272079));
#89257=CARTESIAN_POINT('Ctrl Pts',(-190.033676869816,54.8500102303663,118.341060525259));
#89258=CARTESIAN_POINT('Ctrl Pts',(-190.035292521922,54.8500100929995,118.268831752682));
#89259=CARTESIAN_POINT('Ctrl Pts',(-190.104937525408,54.8500041716088,115.155306818301));
#89260=CARTESIAN_POINT('Ctrl Pts',(-190.148948120071,54.8500017243381,112.039912168456));
#89261=CARTESIAN_POINT('Ctrl Pts',(-190.177365979128,54.850000712722,108.923379427127));
#89262=CARTESIAN_POINT('Ctrl Pts',(-190.197388942463,54.8499999999465,106.727498988393));
#89263=CARTESIAN_POINT('Ctrl Pts',(-190.209672545854,54.8499999999605,104.531053605748));
#89264=CARTESIAN_POINT('Ctrl Pts',(-190.217744333281,54.85,102.334299700914));
#89265=CARTESIAN_POINT('Origin',(-189.999800857363,55.3,102.333498885934));
#89266=CARTESIAN_POINT('Origin',(160.5,55.3,102.225104347672));
#89267=CARTESIAN_POINT('',(190.217944947177,54.85,102.225104347672));
#89268=CARTESIAN_POINT('Origin',(160.5,54.85,102.225104347672));
#89269=CARTESIAN_POINT('Origin',(190.,55.3,102.225104347672));
#89270=CARTESIAN_POINT('Origin',(-160.5,55.3,102.225104347671));
#89271=CARTESIAN_POINT('',(-190.217944947177,54.85,102.225104347671));
#89272=CARTESIAN_POINT('Origin',(-160.5,54.85,102.225104347671));
#89273=CARTESIAN_POINT('Origin',(-190.,55.3,102.225104347671));
#89274=CARTESIAN_POINT('Origin',(190.,55.3,211.4));
#89275=CARTESIAN_POINT('',(190.104681191176,54.811080938995,40.5));
#89276=CARTESIAN_POINT('',(190.217944947177,54.85,41.));
#89277=CARTESIAN_POINT('Ctrl Pts',(190.104681191175,54.8110809389947,40.5000000000008));
#89278=CARTESIAN_POINT('Ctrl Pts',(190.12358091403,54.8151275096016,40.5320279313255));
#89279=CARTESIAN_POINT('Ctrl Pts',(190.140604162343,54.8199259241617,40.5679467634758));
#89280=CARTESIAN_POINT('Ctrl Pts',(190.199161359621,54.8390668735187,40.725766780693));
#89281=CARTESIAN_POINT('Ctrl Pts',(190.217944947177,54.85,40.8634110132489));
#89282=CARTESIAN_POINT('Ctrl Pts',(190.217944947177,54.85,41.));
#89283=CARTESIAN_POINT('Origin',(190.,55.3,40.5));
#89284=CARTESIAN_POINT('',(190.217944947177,54.85,71.6125521738359));
#89285=CARTESIAN_POINT('Origin',(-190.,55.3,211.4));
#89286=CARTESIAN_POINT('',(-190.217944947177,54.85,41.));
#89287=CARTESIAN_POINT('',(-190.217944947177,54.85,71.6125521738355));
#89288=CARTESIAN_POINT('',(-190.104681191184,54.8110809389967,40.5));
#89289=CARTESIAN_POINT('Origin',(-190.,55.3,40.5));
#89290=CARTESIAN_POINT('Ctrl Pts',(-190.217944947177,54.85,41.));
#89291=CARTESIAN_POINT('Ctrl Pts',(-190.217944947177,54.85,40.9938389177394));
#89292=CARTESIAN_POINT('Ctrl Pts',(-190.217905298598,54.8499807908613,40.9876799790596));
#89293=CARTESIAN_POINT('Ctrl Pts',(-190.216401080532,54.849252755359,40.8708492263633));
#89294=CARTESIAN_POINT('Ctrl Pts',(-190.202442092343,54.8416051156352,40.7575089701039));
#89295=CARTESIAN_POINT('Ctrl Pts',(-190.15302607478,54.8236016547333,40.595037086274));
#89296=CARTESIAN_POINT('Ctrl Pts',(-190.130450467364,54.8165983318361,40.5436692439569));
#89297=CARTESIAN_POINT('Ctrl Pts',(-190.104681191177,54.8110809389952,40.5000000000045));
#89298=CARTESIAN_POINT('Origin',(-205.7,55.3,40.5));
#89299=CARTESIAN_POINT('',(-189.999999999997,54.811080938995,40.3953188088242));
#89300=CARTESIAN_POINT('',(-189.5,54.85,40.282055052823));
#89301=CARTESIAN_POINT('Ctrl Pts',(-189.999999999997,54.811080938995,40.3953188088242));
#89302=CARTESIAN_POINT('Ctrl Pts',(-189.967972070583,54.8151275093604,40.3764190870962));
#89303=CARTESIAN_POINT('Ctrl Pts',(-189.932053240841,54.8199259235839,40.3593958397075));
#89304=CARTESIAN_POINT('Ctrl Pts',(-189.774233224941,54.8390668729966,40.3008386411371));
#89305=CARTESIAN_POINT('Ctrl Pts',(-189.636588989633,54.85,40.282055052823));
#89306=CARTESIAN_POINT('Ctrl Pts',(-189.5,54.85,40.282055052823));
#89307=CARTESIAN_POINT('Origin',(-190.,55.3,40.5));
#89308=CARTESIAN_POINT('',(190.,54.8110809389967,40.3953188088159));
#89309=CARTESIAN_POINT('Origin',(190.,55.3,40.5));
#89310=CARTESIAN_POINT('',(189.5,54.85,40.282055052823));
#89311=CARTESIAN_POINT('Ctrl Pts',(189.5,54.85,40.282055052823));
#89312=CARTESIAN_POINT('Ctrl Pts',(189.506161082261,54.85,40.282055052823));
#89313=CARTESIAN_POINT('Ctrl Pts',(189.51232002094,54.8499807908613,40.2820947014021));
#89314=CARTESIAN_POINT('Ctrl Pts',(189.629150773595,54.8492527553593,40.283598919467));
#89315=CARTESIAN_POINT('Ctrl Pts',(189.742491029857,54.8416051156395,40.2975579076449));
#89316=CARTESIAN_POINT('Ctrl Pts',(189.904962913708,54.8236016547353,40.3469739252141));
#89317=CARTESIAN_POINT('Ctrl Pts',(189.95633075603,54.8165983318378,40.3695495326286));
#89318=CARTESIAN_POINT('Ctrl Pts',(189.999999999996,54.8110809389952,40.3953188088232));
#89319=CARTESIAN_POINT('',(-2.77555756156289E-14,54.85,40.282055052823));
#89320=CARTESIAN_POINT('Origin',(190.,55.3,40.5));
#89321=CARTESIAN_POINT('Ctrl Pts',(189.999999999995,54.8110809389952,40.3953188088232));
#89322=CARTESIAN_POINT('Ctrl Pts',(190.02146654402,54.8083687474021,40.4079862436505));
#89323=CARTESIAN_POINT('Ctrl Pts',(190.042396677867,54.8069935753319,40.4245436742059));
#89324=CARTESIAN_POINT('Ctrl Pts',(190.075456325793,54.8069935753319,40.457603322132));
#89325=CARTESIAN_POINT('Ctrl Pts',(190.092013756348,54.8083687474019,40.4785334559779));
#89326=CARTESIAN_POINT('Ctrl Pts',(190.104681191175,54.8110809389947,40.5000000000008));
#89327=CARTESIAN_POINT('Origin',(190.,55.3,40.5));
#89328=CARTESIAN_POINT('Origin',(-190.,55.3,40.5));
#89329=CARTESIAN_POINT('Ctrl Pts',(-190.104681191177,54.8110809389952,40.5000000000045));
#89330=CARTESIAN_POINT('Ctrl Pts',(-190.09201375635,54.8083687474021,40.4785334559804));
#89331=CARTESIAN_POINT('Ctrl Pts',(-190.075456325794,54.8069935753319,40.457603322133));
#89332=CARTESIAN_POINT('Ctrl Pts',(-190.042396677867,54.8069935753319,40.4245436742064));
#89333=CARTESIAN_POINT('Ctrl Pts',(-190.021466544021,54.808368747402,40.4079862436513));
#89334=CARTESIAN_POINT('Ctrl Pts',(-189.999999999997,54.811080938995,40.3953188088242));
#89335=CARTESIAN_POINT('Origin',(-190.,55.3,40.5));
#89336=CARTESIAN_POINT('Origin',(190.,58.8,40.5));
#89337=CARTESIAN_POINT('Origin',(190.,58.3,40.5));
#89338=CARTESIAN_POINT('Origin',(-190.,58.8,40.5));
#89339=CARTESIAN_POINT('Origin',(-190.,58.2999999999999,40.5));
#89340=CARTESIAN_POINT('Origin',(-190.5,58.2999999999999,40.5));
#89341=CARTESIAN_POINT('Origin',(190.,58.3,40.5));
#89342=CARTESIAN_POINT('Origin',(-190.,58.2999999999999,40.5));
#89343=CARTESIAN_POINT('Origin',(190.,58.3,40.5));
#89344=CARTESIAN_POINT('Origin',(190.,58.3,40.5));
#89345=CARTESIAN_POINT('Origin',(-190.,58.2999999999999,40.5));
#89346=CARTESIAN_POINT('Origin',(-190.,58.2999999999999,40.5));
#89347=CARTESIAN_POINT('Origin',(190.,58.3,211.4));
#89348=CARTESIAN_POINT('Origin',(190.,58.3,102.225104347672));
#89349=CARTESIAN_POINT('Origin',(-190.,58.2999999999999,211.4));
#89350=CARTESIAN_POINT('Origin',(-190.,58.2999999999999,102.225104347671));
#89351=CARTESIAN_POINT('Origin',(160.5,58.3,102.225104347672));
#89352=CARTESIAN_POINT('Origin',(189.999800857363,58.3,102.333498885935));
#89353=CARTESIAN_POINT('Origin',(-160.5,58.3,102.225104347671));
#89354=CARTESIAN_POINT('Origin',(-189.999800857363,58.2999999999999,102.333498885934));
#89355=CARTESIAN_POINT('Ctrl Pts',(189.999800857363,58.8,102.333498885935));
#89356=CARTESIAN_POINT('Ctrl Pts',(190.499797482064,58.8,102.335336081499));
#89357=CARTESIAN_POINT('Ctrl Pts',(190.499797482064,58.3,102.335336081499));
#89358=CARTESIAN_POINT('Ctrl Pts',(189.98001814498,58.8,107.717405584026));
#89359=CARTESIAN_POINT('Ctrl Pts',(190.48000829834,58.8000000000187,107.721003970607));
#89360=CARTESIAN_POINT('Ctrl Pts',(190.480008298168,58.3,107.721003970608));
#89361=CARTESIAN_POINT('Ctrl Pts',(189.934928325224,58.8,113.100441490038));
#89362=CARTESIAN_POINT('Ctrl Pts',(190.434912437463,58.8,113.106828120133));
#89363=CARTESIAN_POINT('Ctrl Pts',(190.434912437371,58.3,113.106828120131));
#89364=CARTESIAN_POINT('Ctrl Pts',(189.751276588517,58.8,121.170613300806));
#89365=CARTESIAN_POINT('Ctrl Pts',(190.251090404861,58.8,121.184483209912));
#89366=CARTESIAN_POINT('Ctrl Pts',(190.251090404907,58.3,121.184483209913));
#89367=CARTESIAN_POINT('Ctrl Pts',(189.670257242378,58.8,123.859931990418));
#89368=CARTESIAN_POINT('Ctrl Pts',(190.16998581163,58.7999999999253,123.876850850614));
#89369=CARTESIAN_POINT('Ctrl Pts',(190.169985811573,58.3,123.876850850612));
#89370=CARTESIAN_POINT('Ctrl Pts',(189.446683812013,58.8,129.236274242029));
#89371=CARTESIAN_POINT('Ctrl Pts',(189.946091720075,58.8000000000747,129.260904144743));
#89372=CARTESIAN_POINT('Ctrl Pts',(189.946091720133,58.3,129.260904144745));
#89373=CARTESIAN_POINT('Ctrl Pts',(189.304296283357,58.8,131.923304015849));
#89374=CARTESIAN_POINT('Ctrl Pts',(189.803472315597,58.8000000000374,131.952591176853));
#89375=CARTESIAN_POINT('Ctrl Pts',(189.803472315518,58.3,131.952591176848));
#89376=CARTESIAN_POINT('Ctrl Pts',(188.925895877044,58.8,137.293871517213));
#89377=CARTESIAN_POINT('Ctrl Pts',(189.424246871052,58.7999999999626,137.334868293952));
#89378=CARTESIAN_POINT('Ctrl Pts',(189.424246871131,58.3,137.334868293958));
#89379=CARTESIAN_POINT('Ctrl Pts',(188.689842755583,58.8,139.98027909287));
#89380=CARTESIAN_POINT('Ctrl Pts',(189.187608240863,58.8000000000561,140.028330517364));
#89381=CARTESIAN_POINT('Ctrl Pts',(189.187608240723,58.3000000000561,140.028330517352));
#89382=CARTESIAN_POINT('Ctrl Pts',(188.076546005068,58.8,145.334025694771));
#89383=CARTESIAN_POINT('Ctrl Pts',(188.572283011502,58.799999999944,145.399784634286));
#89384=CARTESIAN_POINT('Ctrl Pts',(188.572283011643,58.2999999999439,145.399784634298));
#89385=CARTESIAN_POINT('Ctrl Pts',(187.700189235296,58.8,147.997700373917));
#89386=CARTESIAN_POINT('Ctrl Pts',(188.194503693773,58.8,148.07409498293));
#89387=CARTESIAN_POINT('Ctrl Pts',(188.194503693509,58.3,148.074094982882));
#89388=CARTESIAN_POINT('Ctrl Pts',(186.736003435206,58.8,153.285009470243));
#89389=CARTESIAN_POINT('Ctrl Pts',(187.225465197661,58.8,153.388014825357));
#89390=CARTESIAN_POINT('Ctrl Pts',(187.225465197925,58.3,153.388014825405));
#89391=CARTESIAN_POINT('Ctrl Pts',(186.148938776817,58.8,155.908788613842));
#89392=CARTESIAN_POINT('Ctrl Pts',(186.635007347117,58.8000000000187,156.027789475654));
#89393=CARTESIAN_POINT('Ctrl Pts',(186.635007346696,58.3000000000375,156.027789475543));
#89394=CARTESIAN_POINT('Ctrl Pts',(185.02518086126,58.8,159.798417119283));
#89395=CARTESIAN_POINT('Ctrl Pts',(185.502677893295,58.7999999999906,159.947086381067));
#89396=CARTESIAN_POINT('Ctrl Pts',(185.502677893506,58.2999999999813,159.947086381122));
#89397=CARTESIAN_POINT('Ctrl Pts',(184.609198475717,58.8,161.087318261543));
#89398=CARTESIAN_POINT('Ctrl Pts',(185.083234340728,58.8000000000093,161.246835918548));
#89399=CARTESIAN_POINT('Ctrl Pts',(185.083234340555,58.3000000000187,161.246835918492));
#89400=CARTESIAN_POINT('Ctrl Pts',(183.687943117541,58.8,163.61446540035));
#89401=CARTESIAN_POINT('Ctrl Pts',(184.153426616828,58.7999999999907,163.797443530339));
#89402=CARTESIAN_POINT('Ctrl Pts',(184.153426617001,58.2999999999813,163.797443530395));
#89403=CARTESIAN_POINT('Ctrl Pts',(183.181708976339,58.8,164.856292405152));
#89404=CARTESIAN_POINT('Ctrl Pts',(183.64209143492,58.8,165.051912885673));
#89405=CARTESIAN_POINT('Ctrl Pts',(183.642091434722,58.3,165.051912885582));
#89406=CARTESIAN_POINT('Ctrl Pts',(182.06196560612,58.8,167.28879435183));
#89407=CARTESIAN_POINT('Ctrl Pts',(182.509961211144,58.8,167.51132371713));
#89408=CARTESIAN_POINT('Ctrl Pts',(182.509961211343,58.3,167.511323717222));
#89409=CARTESIAN_POINT('Ctrl Pts',(181.448441342018,58.8,168.479462124495));
#89410=CARTESIAN_POINT('Ctrl Pts',(181.889144137848,58.7999999999627,168.716261729601));
#89411=CARTESIAN_POINT('Ctrl Pts',(181.889144137668,58.299999999972,168.716261729504));
#89412=CARTESIAN_POINT('Ctrl Pts',(180.434508985192,58.8,170.220810507743));
#89413=CARTESIAN_POINT('Ctrl Pts',(180.862291929331,58.8000000000186,170.479798933213));
#89414=CARTESIAN_POINT('Ctrl Pts',(180.862291929421,58.300000000014,170.479798933262));
#89415=CARTESIAN_POINT('Ctrl Pts',(180.080913450215,58.8,170.793812786376));
#89416=CARTESIAN_POINT('Ctrl Pts',(180.504061049942,58.800000000007,171.060324592655));
#89417=CARTESIAN_POINT('Ctrl Pts',(180.50406104985,58.3,171.060324592596));
#89418=CARTESIAN_POINT('Ctrl Pts',(179.340199864572,58.8,171.923832776648));
#89419=CARTESIAN_POINT('Ctrl Pts',(179.753392709512,58.7999999999929,172.205531386738));
#89420=CARTESIAN_POINT('Ctrl Pts',(179.753392709603,58.3,172.205531386798));
#89421=CARTESIAN_POINT('Ctrl Pts',(178.951622144051,58.8,172.482731520272));
#89422=CARTESIAN_POINT('Ctrl Pts',(179.359474666006,58.7999999999953,172.772119981183));
#89423=CARTESIAN_POINT('Ctrl Pts',(179.359474666015,58.3,172.772119981182));
#89424=CARTESIAN_POINT('Ctrl Pts',(176.94243620339,58.8,175.203904423759));
#89425=CARTESIAN_POINT('Ctrl Pts',(177.322213675789,58.8000000000187,175.531316774216));
#89426=CARTESIAN_POINT('Ctrl Pts',(177.322213675755,58.3,175.531316774218));
#89427=CARTESIAN_POINT('Ctrl Pts',(175.119316602416,58.8,177.151741641064));
#89428=CARTESIAN_POINT('Ctrl Pts',(175.472027446722,58.8,177.508051660755));
#89429=CARTESIAN_POINT('Ctrl Pts',(175.472027446818,58.3,177.508051660867));
#89430=CARTESIAN_POINT('Ctrl Pts',(172.078138682654,58.8,179.748063563884));
#89431=CARTESIAN_POINT('Ctrl Pts',(172.388751140008,58.8,180.140313922463));
#89432=CARTESIAN_POINT('Ctrl Pts',(172.38875113996,58.3,180.140313922407));
#89433=CARTESIAN_POINT('Ctrl Pts',(171.013690961684,58.8,180.55964888304));
#89434=CARTESIAN_POINT('Ctrl Pts',(171.310063503812,58.8,180.962699537774));
#89435=CARTESIAN_POINT('Ctrl Pts',(171.310063503882,58.3,180.962699537876));
#89436=CARTESIAN_POINT('Ctrl Pts',(169.345685170052,58.8,181.701285645969));
#89437=CARTESIAN_POINT('Ctrl Pts',(169.621105252467,58.8,182.118676837442));
#89438=CARTESIAN_POINT('Ctrl Pts',(169.621105252432,58.3,182.118676837391));
#89439=CARTESIAN_POINT('Ctrl Pts',(168.776138991726,58.8,182.070221274742));
#89440=CARTESIAN_POINT('Ctrl Pts',(169.044621938208,58.8000000000094,182.492098102594));
#89441=CARTESIAN_POINT('Ctrl Pts',(169.044621938292,58.3,182.4920981027));
#89442=CARTESIAN_POINT('Ctrl Pts',(167.623396019067,58.8,182.778344901968));
#89443=CARTESIAN_POINT('Ctrl Pts',(167.878336591531,58.7999999999906,183.208540735228));
#89444=CARTESIAN_POINT('Ctrl Pts',(167.878336591447,58.3,183.208540735122));
#89445=CARTESIAN_POINT('Ctrl Pts',(167.040752911306,58.8,183.117347354141));
#89446=CARTESIAN_POINT('Ctrl Pts',(167.289093057169,58.7999999999999,183.551375891322));
#89447=CARTESIAN_POINT('Ctrl Pts',(167.289093057208,58.3,183.551375891393));
#89448=CARTESIAN_POINT('Ctrl Pts',(164.099002476116,58.8,184.743841876051));
#89449=CARTESIAN_POINT('Ctrl Pts',(164.315307422483,58.7999999999999,185.19558268275));
#89450=CARTESIAN_POINT('Ctrl Pts',(164.315307422327,58.3,185.195582682467));
#89451=CARTESIAN_POINT('Ctrl Pts',(161.655214786853,58.8,185.828000216715));
#89452=CARTESIAN_POINT('Ctrl Pts',(161.849125213937,58.8000000000928,186.289321051912));
#89453=CARTESIAN_POINT('Ctrl Pts',(161.849125214018,58.3000000000371,186.28932105219));
#89454=CARTESIAN_POINT('Ctrl Pts',(157.896230834854,58.8,187.230200792056));
#89455=CARTESIAN_POINT('Ctrl Pts',(158.061401990429,58.7999999999536,187.702242136669));
#89456=CARTESIAN_POINT('Ctrl Pts',(158.061401990388,58.2999999999814,187.702242136529));
#89457=CARTESIAN_POINT('Ctrl Pts',(156.627499515221,58.8,187.65981423508));
#89458=CARTESIAN_POINT('Ctrl Pts',(156.783872375754,58.8,188.134808550835));
#89459=CARTESIAN_POINT('Ctrl Pts',(156.783872375793,58.3,188.13480855096));
#89460=CARTESIAN_POINT('Ctrl Pts',(154.063722484356,58.8,188.45585523812));
#89461=CARTESIAN_POINT('Ctrl Pts',(154.203880012417,58.8,188.935884340214));
#89462=CARTESIAN_POINT('Ctrl Pts',(154.203880012378,58.3,188.93588434009));
#89463=CARTESIAN_POINT('Ctrl Pts',(152.766177004478,58.8,188.822895905688));
#89464=CARTESIAN_POINT('Ctrl Pts',(152.898903325027,58.800000000014,189.305009231201));
#89465=CARTESIAN_POINT('Ctrl Pts',(152.898903325061,58.3000000000094,189.305009231311));
#89466=CARTESIAN_POINT('Ctrl Pts',(148.859060109736,58.8,189.839592196685));
#89467=CARTESIAN_POINT('Ctrl Pts',(148.971352624484,58.799999999972,190.327022735643));
#89468=CARTESIAN_POINT('Ctrl Pts',(148.971352624418,58.2999999999813,190.327022735424));
#89469=CARTESIAN_POINT('Ctrl Pts',(146.243348297063,58.8000000000001,190.40454102088));
#89470=CARTESIAN_POINT('Ctrl Pts',(146.344500438298,58.7999999999816,190.894297995552));
#89471=CARTESIAN_POINT('Ctrl Pts',(146.344500438332,58.299999999963,190.894297995767));
#89472=CARTESIAN_POINT('Ctrl Pts',(140.997169684061,58.8000000000001,191.382615165563));
#89473=CARTESIAN_POINT('Ctrl Pts',(141.079295090469,58.8000000000186,191.875919399834));
#89474=CARTESIAN_POINT('Ctrl Pts',(141.079295090435,58.3000000000371,191.87591939962));
#89475=CARTESIAN_POINT('Ctrl Pts',(138.366646422257,58.8,191.79515951725));
#89476=CARTESIAN_POINT('Ctrl Pts',(138.44089270479,58.7999999998615,192.28966379588));
#89477=CARTESIAN_POINT('Ctrl Pts',(138.440892704796,58.2999999999077,192.289663795997));
#89478=CARTESIAN_POINT('Ctrl Pts',(133.095165732956,58.8,192.512884413628));
#89479=CARTESIAN_POINT('Ctrl Pts',(133.155827195428,58.8000000001384,193.009238298581));
#89480=CARTESIAN_POINT('Ctrl Pts',(133.155827195422,58.3000000000922,193.009238298464));
#89481=CARTESIAN_POINT('Ctrl Pts',(130.454180717654,58.8,192.817781092679));
#89482=CARTESIAN_POINT('Ctrl Pts',(130.509142871665,58.7999999999723,193.314776001534));
#89483=CARTESIAN_POINT('Ctrl Pts',(130.50914287167,58.2999999999815,193.31477600159));
#89484=CARTESIAN_POINT('Ctrl Pts',(122.519844509471,58.8,193.615363067465));
#89485=CARTESIAN_POINT('Ctrl Pts',(122.559948354903,58.8000000000553,194.113851575618));
#89486=CARTESIAN_POINT('Ctrl Pts',(122.559948354892,58.3000000000369,194.113851575507));
#89487=CARTESIAN_POINT('Ctrl Pts',(117.215350992657,58.8,193.993397868622));
#89488=CARTESIAN_POINT('Ctrl Pts',(117.248473697783,58.8000000000554,194.492330262396));
#89489=CARTESIAN_POINT('Ctrl Pts',(117.248473697793,58.3000000000369,194.492330262573));
#89490=CARTESIAN_POINT('Ctrl Pts',(106.589963387299,58.8,194.580711495763));
#89491=CARTESIAN_POINT('Ctrl Pts',(106.612030995818,58.7999999999446,195.080254955117));
#89492=CARTESIAN_POINT('Ctrl Pts',(106.612030995808,58.2999999999631,195.08025495494));
#89493=CARTESIAN_POINT('Ctrl Pts',(101.268901729087,58.8,194.788266093034));
#89494=CARTESIAN_POINT('Ctrl Pts',(101.28694296775,58.8000000002218,195.28795077722));
#89495=CARTESIAN_POINT('Ctrl Pts',(101.286942967794,58.3000000001479,195.287950777393));
#89496=CARTESIAN_POINT('Ctrl Pts',(90.6171697705162,58.8,195.104505818827));
#89497=CARTESIAN_POINT('Ctrl Pts',(90.6288044986965,58.7999999997782,195.604380706148));
#89498=CARTESIAN_POINT('Ctrl Pts',(90.6288044986522,58.2999999998521,195.604380705975));
#89499=CARTESIAN_POINT('Ctrl Pts',(85.285877912414,58.8,195.212489935321));
#89500=CARTESIAN_POINT('Ctrl Pts',(85.2951502476821,58.800000000074,195.712407432941));
#89501=CARTESIAN_POINT('Ctrl Pts',(85.2951502476829,58.3,195.712407432999));
#89502=CARTESIAN_POINT('Ctrl Pts',(74.6256438147839,58.8,195.370425946995));
#89503=CARTESIAN_POINT('Ctrl Pts',(74.6311852893859,58.799999999926,195.870398718872));
#89504=CARTESIAN_POINT('Ctrl Pts',(74.6311852893851,58.3,195.870398718815));
#89505=CARTESIAN_POINT('Ctrl Pts',(69.2954065338737,58.8,195.420095627817));
#89506=CARTESIAN_POINT('Ctrl Pts',(69.2995860601197,58.800000000037,195.920079260185));
#89507=CARTESIAN_POINT('Ctrl Pts',(69.2995860601212,58.300000000111,195.920079260346));
#89508=CARTESIAN_POINT('Ctrl Pts',(53.3044940404725,58.8,195.520209490268));
#89509=CARTESIAN_POINT('Ctrl Pts',(53.3055258122745,58.799999999926,196.020212829384));
#89510=CARTESIAN_POINT('Ctrl Pts',(53.3055258122716,58.2999999997781,196.020212829063));
#89511=CARTESIAN_POINT('Ctrl Pts',(42.6436273390892,58.8,195.523991419473));
#89512=CARTESIAN_POINT('Ctrl Pts',(42.6437804406409,58.8000000004438,196.0239915327));
#89513=CARTESIAN_POINT('Ctrl Pts',(42.6437804406409,58.3000000002959,196.023991532478));
#89514=CARTESIAN_POINT('Ctrl Pts',(21.3218250167947,58.8,195.514760894498));
#89515=CARTESIAN_POINT('Ctrl Pts',(21.32123900044,58.7999999995561,196.014760687562));
#89516=CARTESIAN_POINT('Ctrl Pts',(21.32123900044,58.2999999997041,196.014760687785));
#89517=CARTESIAN_POINT('Ctrl Pts',(10.6608798724039,58.8,195.500000000296));
#89518=CARTESIAN_POINT('Ctrl Pts',(10.6604701167662,58.799999999778,196.000000000296));
#89519=CARTESIAN_POINT('Ctrl Pts',(10.6604701167663,58.3,196.));
#89520=CARTESIAN_POINT('Ctrl Pts',(1.14409252987596E-14,58.8,195.5));
#89521=CARTESIAN_POINT('Ctrl Pts',(1.15828019241431E-14,58.8,196.));
#89522=CARTESIAN_POINT('Ctrl Pts',(1.16465450439953E-14,58.3,196.));
#89523=CARTESIAN_POINT('Origin',(1.15046684186118E-14,58.3,195.5));
#89524=CARTESIAN_POINT('Ctrl Pts',(1.15828019241431E-14,58.8,195.5));
#89525=CARTESIAN_POINT('Ctrl Pts',(1.15828019241431E-14,58.8,196.));
#89526=CARTESIAN_POINT('Ctrl Pts',(1.16465450439953E-14,58.3,196.));
#89527=CARTESIAN_POINT('Ctrl Pts',(-10.7118202846616,58.8,195.500000000149));
#89528=CARTESIAN_POINT('Ctrl Pts',(-10.7114086955145,58.7999999998885,196.000000000149));
#89529=CARTESIAN_POINT('Ctrl Pts',(-10.7114086955145,58.3,196.));
#89530=CARTESIAN_POINT('Ctrl Pts',(-21.4237296695725,58.8,195.514918536095));
#89531=CARTESIAN_POINT('Ctrl Pts',(-21.4231418326548,58.8000000001487,196.01491833246));
#89532=CARTESIAN_POINT('Ctrl Pts',(-21.4231418326549,58.3,196.014918332428));
#89533=CARTESIAN_POINT('Ctrl Pts',(-42.8474268144279,58.8,195.523964494094));
#89534=CARTESIAN_POINT('Ctrl Pts',(-42.8475924106281,58.7999999998513,196.023964608585));
#89535=CARTESIAN_POINT('Ctrl Pts',(-42.8475924106281,58.3,196.023964608617));
#89536=CARTESIAN_POINT('Ctrl Pts',(-53.5592277847632,58.8,195.519892463612));
#89537=CARTESIAN_POINT('Ctrl Pts',(-53.5602852850042,58.8000000001115,196.019895896343));
#89538=CARTESIAN_POINT('Ctrl Pts',(-53.5602852850042,58.3000000000743,196.019895896345));
#89539=CARTESIAN_POINT('Ctrl Pts',(-69.6263951900445,58.8,195.417356847765));
#89540=CARTESIAN_POINT('Ctrl Pts',(-69.6306526068966,58.7999999999442,195.917339859648));
#89541=CARTESIAN_POINT('Ctrl Pts',(-69.6306526068966,58.2999999999628,195.917339859647));
#89542=CARTESIAN_POINT('Ctrl Pts',(-74.982025485357,58.8,195.36653562557));
#89543=CARTESIAN_POINT('Ctrl Pts',(-74.9876678043093,58.7999999999256,195.86650739624));
#89544=CARTESIAN_POINT('Ctrl Pts',(-74.9876678043095,58.3,195.866507396251));
#89545=CARTESIAN_POINT('Ctrl Pts',(-85.6929541822509,58.8,195.204966816963));
#89546=CARTESIAN_POINT('Ctrl Pts',(-85.7023946291779,58.8000000000743,195.704881294909));
#89547=CARTESIAN_POINT('Ctrl Pts',(-85.7023946291777,58.3,195.704881294898));
#89548=CARTESIAN_POINT('Ctrl Pts',(-91.0488456914488,58.8,195.094552429692));
#89549=CARTESIAN_POINT('Ctrl Pts',(-91.0606918125482,58.7999999998699,195.594422790096));
#89550=CARTESIAN_POINT('Ctrl Pts',(-91.0606918125442,58.2999999999628,195.594422789964));
#89551=CARTESIAN_POINT('Ctrl Pts',(-101.757516044794,58.8,194.770640584481));
#89552=CARTESIAN_POINT('Ctrl Pts',(-101.775903721111,58.8000000001301,195.270313078333));
#89553=CARTESIAN_POINT('Ctrl Pts',(-101.775903721115,58.3000000000371,195.270313078465));
#89554=CARTESIAN_POINT('Ctrl Pts',(-107.107721166644,58.8,194.557957974675));
#89555=CARTESIAN_POINT('Ctrl Pts',(-107.130224336241,58.7999999999257,195.057483582615));
#89556=CARTESIAN_POINT('Ctrl Pts',(-107.130224336237,58.2999999999999,195.057483582537));
#89557=CARTESIAN_POINT('Ctrl Pts',(-117.793666862769,58.8,193.954934442877));
#89558=CARTESIAN_POINT('Ctrl Pts',(-117.827505515304,58.8000000000742,194.453820372871));
#89559=CARTESIAN_POINT('Ctrl Pts',(-117.827505515308,58.2999999999999,194.453820372949));
#89560=CARTESIAN_POINT('Ctrl Pts',(-123.129559723837,58.8,193.566463954364));
#89561=CARTESIAN_POINT('Ctrl Pts',(-123.170566875692,58.7999999999999,194.064885467423));
#89562=CARTESIAN_POINT('Ctrl Pts',(-123.170566875683,58.3,194.06488546734));
#89563=CARTESIAN_POINT('Ctrl Pts',(-131.113885005264,58.8,192.74408075586));
#89564=CARTESIAN_POINT('Ctrl Pts',(-131.170224675438,58.7999999999999,193.240923023939));
#89565=CARTESIAN_POINT('Ctrl Pts',(-131.170224675442,58.3,193.240923023981));
#89566=CARTESIAN_POINT('Ctrl Pts',(-133.772021287641,58.8,192.429354057039));
#89567=CARTESIAN_POINT('Ctrl Pts',(-133.834251546661,58.8000000000557,192.925517262575));
#89568=CARTESIAN_POINT('Ctrl Pts',(-133.834251546645,58.3000000000185,192.925517262463));
#89569=CARTESIAN_POINT('Ctrl Pts',(-137.752328543611,58.8,191.872550736023));
#89570=CARTESIAN_POINT('Ctrl Pts',(-137.82511882244,58.7999999999721,192.367236705325));
#89571=CARTESIAN_POINT('Ctrl Pts',(-137.825118822448,58.2999999999907,192.36723670538));
#89572=CARTESIAN_POINT('Ctrl Pts',(-139.077940504066,58.8,191.672737442318));
#89573=CARTESIAN_POINT('Ctrl Pts',(-139.154540611854,58.7999999999906,192.166853050365));
#89574=CARTESIAN_POINT('Ctrl Pts',(-139.154540611843,58.2999999999906,192.166853050303));
#89575=CARTESIAN_POINT('Ctrl Pts',(-141.726406587006,58.8,191.239238184666));
#89576=CARTESIAN_POINT('Ctrl Pts',(-141.811336381096,58.8000000000093,191.73199039492));
#89577=CARTESIAN_POINT('Ctrl Pts',(-141.811336381106,58.3000000000093,191.731990394982));
#89578=CARTESIAN_POINT('Ctrl Pts',(-143.050153383207,58.7999999999999,191.005369438704));
#89579=CARTESIAN_POINT('Ctrl Pts',(-143.139606665615,58.7999999999999,191.497328231557));
#89580=CARTESIAN_POINT('Ctrl Pts',(-143.1396066656,58.2999999999999,191.497328231477));
#89581=CARTESIAN_POINT('Ctrl Pts',(-147.003773115755,58.7999999999999,190.245280923907));
#89582=CARTESIAN_POINT('Ctrl Pts',(-147.108057529436,58.7999999999999,190.734388412564));
#89583=CARTESIAN_POINT('Ctrl Pts',(-147.108057529467,58.2999999999999,190.734388412723));
#89584=CARTESIAN_POINT('Ctrl Pts',(-149.619187452484,58.7999999999999,189.661180882931));
#89585=CARTESIAN_POINT('Ctrl Pts',(-149.735031156308,58.7999999999442,190.147792646827));
#89586=CARTESIAN_POINT('Ctrl Pts',(-149.735031156257,58.2999999999628,190.147792646636));
#89587=CARTESIAN_POINT('Ctrl Pts',(-153.498376682197,58.7999999999999,188.617845764116));
#89588=CARTESIAN_POINT('Ctrl Pts',(-153.635250053141,58.8000000000278,189.098801451736));
#89589=CARTESIAN_POINT('Ctrl Pts',(-153.635250053166,58.3000000000185,189.098801451831));
#89590=CARTESIAN_POINT('Ctrl Pts',(-154.784060017518,58.7999999999999,188.241983654962));
#89591=CARTESIAN_POINT('Ctrl Pts',(-154.928562946898,58.8000000000278,188.720727975089));
#89592=CARTESIAN_POINT('Ctrl Pts',(-154.928562946852,58.3000000000185,188.720727974947));
#89593=CARTESIAN_POINT('Ctrl Pts',(-157.337498640619,58.7999999999999,187.422033931746));
#89594=CARTESIAN_POINT('Ctrl Pts',(-157.498735050851,58.799999999972,187.895404865258));
#89595=CARTESIAN_POINT('Ctrl Pts',(-157.498735050897,58.2999999999813,187.8954048654));
#89596=CARTESIAN_POINT('Ctrl Pts',(-158.606653739105,58.8,186.977439099048));
#89597=CARTESIAN_POINT('Ctrl Pts',(-158.777006808703,58.800000000028,187.447644908311));
#89598=CARTESIAN_POINT('Ctrl Pts',(-158.777006808644,58.3000000000187,187.447644908159));
#89599=CARTESIAN_POINT('Ctrl Pts',(-162.372251203529,58.8,185.52164141396));
#89600=CARTESIAN_POINT('Ctrl Pts',(-162.572437434611,58.799999999944,185.980313582696));
#89601=CARTESIAN_POINT('Ctrl Pts',(-162.572437434729,58.2999999999626,185.980313583));
#89602=CARTESIAN_POINT('Ctrl Pts',(-164.798663242189,58.8,184.400617898551));
#89603=CARTESIAN_POINT('Ctrl Pts',(-165.02194750263,58.8000000000555,184.848989685973));
#89604=CARTESIAN_POINT('Ctrl Pts',(-165.021947502421,58.300000000037,184.84898968561));
#89605=CARTESIAN_POINT('Ctrl Pts',(-168.264719930277,58.8,182.408084773135));
#89606=CARTESIAN_POINT('Ctrl Pts',(-168.526867773756,58.7999999999722,182.834115040067));
#89607=CARTESIAN_POINT('Ctrl Pts',(-168.526867773861,58.2999999999815,182.834115040249));
#89608=CARTESIAN_POINT('Ctrl Pts',(-169.390999188975,58.7999999999999,181.691812341728));
#89609=CARTESIAN_POINT('Ctrl Pts',(-169.666776786259,58.7999999999906,182.109235796414));
#89610=CARTESIAN_POINT('Ctrl Pts',(-169.666776786143,58.3000000000092,182.109235796277));
#89611=CARTESIAN_POINT('Ctrl Pts',(-171.029630345911,58.7999999999999,180.526399139192));
#89612=CARTESIAN_POINT('Ctrl Pts',(-171.32642510615,58.8000000000046,180.928874947422));
#89613=CARTESIAN_POINT('Ctrl Pts',(-171.326425106208,58.2999999999953,180.92887494749));
#89614=CARTESIAN_POINT('Ctrl Pts',(-171.567368036222,58.8,180.122746179185));
#89615=CARTESIAN_POINT('Ctrl Pts',(-171.871260701913,58.8000000000046,180.519901406522));
#89616=CARTESIAN_POINT('Ctrl Pts',(-171.871260701861,58.3,180.519901406445));
#89617=CARTESIAN_POINT('Ctrl Pts',(-172.624619471896,58.8,179.282785482643));
#89618=CARTESIAN_POINT('Ctrl Pts',(-172.942780916019,58.7999999999953,179.668604510607));
#89619=CARTESIAN_POINT('Ctrl Pts',(-172.942780916071,58.3,179.668604510684));
#89620=CARTESIAN_POINT('Ctrl Pts',(-173.142833366156,58.8,178.847331341283));
#89621=CARTESIAN_POINT('Ctrl Pts',(-173.468148508335,58.800000000007,179.227145347679));
#89622=CARTESIAN_POINT('Ctrl Pts',(-173.468148508321,58.3,179.227145347663));
#89623=CARTESIAN_POINT('Ctrl Pts',(-175.653687288211,58.8,176.613457905974));
#89624=CARTESIAN_POINT('Ctrl Pts',(-176.014168613236,58.799999999972,176.961985025883));
#89625=CARTESIAN_POINT('Ctrl Pts',(-176.014168613293,58.3,176.961985025947));
#89626=CARTESIAN_POINT('Ctrl Pts',(-177.428617853825,58.7999999999999,174.624131223718));
#89627=CARTESIAN_POINT('Ctrl Pts',(-177.815415056938,58.8000000000464,174.943121919096));
#89628=CARTESIAN_POINT('Ctrl Pts',(-177.81541505701,58.3000000000371,174.94312191921));
#89629=CARTESIAN_POINT('Ctrl Pts',(-179.362497837556,58.7999999999999,171.891096446713));
#89630=CARTESIAN_POINT('Ctrl Pts',(-179.77599160755,58.7999999999883,172.17235851032));
#89631=CARTESIAN_POINT('Ctrl Pts',(-179.775991607532,58.2999999999906,172.172358510292));
#89632=CARTESIAN_POINT('Ctrl Pts',(-179.735156702828,58.8,171.332276242436));
#89633=CARTESIAN_POINT('Ctrl Pts',(-180.153696573167,58.7999999999789,171.605961657972));
#89634=CARTESIAN_POINT('Ctrl Pts',(-180.153696573215,58.2999999999953,171.605961658012));
#89635=CARTESIAN_POINT('Ctrl Pts',(-180.452895188782,58.8,170.190776016648));
#89636=CARTESIAN_POINT('Ctrl Pts',(-180.880916991989,58.800000000021,170.449381248111));
#89637=CARTESIAN_POINT('Ctrl Pts',(-180.88091699194,58.3000000000046,170.449381248071));
#89638=CARTESIAN_POINT('Ctrl Pts',(-180.797963758657,58.8,169.607853241695));
#89639=CARTESIAN_POINT('Ctrl Pts',(-181.230420402717,58.7999999999766,169.858953973832));
#89640=CARTESIAN_POINT('Ctrl Pts',(-181.230420402812,58.2999999999906,169.858953973894));
#89641=CARTESIAN_POINT('Ctrl Pts',(-181.781931362112,58.8,167.84582021067));
#89642=CARTESIAN_POINT('Ctrl Pts',(-182.226654132377,58.8000000000467,168.074955464039));
#89643=CARTESIAN_POINT('Ctrl Pts',(-182.226654132187,58.3000000000186,168.074955463915));
#89644=CARTESIAN_POINT('Ctrl Pts',(-182.374255506228,58.8,166.646517916866));
#89645=CARTESIAN_POINT('Ctrl Pts',(-182.825829796625,58.8,166.861660004045));
#89646=CARTESIAN_POINT('Ctrl Pts',(-182.825829796819,58.3,166.861660004131));
#89647=CARTESIAN_POINT('Ctrl Pts',(-183.99092543293,58.8,162.986625821498));
#89648=CARTESIAN_POINT('Ctrl Pts',(-184.459874896285,58.8,163.162433189105));
#89649=CARTESIAN_POINT('Ctrl Pts',(-184.459874895897,58.3,163.162433188933));
#89650=CARTESIAN_POINT('Ctrl Pts',(-184.856296646016,58.8,160.464564288146));
#89651=CARTESIAN_POINT('Ctrl Pts',(-185.332658084315,58.8000000000093,160.617765879063));
#89652=CARTESIAN_POINT('Ctrl Pts',(-185.332658084617,58.2999999999814,160.617765879137));
#89653=CARTESIAN_POINT('Ctrl Pts',(-185.933727730562,58.8,156.59616119807));
#89654=CARTESIAN_POINT('Ctrl Pts',(-186.418046815945,58.7999999999953,156.720791693547));
#89655=CARTESIAN_POINT('Ctrl Pts',(-186.418046815794,58.3000000000093,156.72079169351));
#89656=CARTESIAN_POINT('Ctrl Pts',(-186.256430054963,58.8,155.289137032266));
#89657=CARTESIAN_POINT('Ctrl Pts',(-186.742866764348,58.7999999999813,155.405086705275));
#89658=CARTESIAN_POINT('Ctrl Pts',(-186.74286676451,58.3,155.405086705311));
#89659=CARTESIAN_POINT('Ctrl Pts',(-186.836507038269,58.8,152.668979197173));
#89660=CARTESIAN_POINT('Ctrl Pts',(-187.326429131997,58.8000000000186,152.769185688968));
#89661=CARTESIAN_POINT('Ctrl Pts',(-187.326429131835,58.3,152.769185688932));
#89662=CARTESIAN_POINT('Ctrl Pts',(-187.093966794783,58.8,151.356609778289));
#89663=CARTESIAN_POINT('Ctrl Pts',(-187.585258126186,58.7999999999722,151.449750314483));
#89664=CARTESIAN_POINT('Ctrl Pts',(-187.585258126307,58.2999999999814,151.449750314505));
#89665=CARTESIAN_POINT('Ctrl Pts',(-187.788398583071,58.8,147.414021296038));
#89666=CARTESIAN_POINT('Ctrl Pts',(-188.283075769721,58.8000000000555,147.487938873115));
#89667=CARTESIAN_POINT('Ctrl Pts',(-188.283075769478,58.300000000037,147.487938873072));
#89668=CARTESIAN_POINT('Ctrl Pts',(-188.148412170526,58.8,144.778391543178));
#89669=CARTESIAN_POINT('Ctrl Pts',(-188.644410165613,58.7999999999447,144.842102846955));
#89670=CARTESIAN_POINT('Ctrl Pts',(-188.644410165759,58.2999999999631,144.842102846971));
#89671=CARTESIAN_POINT('Ctrl Pts',(-188.735101605106,58.8,139.49775750896));
#89672=CARTESIAN_POINT('Ctrl Pts',(-189.232988329617,58.8000000000553,139.544468866576));
#89673=CARTESIAN_POINT('Ctrl Pts',(-189.232988329472,58.3000000000369,139.54446886656));
#89674=CARTESIAN_POINT('Ctrl Pts',(-188.961273483377,58.8,136.852717795317));
#89675=CARTESIAN_POINT('Ctrl Pts',(-189.459709168613,58.7999999999723,136.892642646102));
#89676=CARTESIAN_POINT('Ctrl Pts',(-189.459709168717,58.2999999999815,136.892642646109));
#89677=CARTESIAN_POINT('Ctrl Pts',(-189.325139639208,58.8,131.556417805101));
#89678=CARTESIAN_POINT('Ctrl Pts',(-189.824352296292,58.8000000000276,131.585033344344));
#89679=CARTESIAN_POINT('Ctrl Pts',(-189.824352296188,58.3000000000184,131.585033344337));
#89680=CARTESIAN_POINT('Ctrl Pts',(-189.462571780471,58.7999999999999,128.905139098825));
#89681=CARTESIAN_POINT('Ctrl Pts',(-189.962004740431,58.7999999999078,128.929238461044));
#89682=CARTESIAN_POINT('Ctrl Pts',(-189.962004740442,58.2999999999631,128.929238461044));
#89683=CARTESIAN_POINT('Ctrl Pts',(-189.678761610221,58.7999999999999,123.598456482345));
#89684=CARTESIAN_POINT('Ctrl Pts',(-190.178499841919,58.800000000092,123.615062522244));
#89685=CARTESIAN_POINT('Ctrl Pts',(-190.178499841907,58.3000000000368,123.615062522244));
#89686=CARTESIAN_POINT('Ctrl Pts',(-189.757373218151,58.7999999999999,120.943042302021));
#89687=CARTESIAN_POINT('Ctrl Pts',(-190.257193263786,58.8000000000552,120.956675467134));
#89688=CARTESIAN_POINT('Ctrl Pts',(-190.257193263798,58.3000000000368,120.956675467134));
#89689=CARTESIAN_POINT('Ctrl Pts',(-189.935893374821,58.7999999999999,112.972770159095));
#89690=CARTESIAN_POINT('Ctrl Pts',(-190.435877163826,58.7999999998893,112.979092781064));
#89691=CARTESIAN_POINT('Ctrl Pts',(-190.435877163802,58.2999999999262,112.979092781063));
#89692=CARTESIAN_POINT('Ctrl Pts',(-189.980251348956,58.8,107.653938592502));
#89693=CARTESIAN_POINT('Ctrl Pts',(-190.480241583042,58.7999999991693,107.657514868693));
#89694=CARTESIAN_POINT('Ctrl Pts',(-190.480241583535,58.299999999557,107.657514868695));
#89695=CARTESIAN_POINT('Ctrl Pts',(-189.999800857363,58.8,102.333498885934));
#89696=CARTESIAN_POINT('Ctrl Pts',(-190.499797482064,58.8,102.335336081498));
#89697=CARTESIAN_POINT('Ctrl Pts',(-190.499797482064,58.3,102.335336081498));
#89698=CARTESIAN_POINT('Origin',(125.29348064571,25.4505574462982,228.3));
#89699=CARTESIAN_POINT('',(121.237845913371,25.4505574462982,229.));
#89700=CARTESIAN_POINT('',(120.537845913371,25.4505574462982,228.3));
#89701=CARTESIAN_POINT('Origin',(121.237845913371,25.4505574462982,228.3));
#89702=CARTESIAN_POINT('',(130.049115378049,25.4505574462982,228.3));
#89703=CARTESIAN_POINT('Origin',(125.29348064571,25.4505574462982,228.3));
#89704=CARTESIAN_POINT('',(129.349115378049,25.4505574462982,229.));
#89705=CARTESIAN_POINT('Origin',(129.349115378049,25.4505574462982,228.3));
#89706=CARTESIAN_POINT('Origin',(125.29348064571,25.4505574462982,229.));
#89707=CARTESIAN_POINT('Origin',(129.349115378049,25.4505574462982,228.3));
#89708=CARTESIAN_POINT('',(130.049115378049,53.4601166829598,228.3));
#89709=CARTESIAN_POINT('',(129.349115378049,53.4601166829598,229.));
#89710=CARTESIAN_POINT('Origin',(129.349115378049,53.4601166829598,228.3));
#89711=CARTESIAN_POINT('',(129.349115378049,25.4505574462982,229.));
#89712=CARTESIAN_POINT('',(130.049115378049,25.4505574462982,228.3));
#89713=CARTESIAN_POINT('Origin',(121.237845913371,25.4505574462982,228.3));
#89714=CARTESIAN_POINT('',(121.237845913371,53.4601166829598,229.));
#89715=CARTESIAN_POINT('',(120.537845913371,53.4601166829598,228.3));
#89716=CARTESIAN_POINT('Origin',(121.237845913371,53.4601166829598,228.3));
#89717=CARTESIAN_POINT('',(120.537845913371,25.4505574462982,228.3));
#89718=CARTESIAN_POINT('',(121.237845913371,25.4505574462982,229.));
#89719=CARTESIAN_POINT('Origin',(125.29348064571,53.4601166829598,228.3));
#89720=CARTESIAN_POINT('Origin',(125.29348064571,53.4601166829598,228.3));
#89721=CARTESIAN_POINT('Origin',(125.29348064571,53.4601166829598,229.));
#89722=CARTESIAN_POINT('Origin',(119.837845913371,51.61032741828,227.));
#89723=CARTESIAN_POINT('',(120.537845913371,51.61032741828,226.3));
#89724=CARTESIAN_POINT('Origin',(119.837845913371,51.61032741828,226.3));
#89725=CARTESIAN_POINT('',(120.537845913371,51.61032741828,202.7));
#89726=CARTESIAN_POINT('',(120.537845913371,51.61032741828,202.));
#89727=CARTESIAN_POINT('Origin',(119.837845913371,51.61032741828,202.7));
#89728=CARTESIAN_POINT('Ctrl Pts',(119.980756553526,50.9250708612662,202.7));
#89729=CARTESIAN_POINT('Ctrl Pts',(120.537845913371,51.0412521604076,202.7));
#89730=CARTESIAN_POINT('Ctrl Pts',(120.537845913371,51.61032741828,202.7));
#89731=CARTESIAN_POINT('Ctrl Pts',(119.980756569514,50.9250708646006,202.515401659683));
#89732=CARTESIAN_POINT('Ctrl Pts',(120.53784592438,51.0412521623395,202.592003939902));
#89733=CARTESIAN_POINT('Ctrl Pts',(120.537845913371,51.6103274217032,202.607700830635));
#89734=CARTESIAN_POINT('Ctrl Pts',(120.016933348296,50.9326865962307,202.330393020895));
#89735=CARTESIAN_POINT('Ctrl Pts',(120.563210336327,51.0457300061094,202.483460486543));
#89736=CARTESIAN_POINT('Ctrl Pts',(120.556420880425,51.6181480150106,202.515196509376));
#89737=CARTESIAN_POINT('Ctrl Pts',(120.12071246513,50.9538824639444,202.075296318228));
#89738=CARTESIAN_POINT('Ctrl Pts',(120.632852328253,51.0577402793023,202.34004784784));
#89739=CARTESIAN_POINT('Ctrl Pts',(120.609706255931,51.6399140437658,202.38764815965));
#89740=CARTESIAN_POINT('Ctrl Pts',(120.163000282663,50.9624493988279,201.994724706521));
#89741=CARTESIAN_POINT('Ctrl Pts',(120.661125768475,51.0625838875446,202.295519980409));
#89742=CARTESIAN_POINT('Ctrl Pts',(120.631418928709,51.648711427579,202.347362353776));
#89743=CARTESIAN_POINT('Ctrl Pts',(120.262801434937,50.9823166185813,201.842380942087));
#89744=CARTESIAN_POINT('Ctrl Pts',(120.726488287769,51.0736408783625,202.213784518412));
#89745=CARTESIAN_POINT('Ctrl Pts',(120.682661813548,51.6691130682172,202.271190470529));
#89746=CARTESIAN_POINT('Ctrl Pts',(120.320608134591,50.9936686129295,201.770645389731));
#89747=CARTESIAN_POINT('Ctrl Pts',(120.763864029259,51.0798986385742,202.176621792572));
#89748=CARTESIAN_POINT('Ctrl Pts',(120.712342654789,51.6807704288856,202.235322694426));
#89749=CARTESIAN_POINT('Ctrl Pts',(120.509667057382,51.0299919759325,201.57792765521));
#89750=CARTESIAN_POINT('Ctrl Pts',(120.883631159183,51.0996738601009,202.080620018702));
#89751=CARTESIAN_POINT('Ctrl Pts',(120.809414931026,51.7180708774407,202.138963828484));
#89752=CARTESIAN_POINT('Ctrl Pts',(120.661556892567,51.0581478200239,201.474556554105));
#89753=CARTESIAN_POINT('Ctrl Pts',(120.976009362001,51.1145360804081,202.03632174739));
#89754=CARTESIAN_POINT('Ctrl Pts',(120.887402742536,51.746984107053,202.087278277309));
#89755=CARTESIAN_POINT('Ctrl Pts',(120.988479548833,51.1151316286093,201.336326839815));
#89756=CARTESIAN_POINT('Ctrl Pts',(121.161594565797,51.1436937459234,201.989169936985));
#89757=CARTESIAN_POINT('Ctrl Pts',(121.055261129938,51.805500760816,202.018163419651));
#89758=CARTESIAN_POINT('Ctrl Pts',(121.168035486324,51.1446870647112,201.300000006569));
#89759=CARTESIAN_POINT('Ctrl Pts',(121.257345167804,51.1584002645244,201.986437757956));
#89760=CARTESIAN_POINT('Ctrl Pts',(121.147464824898,51.8358545236066,202.));
#89761=CARTESIAN_POINT('Ctrl Pts',(121.344083479533,51.1717186376762,201.3));
#89762=CARTESIAN_POINT('Ctrl Pts',(121.344083479533,51.1717186376762,202.));
#89763=CARTESIAN_POINT('Ctrl Pts',(121.237845913371,51.8636099438334,202.));
#89764=CARTESIAN_POINT('',(121.237845913371,51.8636099438334,202.));
#89765=CARTESIAN_POINT('Origin',(121.237845913371,51.8636099438334,201.3));
#89766=CARTESIAN_POINT('Ctrl Pts',(120.537845913371,51.61032741828,202.7));
#89767=CARTESIAN_POINT('Ctrl Pts',(120.537845913371,51.61032741828,202.66960977505));
#89768=CARTESIAN_POINT('Ctrl Pts',(120.539855658745,51.6111733231747,202.639425914894));
#89769=CARTESIAN_POINT('Ctrl Pts',(120.54375094998,51.612797640954,202.60963193772));
#89770=CARTESIAN_POINT('Ctrl Pts',(120.547805934794,51.6144885501911,202.578616509673));
#89771=CARTESIAN_POINT('Ctrl Pts',(120.553904211385,51.6170230548541,202.548022544351));
#89772=CARTESIAN_POINT('Ctrl Pts',(120.561957633332,51.620347527652,202.51804567938));
#89773=CARTESIAN_POINT('Ctrl Pts',(120.57001105528,51.6236720004499,202.48806881441));
#89774=CARTESIAN_POINT('Ctrl Pts',(120.580019901367,51.6277866249341,202.458707903137));
#89775=CARTESIAN_POINT('Ctrl Pts',(120.591944490529,51.6326578298738,202.430164212952));
#89776=CARTESIAN_POINT('Ctrl Pts',(120.592593281725,51.632922861636,202.428611212287));
#89777=CARTESIAN_POINT('Ctrl Pts',(120.593247373301,51.6331899634816,202.427061118066));
#89778=CARTESIAN_POINT('Ctrl Pts',(120.593906770483,51.633459131624,202.425513916105));
#89779=CARTESIAN_POINT('Ctrl Pts',(120.611371061272,51.6405881137296,202.384535905139));
#89780=CARTESIAN_POINT('Ctrl Pts',(120.632459420528,51.6491254533931,202.345815672698));
#89781=CARTESIAN_POINT('Ctrl Pts',(120.65704038842,51.6589119690931,202.309276386448));
#89782=CARTESIAN_POINT('Ctrl Pts',(120.678024081841,51.667266288012,202.2780844015));
#89783=CARTESIAN_POINT('Ctrl Pts',(120.701651295733,51.6765655446655,202.248497154293));
#89784=CARTESIAN_POINT('Ctrl Pts',(120.727118155272,51.6864222072939,202.221305435165));
#89785=CARTESIAN_POINT('Ctrl Pts',(120.732887337535,51.6886551046452,202.215145508636));
#89786=CARTESIAN_POINT('Ctrl Pts',(120.738751061304,51.6909166731422,202.209108367204));
#89787=CARTESIAN_POINT('Ctrl Pts',(120.744700214597,51.6932025229427,202.203202939035));
#89788=CARTESIAN_POINT('Ctrl Pts',(120.746092792191,51.693737594584,202.201820596616));
#89789=CARTESIAN_POINT('Ctrl Pts',(120.74749123962,51.6942744329583,202.200444341435));
#89790=CARTESIAN_POINT('Ctrl Pts',(120.748895476413,51.6948129989188,202.199074212284));
#89791=CARTESIAN_POINT('Ctrl Pts',(120.772718863232,51.7039499658979,202.175829473978));
#89792=CARTESIAN_POINT('Ctrl Pts',(120.798162272373,51.7135669523555,202.154387377056));
#89793=CARTESIAN_POINT('Ctrl Pts',(120.824895788136,51.7234982117892,202.134874709475));
#89794=CARTESIAN_POINT('Ctrl Pts',(120.85282975049,51.733875426279,202.114485841566));
#89795=CARTESIAN_POINT('Ctrl Pts',(120.882173281514,51.7445963236697,202.096202574251));
#89796=CARTESIAN_POINT('Ctrl Pts',(120.912593768197,51.7554862438252,202.08020234405));
#89797=CARTESIAN_POINT('Ctrl Pts',(120.931770422228,51.7623510988628,202.070116020245));
#89798=CARTESIAN_POINT('Ctrl Pts',(120.951375867509,51.7692833814873,202.060937650301));
#89799=CARTESIAN_POINT('Ctrl Pts',(120.971332224645,51.7762404987801,202.052720729726));
#89800=CARTESIAN_POINT('Ctrl Pts',(121.00280605992,51.7872128000952,202.039761550711));
#89801=CARTESIAN_POINT('Ctrl Pts',(121.035480957547,51.7983527205708,202.029088055337));
#89802=CARTESIAN_POINT('Ctrl Pts',(121.068916659086,51.8094930078735,202.020802179907));
#89803=CARTESIAN_POINT('Ctrl Pts',(121.09993022458,51.8198262748305,202.013116546632));
#89804=CARTESIAN_POINT('Ctrl Pts',(121.131599665853,51.8301602846134,202.007485376878));
#89805=CARTESIAN_POINT('Ctrl Pts',(121.163565450452,51.8403542638175,202.004031182709));
#89806=CARTESIAN_POINT('Ctrl Pts',(121.188207937351,51.8482128226525,202.001368337558));
#89807=CARTESIAN_POINT('Ctrl Pts',(121.213026553804,51.8559880865824,202.));
#89808=CARTESIAN_POINT('Ctrl Pts',(121.237845913371,51.8636099438334,202.));
#89809=CARTESIAN_POINT('Ctrl Pts',(120.537845913371,51.61032741828,226.3));
#89810=CARTESIAN_POINT('Ctrl Pts',(120.537845913371,51.0412521604076,226.3));
#89811=CARTESIAN_POINT('Ctrl Pts',(119.980756553526,50.9250708612662,226.3));
#89812=CARTESIAN_POINT('Ctrl Pts',(120.537845913371,51.6103274014729,226.485230527047));
#89813=CARTESIAN_POINT('Ctrl Pts',(120.537845913371,51.0412521492249,226.40834300785));
#89814=CARTESIAN_POINT('Ctrl Pts',(119.980756550258,50.9250708605847,226.392615262739));
#89815=CARTESIAN_POINT('Ctrl Pts',(120.537845913371,51.5720784940094,226.670993650709));
#89816=CARTESIAN_POINT('Ctrl Pts',(120.537845913372,51.0154718436456,226.517300435127));
#89817=CARTESIAN_POINT('Ctrl Pts',(119.977147933168,50.905195322387,226.485496826417));
#89818=CARTESIAN_POINT('Ctrl Pts',(120.537845913371,51.4624739877832,226.926759478812));
#89819=CARTESIAN_POINT('Ctrl Pts',(120.53784591337,50.9435849182146,226.662349946297));
#89820=CARTESIAN_POINT('Ctrl Pts',(119.966685777936,50.8482018526639,226.613379738875));
#89821=CARTESIAN_POINT('Ctrl Pts',(120.537845913371,51.4178168105653,227.007514343431));
#89822=CARTESIAN_POINT('Ctrl Pts',(120.537845913371,50.9143149102838,226.707540176998));
#89823=CARTESIAN_POINT('Ctrl Pts',(119.962410036061,50.8249762936204,226.653757171192));
#89824=CARTESIAN_POINT('Ctrl Pts',(120.537845913371,51.312438648417,227.160123469212));
#89825=CARTESIAN_POINT('Ctrl Pts',(120.537845913371,50.8461079001102,226.790822267366));
#89826=CARTESIAN_POINT('Ctrl Pts',(119.952253732179,50.7701490700559,226.73006173513));
#89827=CARTESIAN_POINT('Ctrl Pts',(120.537845913371,51.2514663528816,227.23186217591));
#89828=CARTESIAN_POINT('Ctrl Pts',(120.537845913371,50.8069032828533,226.828843822385));
#89829=CARTESIAN_POINT('Ctrl Pts',(119.946347697567,50.7384162488755,226.765931088417));
#89830=CARTESIAN_POINT('Ctrl Pts',(120.537845913371,51.0522284602922,227.424379532362));
#89831=CARTESIAN_POINT('Ctrl Pts',(120.537845913371,50.6803088645031,226.927203621114));
#89832=CARTESIAN_POINT('Ctrl Pts',(119.926892953773,50.6346729547807,226.862189765258));
#89833=CARTESIAN_POINT('Ctrl Pts',(120.537845913371,50.8924503496942,227.527224116548));
#89834=CARTESIAN_POINT('Ctrl Pts',(120.537845913373,50.5809974336902,226.973017056931));
#89835=CARTESIAN_POINT('Ctrl Pts',(119.911093129127,50.5514121280869,226.913612058182));
#89836=CARTESIAN_POINT('Ctrl Pts',(120.537845913371,50.549650402769,227.664303698141));
#89837=CARTESIAN_POINT('Ctrl Pts',(120.537845913368,50.378975163546,227.019149612712));
#89838=CARTESIAN_POINT('Ctrl Pts',(119.876462473964,50.3725357589363,226.982151849163));
#89839=CARTESIAN_POINT('Ctrl Pts',(120.537845913371,50.3620142055013,227.699999994234));
#89840=CARTESIAN_POINT('Ctrl Pts',(120.537845913371,50.2731525920023,227.019033760568));
#89841=CARTESIAN_POINT('Ctrl Pts',(119.857153207514,50.2745131115586,227.));
#89842=CARTESIAN_POINT('Ctrl Pts',(120.537845913371,50.1784824778425,227.7));
#89843=CARTESIAN_POINT('Ctrl Pts',(120.537845913371,50.1784824778428,227.));
#89844=CARTESIAN_POINT('Ctrl Pts',(119.83784591337,50.1784824778428,227.));
#89845=CARTESIAN_POINT('',(120.537845913371,50.178482477843,227.7));
#89846=CARTESIAN_POINT('Origin',(119.837845913371,50.178482477843,227.7));
#89847=CARTESIAN_POINT('Ctrl Pts',(120.537845913371,50.178482477843,227.7));
#89848=CARTESIAN_POINT('Ctrl Pts',(120.537845913371,50.2266182247457,227.699999998488));
#89849=CARTESIAN_POINT('Ctrl Pts',(120.537845913371,50.2746956243944,227.697548388819));
#89850=CARTESIAN_POINT('Ctrl Pts',(120.53784591337,50.3224646868022,227.69277495358));
#89851=CARTESIAN_POINT('Ctrl Pts',(120.53784591337,50.3716410766915,227.687860887852));
#89852=CARTESIAN_POINT('Ctrl Pts',(120.537845913368,50.4204918776408,227.680486173035));
#89853=CARTESIAN_POINT('Ctrl Pts',(120.537845913367,50.4687648579522,227.670738951763));
#89854=CARTESIAN_POINT('Ctrl Pts',(120.537845913365,50.5174165969936,227.660915251991));
#89855=CARTESIAN_POINT('Ctrl Pts',(120.537845913364,50.5654827340969,227.648681512488));
#89856=CARTESIAN_POINT('Ctrl Pts',(120.537845913363,50.6127063716968,227.634075950352));
#89857=CARTESIAN_POINT('Ctrl Pts',(120.537845913363,50.6493708477602,227.622736178353));
#89858=CARTESIAN_POINT('Ctrl Pts',(120.537845913364,50.6855276842963,227.609965612803));
#89859=CARTESIAN_POINT('Ctrl Pts',(120.537845913366,50.7210494651645,227.595761629006));
#89860=CARTESIAN_POINT('Ctrl Pts',(120.537845913366,50.7215096846164,227.595577602488));
#89861=CARTESIAN_POINT('Ctrl Pts',(120.537845913366,50.7219698305945,227.595393324582));
#89862=CARTESIAN_POINT('Ctrl Pts',(120.537845913366,50.7224299029115,227.595208795376));
#89863=CARTESIAN_POINT('Ctrl Pts',(120.537845913373,50.8577361254776,227.540939175357));
#89864=CARTESIAN_POINT('Ctrl Pts',(120.537845913368,50.9857915093738,227.465273532112));
#89865=CARTESIAN_POINT('Ctrl Pts',(120.537845913369,51.0990063730544,227.37257058707));
#89866=CARTESIAN_POINT('Ctrl Pts',(120.537845913369,51.1287591671713,227.348208312116));
#89867=CARTESIAN_POINT('Ctrl Pts',(120.53784591337,51.1574871836322,227.322669608678));
#89868=CARTESIAN_POINT('Ctrl Pts',(120.53784591337,51.1850531176328,227.296034002577));
#89869=CARTESIAN_POINT('Ctrl Pts',(120.53784591337,51.1852908868274,227.2958042579));
#89870=CARTESIAN_POINT('Ctrl Pts',(120.53784591337,51.1855285862015,227.295574416347));
#89871=CARTESIAN_POINT('Ctrl Pts',(120.53784591337,51.1857662156247,227.295344478058));
#89872=CARTESIAN_POINT('Ctrl Pts',(120.537845913371,51.2518975783998,227.231353528472));
#89873=CARTESIAN_POINT('Ctrl Pts',(120.537845913371,51.3126273026802,227.159850257429));
#89874=CARTESIAN_POINT('Ctrl Pts',(120.53784591337,51.3651275337233,227.083818771142));
#89875=CARTESIAN_POINT('Ctrl Pts',(120.53784591337,51.3652690148093,227.083613876477));
#89876=CARTESIAN_POINT('Ctrl Pts',(120.53784591337,51.3654104379503,227.083408949767));
#89877=CARTESIAN_POINT('Ctrl Pts',(120.53784591337,51.3655518031444,227.08320399101));
#89878=CARTESIAN_POINT('Ctrl Pts',(120.53784591337,51.418056152811,227.007080400097));
#89879=CARTESIAN_POINT('Ctrl Pts',(120.53784591337,51.4625703069915,226.926533129112));
#89880=CARTESIAN_POINT('Ctrl Pts',(120.53784591337,51.4990085348243,226.841504079202));
#89881=CARTESIAN_POINT('Ctrl Pts',(120.53784591337,51.4990739390667,226.841351457603));
#89882=CARTESIAN_POINT('Ctrl Pts',(120.53784591337,51.4991393154205,226.841198823767));
#89883=CARTESIAN_POINT('Ctrl Pts',(120.53784591337,51.4992046638834,226.841046177703));
#89884=CARTESIAN_POINT('Ctrl Pts',(120.537845913371,51.5143302327706,226.805714687968));
#89885=CARTESIAN_POINT('Ctrl Pts',(120.537845913371,51.5280125310827,226.769597689428));
#89886=CARTESIAN_POINT('Ctrl Pts',(120.537845913371,51.5401513369114,226.7329742214));
#89887=CARTESIAN_POINT('Ctrl Pts',(120.537845913371,51.552355291154,226.6961541969));
#89888=CARTESIAN_POINT('Ctrl Pts',(120.537845913371,51.5629989358661,226.658823004492));
#89889=CARTESIAN_POINT('Ctrl Pts',(120.537845913371,51.5720303361862,226.621280362417));
#89890=CARTESIAN_POINT('Ctrl Pts',(120.537845913371,51.5756770373127,226.606121384818));
#89891=CARTESIAN_POINT('Ctrl Pts',(120.537845913371,51.5790614626629,226.590928052307));
#89892=CARTESIAN_POINT('Ctrl Pts',(120.537845913371,51.5821825826778,226.575720403825));
#89893=CARTESIAN_POINT('Ctrl Pts',(120.537845913371,51.5900124195483,226.537569545728));
#89894=CARTESIAN_POINT('Ctrl Pts',(120.537845913371,51.5962282679499,226.499143671121));
#89895=CARTESIAN_POINT('Ctrl Pts',(120.537845913371,51.6008158826798,226.460436009908));
#89896=CARTESIAN_POINT('Ctrl Pts',(120.537845913371,51.6053222463237,226.422413898744));
#89897=CARTESIAN_POINT('Ctrl Pts',(120.537845913371,51.608257592452,226.384119167664));
#89898=CARTESIAN_POINT('Ctrl Pts',(120.537845913371,51.6095585651145,226.345544518822));
#89899=CARTESIAN_POINT('Ctrl Pts',(120.537845913371,51.6100691246589,226.330406110686));
#89900=CARTESIAN_POINT('Ctrl Pts',(120.537845913371,51.6103274168984,226.315224640044));
#89901=CARTESIAN_POINT('Ctrl Pts',(120.537845913371,51.6103274182798,226.3));
#89902=CARTESIAN_POINT('Origin',(121.237845913371,25.4505574462982,202.7));
#89903=CARTESIAN_POINT('',(120.537845913371,53.4601166829598,202.7));
#89904=CARTESIAN_POINT('',(121.237845913371,53.4601166829598,202.));
#89905=CARTESIAN_POINT('Origin',(121.237845913371,53.4601166829598,202.7));
#89906=CARTESIAN_POINT('',(121.237845913371,53.4601166829598,202.));
#89907=CARTESIAN_POINT('',(120.537845913371,51.0349239481607,202.7));
#89908=CARTESIAN_POINT('Origin',(125.29348064571,25.4505574462982,201.3));
#89909=CARTESIAN_POINT('',(129.349115378049,51.8636099438334,202.));
#89910=CARTESIAN_POINT('Origin',(129.349115378049,51.8636099438334,201.3));
#89911=CARTESIAN_POINT('Origin',(125.29348064571,25.4505574462982,202.));
#89912=CARTESIAN_POINT('Origin',(119.837845913371,25.4505574462982,227.7));
#89913=CARTESIAN_POINT('',(119.837845913371,25.4505574462982,227.));
#89914=CARTESIAN_POINT('',(120.537845913371,25.4505574462982,227.7));
#89915=CARTESIAN_POINT('Origin',(119.837845913371,25.4505574462982,227.7));
#89916=CARTESIAN_POINT('',(120.537845913371,25.4505574462982,227.7));
#89917=CARTESIAN_POINT('',(119.837845913371,51.0349239481607,227.));
#89918=CARTESIAN_POINT('Origin',(125.29348064571,53.4601166829598,202.7));
#89919=CARTESIAN_POINT('',(130.049115378049,53.4601166829598,202.7));
#89920=CARTESIAN_POINT('',(129.349115378049,53.4601166829598,202.));
#89921=CARTESIAN_POINT('Origin',(129.349115378049,53.4601166829598,202.7));
#89922=CARTESIAN_POINT('Origin',(125.29348064571,53.4601166829598,202.));
#89923=CARTESIAN_POINT('Origin',(125.29348064571,53.4601166829598,202.7));
#89924=CARTESIAN_POINT('Ctrl Pts',(129.242877811887,51.1717186376762,201.3));
#89925=CARTESIAN_POINT('Ctrl Pts',(129.242877811887,51.1717186376762,202.));
#89926=CARTESIAN_POINT('Ctrl Pts',(129.349115378049,51.8636099438334,202.));
#89927=CARTESIAN_POINT('Ctrl Pts',(129.420790531699,51.1444007422584,201.30000001605));
#89928=CARTESIAN_POINT('Ctrl Pts',(129.330552739425,51.1582564503628,201.986291315068));
#89929=CARTESIAN_POINT('Ctrl Pts',(129.440457412025,51.8355594232403,202.));
#89930=CARTESIAN_POINT('Ctrl Pts',(129.598075339384,51.1152070969532,201.336045209247));
#89931=CARTESIAN_POINT('Ctrl Pts',(129.4251056608,51.1437356540326,201.989044028215));
#89932=CARTESIAN_POINT('Ctrl Pts',(129.531491494697,51.8055782590138,202.018022602192));
#89933=CARTESIAN_POINT('Ctrl Pts',(129.844929320498,51.0721725887805,201.440585262543));
#89934=CARTESIAN_POINT('Ctrl Pts',(129.566019525609,51.1215950595266,202.024935223531));
#89935=CARTESIAN_POINT('Ctrl Pts',(129.658238631884,51.7613861374496,202.070292632487));
#89936=CARTESIAN_POINT('Ctrl Pts',(129.922998586318,51.0581555745418,201.483235952924));
#89937=CARTESIAN_POINT('Ctrl Pts',(129.611787002084,51.1143254180597,202.041693414839));
#89938=CARTESIAN_POINT('Ctrl Pts',(129.698323284282,51.7469920688305,202.091617977236));
#89939=CARTESIAN_POINT('Ctrl Pts',(130.070819619104,51.0309904096655,201.584008547698));
#89940=CARTESIAN_POINT('Ctrl Pts',(129.700624875494,51.1000325324506,202.085699650362));
#89941=CARTESIAN_POINT('Ctrl Pts',(129.774221971894,51.719096170358,202.142004273075));
#89942=CARTESIAN_POINT('Ctrl Pts',(130.141021021261,51.0177501887032,201.642790906908));
#89943=CARTESIAN_POINT('Ctrl Pts',(129.744060773163,51.0929493134279,202.113213517417));
#89944=CARTESIAN_POINT('Ctrl Pts',(129.810266870854,51.705499790411,202.171395452989));
#89945=CARTESIAN_POINT('Ctrl Pts',(130.330155491038,50.981406690983,201.835877820745));
#89946=CARTESIAN_POINT('Ctrl Pts',(129.862797424543,51.0733422962284,202.208553654803));
#89947=CARTESIAN_POINT('Ctrl Pts',(129.907377934003,51.6681786657293,202.267938911302));
#89948=CARTESIAN_POINT('Ctrl Pts',(130.432435875125,50.9607892587758,201.991913652187));
#89949=CARTESIAN_POINT('Ctrl Pts',(129.931172038655,51.0616962900198,202.292657911015));
#89950=CARTESIAN_POINT('Ctrl Pts',(129.959893782294,51.6470066287864,202.345956826036));
#89951=CARTESIAN_POINT('Ctrl Pts',(130.569841134829,50.9327239155203,202.330202935899));
#89952=CARTESIAN_POINT('Ctrl Pts',(130.023631529767,51.0457502346248,202.483369876793));
#89953=CARTESIAN_POINT('Ctrl Pts',(130.030444491613,51.6181863382183,202.515101468007));
#89954=CARTESIAN_POINT('Ctrl Pts',(130.606204734282,50.9250708620194,202.516399404814));
#89955=CARTESIAN_POINT('Ctrl Pts',(130.049115375546,51.0412521608442,202.592582962827));
#89956=CARTESIAN_POINT('Ctrl Pts',(130.049115378049,51.6103274190584,202.60819970236));
#89957=CARTESIAN_POINT('Ctrl Pts',(130.606204737894,50.9250708612662,202.7));
#89958=CARTESIAN_POINT('Ctrl Pts',(130.049115378049,51.0412521604076,202.7));
#89959=CARTESIAN_POINT('Ctrl Pts',(130.049115378049,51.61032741828,202.7));
#89960=CARTESIAN_POINT('',(130.049115378049,51.61032741828,202.7));
#89961=CARTESIAN_POINT('Origin',(130.749115378049,51.61032741828,202.7));
#89962=CARTESIAN_POINT('Ctrl Pts',(129.349115378049,51.8636099438334,202.));
#89963=CARTESIAN_POINT('Ctrl Pts',(129.378353274608,51.8546311836304,202.));
#89964=CARTESIAN_POINT('Ctrl Pts',(129.407352909326,51.8455186460904,202.001842190722));
#89965=CARTESIAN_POINT('Ctrl Pts',(129.436016335062,51.8363253799306,202.005435824546));
#89966=CARTESIAN_POINT('Ctrl Pts',(129.466313728877,51.8266080485878,202.009234314657));
#89967=CARTESIAN_POINT('Ctrl Pts',(129.496236566828,51.8168001521295,202.014989357515));
#89968=CARTESIAN_POINT('Ctrl Pts',(129.525671916517,51.8069563789023,202.022654975898));
#89969=CARTESIAN_POINT('Ctrl Pts',(129.555107266207,51.7971126056752,202.03032059428));
#89970=CARTESIAN_POINT('Ctrl Pts',(129.584056310451,51.7872324900621,202.039897017501));
#89971=CARTESIAN_POINT('Ctrl Pts',(129.612391438466,51.7773694907784,202.05139719529));
#89972=CARTESIAN_POINT('Ctrl Pts',(129.613592056781,51.7769515749824,202.051884481745));
#89973=CARTESIAN_POINT('Ctrl Pts',(129.614791403714,51.7765337478366,202.052375163507));
#89974=CARTESIAN_POINT('Ctrl Pts',(129.615989462678,51.7761160158889,202.052869238133));
#89975=CARTESIAN_POINT('Ctrl Pts',(129.658186901675,51.7614028682804,202.070271289727));
#89976=CARTESIAN_POINT('Ctrl Pts',(129.698259377414,51.7470135279152,202.091575579855));
#89977=CARTESIAN_POINT('Ctrl Pts',(129.736272329953,51.7330417822806,202.11681092723));
#89978=CARTESIAN_POINT('Ctrl Pts',(129.768808503909,51.7210830388506,202.138410450477));
#89979=CARTESIAN_POINT('Ctrl Pts',(129.800007889183,51.7093596806358,202.16313533375));
#89980=CARTESIAN_POINT('Ctrl Pts',(129.828750982204,51.6983779810147,202.190153705326));
#89981=CARTESIAN_POINT('Ctrl Pts',(129.831763959202,51.6972268311251,202.192985889462));
#89982=CARTESIAN_POINT('Ctrl Pts',(129.834749901387,51.6960838481987,202.195843270102));
#89983=CARTESIAN_POINT('Ctrl Pts',(129.837707485871,51.694949628585,202.198724884211));
#89984=CARTESIAN_POINT('Ctrl Pts',(129.839359638223,51.6943160359987,202.200334598338));
#89985=CARTESIAN_POINT('Ctrl Pts',(129.841002890048,51.693685195333,202.201951824494));
#89986=CARTESIAN_POINT('Ctrl Pts',(129.842637012104,51.6930572101032,202.203576393868));
#89987=CARTESIAN_POINT('Ctrl Pts',(129.872259007364,51.6816736200997,202.233025226127));
#89988=CARTESIAN_POINT('Ctrl Pts',(129.899402602918,51.6710350326229,202.265409408267));
#89989=CARTESIAN_POINT('Ctrl Pts',(129.923562110217,51.6614414622518,202.300131331105));
#89990=CARTESIAN_POINT('Ctrl Pts',(129.945932245253,51.6525584390168,202.332281577094));
#89991=CARTESIAN_POINT('Ctrl Pts',(129.965744082943,51.6445712156073,202.366436892053));
#89992=CARTESIAN_POINT('Ctrl Pts',(129.982555408054,51.637736668221,202.402115810062));
#89993=CARTESIAN_POINT('Ctrl Pts',(129.986969969209,51.6359419538121,202.411484896942));
#89994=CARTESIAN_POINT('Ctrl Pts',(129.99117738931,51.6342268363493,202.420958971512));
#89995=CARTESIAN_POINT('Ctrl Pts',(129.995169129062,51.6325962227829,202.430529128101));
#89996=CARTESIAN_POINT('Ctrl Pts',(130.009842100651,51.6266023584496,202.465707432407));
#89997=CARTESIAN_POINT('Ctrl Pts',(130.021713385473,51.6217126940862,202.502527760224));
#89998=CARTESIAN_POINT('Ctrl Pts',(130.030551890778,51.6180547683919,202.540342857465));
#89999=CARTESIAN_POINT('Ctrl Pts',(130.038818443306,51.6146335524908,202.575710883717));
#90000=CARTESIAN_POINT('Ctrl Pts',(130.044431912552,51.6122898468198,202.611949523054));
#90001=CARTESIAN_POINT('Ctrl Pts',(130.047175263708,51.6111411941615,202.648495735808));
#90002=CARTESIAN_POINT('Ctrl Pts',(130.048460491453,51.6106030639031,202.665617206574));
#90003=CARTESIAN_POINT('Ctrl Pts',(130.049115378049,51.61032741828,202.682805650654));
#90004=CARTESIAN_POINT('Ctrl Pts',(130.049115378049,51.61032741828,202.7));
#90005=CARTESIAN_POINT('Ctrl Pts',(130.049115378049,50.178482477843,227.7));
#90006=CARTESIAN_POINT('Ctrl Pts',(130.049115378049,50.178482477843,227.));
#90007=CARTESIAN_POINT('Ctrl Pts',(130.749115378049,50.178482477843,227.));
#90008=CARTESIAN_POINT('Ctrl Pts',(130.049115378049,50.3640529785653,227.699999985699));
#90009=CARTESIAN_POINT('Ctrl Pts',(130.049115378046,50.2742101005222,227.019246371374));
#90010=CARTESIAN_POINT('Ctrl Pts',(130.729594026839,50.2755777892112,227.));
#90011=CARTESIAN_POINT('Ctrl Pts',(130.049115378049,50.5491164643398,227.664615075625));
#90012=CARTESIAN_POINT('Ctrl Pts',(130.049115378049,50.3786321825897,227.019287176017));
#90013=CARTESIAN_POINT('Ctrl Pts',(130.710551910362,50.3722574264186,226.982307540039));
#90014=CARTESIAN_POINT('Ctrl Pts',(130.049115378049,50.8080062597781,227.560942587807));
#90015=CARTESIAN_POINT('Ctrl Pts',(130.049115378049,50.5320966264688,226.984154463904));
#90016=CARTESIAN_POINT('Ctrl Pts',(130.6843993777,50.5073482333576,226.93047129279));
#90017=CARTESIAN_POINT('Ctrl Pts',(130.049115378049,50.8899726556653,227.518580284352));
#90018=CARTESIAN_POINT('Ctrl Pts',(130.049115378049,50.581618854421,226.967154819554));
#90019=CARTESIAN_POINT('Ctrl Pts',(130.676202303086,50.5500914608447,226.909290141361));
#90020=CARTESIAN_POINT('Ctrl Pts',(130.049115378049,51.04529430901,227.418334861381));
#90021=CARTESIAN_POINT('Ctrl Pts',(130.049115378049,50.676931026749,226.922196051976));
#90022=CARTESIAN_POINT('Ctrl Pts',(130.660793255904,50.6310467935792,226.859167431505));
#90023=CARTESIAN_POINT('Ctrl Pts',(130.049115378049,51.1192364398054,227.359716859222));
#90024=CARTESIAN_POINT('Ctrl Pts',(130.049115378048,50.7232221818321,226.893911925771));
#90025=CARTESIAN_POINT('Ctrl Pts',(130.653524972478,50.6695641554132,226.8298584301));
#90026=CARTESIAN_POINT('Ctrl Pts',(130.049115378049,51.3187163915109,227.166709167936));
#90027=CARTESIAN_POINT('Ctrl Pts',(130.049115378052,50.8489603384451,226.796066144146));
#90028=CARTESIAN_POINT('Ctrl Pts',(130.634047549317,50.7734331756717,226.733354582991));
#90029=CARTESIAN_POINT('Ctrl Pts',(130.049115378049,51.4266877775246,227.010514764464));
#90030=CARTESIAN_POINT('Ctrl Pts',(130.049115378049,50.9199140373353,226.710257286212));
#90031=CARTESIAN_POINT('Ctrl Pts',(130.62369129701,50.8295933572578,226.655257382363));
#90032=CARTESIAN_POINT('Ctrl Pts',(130.049115378049,51.5719050301311,226.671150503398));
#90033=CARTESIAN_POINT('Ctrl Pts',(130.049115378049,51.0153618694534,226.517377439877));
#90034=CARTESIAN_POINT('Ctrl Pts',(130.609830059099,50.9051050736271,226.485575251568));
#90035=CARTESIAN_POINT('Ctrl Pts',(130.049115378049,51.6103274150268,226.484470451835));
#90036=CARTESIAN_POINT('Ctrl Pts',(130.049115378049,51.0412521582374,226.407900947214));
#90037=CARTESIAN_POINT('Ctrl Pts',(130.606204738526,50.9250708611343,226.392235226019));
#90038=CARTESIAN_POINT('Ctrl Pts',(130.049115378049,51.61032741828,226.3));
#90039=CARTESIAN_POINT('Ctrl Pts',(130.049115378049,51.0412521604076,226.3));
#90040=CARTESIAN_POINT('Ctrl Pts',(130.606204737894,50.9250708612662,226.3));
#90041=CARTESIAN_POINT('',(130.049115378049,51.61032741828,226.3));
#90042=CARTESIAN_POINT('',(130.049115378049,50.178482477843,227.7));
#90043=CARTESIAN_POINT('Ctrl Pts',(130.049115378049,51.61032741828,226.3));
#90044=CARTESIAN_POINT('Ctrl Pts',(130.049115378049,51.6103274173581,226.352275490756));
#90045=CARTESIAN_POINT('Ctrl Pts',(130.049115378049,51.6072458611602,226.40444186111));
#90046=CARTESIAN_POINT('Ctrl Pts',(130.04911537805,51.6012540856931,226.456167219767));
#90047=CARTESIAN_POINT('Ctrl Pts',(130.04911537805,51.5950870508888,226.509405544342));
#90048=CARTESIAN_POINT('Ctrl Pts',(130.049115378051,51.5858369917708,226.562177812294));
#90049=CARTESIAN_POINT('Ctrl Pts',(130.049115378052,51.5736365792281,226.614138230052));
#90050=CARTESIAN_POINT('Ctrl Pts',(130.049115378054,51.5612855538423,226.666740093844));
#90051=CARTESIAN_POINT('Ctrl Pts',(130.049115378054,51.5459106783256,226.718511224708));
#90052=CARTESIAN_POINT('Ctrl Pts',(130.049115378053,51.5275972011629,226.769090547588));
#90053=CARTESIAN_POINT('Ctrl Pts',(130.049115378053,51.5188348162022,226.793291058184));
#90054=CARTESIAN_POINT('Ctrl Pts',(130.049115378052,51.5093989505799,226.817218572867));
#90055=CARTESIAN_POINT('Ctrl Pts',(130.049115378051,51.4992949803203,226.840832024798));
#90056=CARTESIAN_POINT('Ctrl Pts',(130.049115378051,51.4991039032287,226.841278580915));
#90057=CARTESIAN_POINT('Ctrl Pts',(130.049115378051,51.4989125789814,226.841725048981));
#90058=CARTESIAN_POINT('Ctrl Pts',(130.049115378051,51.498721007717,226.842171428811));
#90059=CARTESIAN_POINT('Ctrl Pts',(130.049115378049,51.4829426914355,226.878936452861));
#90060=CARTESIAN_POINT('Ctrl Pts',(130.049115378049,51.4654314885516,226.915223527298));
#90061=CARTESIAN_POINT('Ctrl Pts',(130.049115378049,51.4463326897367,226.950746995099));
#90062=CARTESIAN_POINT('Ctrl Pts',(130.049115378049,51.4270191511954,226.986669875442));
#90063=CARTESIAN_POINT('Ctrl Pts',(130.049115378049,51.4060825500491,227.021811110712));
#90064=CARTESIAN_POINT('Ctrl Pts',(130.049115378049,51.3837210648003,227.055897707461));
#90065=CARTESIAN_POINT('Ctrl Pts',(130.049115378049,51.3772329873993,227.065787769574));
#90066=CARTESIAN_POINT('Ctrl Pts',(130.049115378049,51.3706252381693,227.075589231533));
#90067=CARTESIAN_POINT('Ctrl Pts',(130.049115378049,51.3639033150166,227.085295915543));
#90068=CARTESIAN_POINT('Ctrl Pts',(130.049115378049,51.3417215427007,227.117327143775));
#90069=CARTESIAN_POINT('Ctrl Pts',(130.049115378049,51.3183237725072,227.14829466271));
#90070=CARTESIAN_POINT('Ctrl Pts',(130.049115378049,51.2937326377604,227.1782127794));
#90071=CARTESIAN_POINT('Ctrl Pts',(130.049115378049,51.2692357654807,227.208016214294));
#90072=CARTESIAN_POINT('Ctrl Pts',(130.04911537805,51.243554116965,227.236778933117));
#90073=CARTESIAN_POINT('Ctrl Pts',(130.04911537805,51.2166697232773,227.264483603619));
#90074=CARTESIAN_POINT('Ctrl Pts',(130.04911537805,51.2065284811418,227.274934267863));
#90075=CARTESIAN_POINT('Ctrl Pts',(130.04911537805,51.1962157273765,227.285234007762));
#90076=CARTESIAN_POINT('Ctrl Pts',(130.049115378049,51.1857292329141,227.295380420424));
#90077=CARTESIAN_POINT('Ctrl Pts',(130.049115378049,51.1854959240312,227.295606162994));
#90078=CARTESIAN_POINT('Ctrl Pts',(130.049115378049,51.1852625144088,227.295831843945));
#90079=CARTESIAN_POINT('Ctrl Pts',(130.049115378049,51.1850290041207,227.296057463206));
#90080=CARTESIAN_POINT('Ctrl Pts',(130.049115378049,51.1187206958901,227.360125010799));
#90081=CARTESIAN_POINT('Ctrl Pts',(130.049115378049,51.0450217810817,227.418510753969));
#90082=CARTESIAN_POINT('Ctrl Pts',(130.049115378049,50.9676333634749,227.468457388699));
#90083=CARTESIAN_POINT('Ctrl Pts',(130.049115378049,50.9674289789469,227.468589298869));
#90084=CARTESIAN_POINT('Ctrl Pts',(130.049115378049,50.9672245646234,227.468721155272));
#90085=CARTESIAN_POINT('Ctrl Pts',(130.049115378049,50.9670201205043,227.468852957906));
#90086=CARTESIAN_POINT('Ctrl Pts',(130.049115378049,50.8895409876893,227.51880281126));
#90087=CARTESIAN_POINT('Ctrl Pts',(130.049115378049,50.8077835053153,227.561031606915));
#90088=CARTESIAN_POINT('Ctrl Pts',(130.049115378049,50.721709619144,227.595499978478));
#90089=CARTESIAN_POINT('Ctrl Pts',(130.049115378049,50.7215582076484,227.595560611359));
#90090=CARTESIAN_POINT('Ctrl Pts',(130.049115378049,50.721406786528,227.595621218291));
#90091=CARTESIAN_POINT('Ctrl Pts',(130.049115378049,50.7212553557907,227.595681799273));
#90092=CARTESIAN_POINT('Ctrl Pts',(130.049115378049,50.6710671469183,227.615759962087));
#90093=CARTESIAN_POINT('Ctrl Pts',(130.049115378049,50.6199526275822,227.632940553192));
#90094=CARTESIAN_POINT('Ctrl Pts',(130.049115378049,50.5681013780827,227.647244653797));
#90095=CARTESIAN_POINT('Ctrl Pts',(130.049115378049,50.5160514903066,227.661603552347));
#90096=CARTESIAN_POINT('Ctrl Pts',(130.049115378049,50.4632583681232,227.673064024006));
#90097=CARTESIAN_POINT('Ctrl Pts',(130.049115378049,50.4098993109671,227.681596908351));
#90098=CARTESIAN_POINT('Ctrl Pts',(130.049115378049,50.3572232257564,227.690020575613));
#90099=CARTESIAN_POINT('Ctrl Pts',(130.049115378049,50.3039947720342,227.695591155994));
#90100=CARTESIAN_POINT('Ctrl Pts',(130.049115378049,50.2503829577808,227.698230353047));
#90101=CARTESIAN_POINT('Ctrl Pts',(130.049115378049,50.2264870648022,227.699406697686));
#90102=CARTESIAN_POINT('Ctrl Pts',(130.049115378049,50.2025150640935,227.699999998148));
#90103=CARTESIAN_POINT('Ctrl Pts',(130.049115378049,50.178482477843,227.7));
#90104=CARTESIAN_POINT('Origin',(130.749115378049,50.178482477843,227.7));
#90105=CARTESIAN_POINT('Origin',(130.749115378049,51.61032741828,226.3));
#90106=CARTESIAN_POINT('Origin',(125.29348064571,25.4505574462982,227.7));
#90107=CARTESIAN_POINT('',(130.749115378049,25.4505574462982,227.));
#90108=CARTESIAN_POINT('',(130.049115378049,25.4505574462982,227.7));
#90109=CARTESIAN_POINT('Origin',(130.749115378049,25.4505574462982,227.7));
#90110=CARTESIAN_POINT('Origin',(125.29348064571,25.4505574462982,227.7));
#90111=CARTESIAN_POINT('Origin',(125.29348064571,25.4505574462982,227.));
#90112=CARTESIAN_POINT('Origin',(129.349115378049,25.4505574462982,202.7));
#90113=CARTESIAN_POINT('',(130.049115378049,53.4601166829598,202.7));
#90114=CARTESIAN_POINT('',(129.349115378049,51.0349239481607,202.));
#90115=CARTESIAN_POINT('Origin',(130.749115378049,51.61032741828,227.));
#90116=CARTESIAN_POINT('',(130.049115378049,51.61032741828,202.));
#90117=CARTESIAN_POINT('Origin',(130.749115378049,25.4505574462982,227.7));
#90118=CARTESIAN_POINT('',(130.049115378049,51.0349239481607,227.7));
#90119=CARTESIAN_POINT('',(130.749115378049,25.4505574462982,227.));
#90120=CARTESIAN_POINT('Origin',(125.29348064571,25.4505574462982,229.));
#90121=CARTESIAN_POINT('Origin',(125.29348064571,25.4505574462982,202.));
#90122=CARTESIAN_POINT('Origin',(125.29348064571,53.4601166829598,202.));
#90123=CARTESIAN_POINT('',(120.537845913371,53.4601166829598,202.));
#90124=CARTESIAN_POINT('',(130.049115378049,53.4601166829598,202.));
#90125=CARTESIAN_POINT('Origin',(125.29348064571,25.4505574462982,202.));
#90126=CARTESIAN_POINT('',(130.049115378049,25.4505574462982,202.));
#90127=CARTESIAN_POINT('',(120.537845913371,25.4505574462982,202.));
#90128=CARTESIAN_POINT('Origin',(130.049115378049,25.4505574462982,202.));
#90129=CARTESIAN_POINT('Origin',(120.537845913371,25.4505574462982,202.));
#90130=CARTESIAN_POINT('Origin',(125.29348064571,25.4505574462982,227.));
#90131=CARTESIAN_POINT('Origin',(37.8448101558397,24.2184812945555,172.608250755187));
#90132=CARTESIAN_POINT('',(16.5267601345175,3.11418027746145,173.108250755187));
#90133=CARTESIAN_POINT('',(16.8785276479032,2.7588499853016,172.608250755187));
#90134=CARTESIAN_POINT('Origin',(16.5267601345175,3.11418027746145,172.608250755187));
#90135=CARTESIAN_POINT('',(38.1965776692254,23.8631510023956,172.608250755187));
#90136=CARTESIAN_POINT('',(37.8448101558397,24.2184812945555,173.108250755187));
#90137=CARTESIAN_POINT('Origin',(14.0868850299881,5.57876697388923,172.608250755187));
#90138=CARTESIAN_POINT('',(11.6470099254586,8.043353670317,173.108250755187));
#90139=CARTESIAN_POINT('',(11.2952424120729,8.39868396247686,172.608250755187));
#90140=CARTESIAN_POINT('Origin',(11.6470099254586,8.043353670317,172.608250755187));
#90141=CARTESIAN_POINT('Origin',(14.0868850299881,5.57876697388923,172.608250755187));
#90142=CARTESIAN_POINT('Origin',(14.0868850299881,5.57876697388923,173.108250755187));
#90143=CARTESIAN_POINT('Origin',(32.9650599467808,29.147654687411,172.608250755187));
#90144=CARTESIAN_POINT('',(32.6132924333951,29.5029849795709,172.608250755187));
#90145=CARTESIAN_POINT('',(32.9650599467808,29.147654687411,173.108250755187));
#90146=CARTESIAN_POINT('Origin',(35.4049350513103,26.6830679909832,152.608250755187));
#90147=CARTESIAN_POINT('',(21.5010931458411,17.798633272459,153.108250755187));
#90148=CARTESIAN_POINT('Origin',(21.5010931458411,17.798633272459,152.608250755187));
#90149=CARTESIAN_POINT('',(26.3808433549,12.8694598796034,153.108250755187));
#90150=CARTESIAN_POINT('Origin',(26.3808433549,12.8694598796034,152.608250755187));
#90151=CARTESIAN_POINT('Origin',(35.4049350513103,26.6830679909832,153.108250755187));
#90152=CARTESIAN_POINT('Ctrl Pts',(27.5073406548652,12.768040044578,153.608250755187));
#90153=CARTESIAN_POINT('Ctrl Pts',(27.1779404377158,12.9549939852504,153.608250755187));
#90154=CARTESIAN_POINT('Ctrl Pts',(26.9087733165906,12.6885257134127,153.608250755187));
#90155=CARTESIAN_POINT('Ctrl Pts',(27.5073406342015,12.7680400563058,153.475551801171));
#90156=CARTESIAN_POINT('Ctrl Pts',(27.1779404229081,12.9549939942968,153.527723751245));
#90157=CARTESIAN_POINT('Ctrl Pts',(26.9087733118706,12.68852570874,153.541901279333));
#90158=CARTESIAN_POINT('Ctrl Pts',(27.4836651381883,12.7814084763901,153.342399703391));
#90159=CARTESIAN_POINT('Ctrl Pts',(27.1606400720877,12.965534956355,153.446619353193));
#90160=CARTESIAN_POINT('Ctrl Pts',(26.893846651724,12.6927270912806,153.475325227732));
#90161=CARTESIAN_POINT('Ctrl Pts',(27.3943038776747,12.8327090607538,153.098820706789));
#90162=CARTESIAN_POINT('Ctrl Pts',(27.0980595223776,13.0041108087012,153.3049590945));
#90163=CARTESIAN_POINT('Ctrl Pts',(26.8377244017675,12.7092343374354,153.353535732545));
#90164=CARTESIAN_POINT('Ctrl Pts',(27.3285209197659,12.8707492134963,152.987832794725));
#90165=CARTESIAN_POINT('Ctrl Pts',(27.0522238475563,13.0325418769711,153.243730625338));
#90166=CARTESIAN_POINT('Ctrl Pts',(26.7964812241876,12.7215983775456,153.298041773782));
#90167=CARTESIAN_POINT('Ctrl Pts',(27.168815411942,12.9653805575585,152.805062971569));
#90168=CARTESIAN_POINT('Ctrl Pts',(26.9473919563668,13.0985506777719,153.152596157915));
#90169=CARTESIAN_POINT('Ctrl Pts',(26.696939992414,12.7533719782571,153.206656864552));
#90170=CARTESIAN_POINT('Ctrl Pts',(27.0735561471923,13.0228217613016,152.731827736181));
#90171=CARTESIAN_POINT('Ctrl Pts',(26.8870893049663,13.136998440275,153.1222986856));
#90172=CARTESIAN_POINT('Ctrl Pts',(26.637823732227,12.7730921439478,153.170039246316));
#90173=CARTESIAN_POINT('Ctrl Pts',(26.8710052246367,13.1484367358317,152.633922888492));
#90174=CARTESIAN_POINT('Ctrl Pts',(26.7679788506669,13.2138353374613,153.093277185672));
#90175=CARTESIAN_POINT('Ctrl Pts',(26.5130205024505,12.8177036267266,153.121086821207));
#90176=CARTESIAN_POINT('Ctrl Pts',(26.760985873486,13.2183592414295,152.608250765972));
#90177=CARTESIAN_POINT('Ctrl Pts',(26.7075856545808,13.2532442939392,153.094953472493));
#90178=CARTESIAN_POINT('Ctrl Pts',(26.4456558529318,12.8432444717969,153.108250755187));
#90179=CARTESIAN_POINT('Ctrl Pts',(26.6543006790336,13.2880540647968,152.608250755187));
#90180=CARTESIAN_POINT('Ctrl Pts',(26.6543006790336,13.2880540647968,153.108250755187));
#90181=CARTESIAN_POINT('Ctrl Pts',(26.3808433549,12.8694598796034,153.108250755187));
#90182=CARTESIAN_POINT('',(26.9087733165906,12.6885257134127,153.608250755187));
#90183=CARTESIAN_POINT('Origin',(27.2605408299763,12.3331954212528,153.608250755187));
#90184=CARTESIAN_POINT('Ctrl Pts',(26.9087733165906,12.6885257134127,153.608250755187));
#90185=CARTESIAN_POINT('Ctrl Pts',(26.9087733165906,12.6885257134127,153.58561192993));
#90186=CARTESIAN_POINT('Ctrl Pts',(26.9070395695061,12.6890138059481,153.563154237045));
#90187=CARTESIAN_POINT('Ctrl Pts',(26.9037135366198,12.6899636529495,153.541035429084));
#90188=CARTESIAN_POINT('Ctrl Pts',(26.900229546794,12.6909586092238,153.517866174742));
#90189=CARTESIAN_POINT('Ctrl Pts',(26.8949984104558,12.6924601686093,153.495067766235));
#90190=CARTESIAN_POINT('Ctrl Pts',(26.8881298385863,12.6944521653016,153.472807844592));
#90191=CARTESIAN_POINT('Ctrl Pts',(26.886517484165,12.6949197741052,153.467582466775));
#90192=CARTESIAN_POINT('Ctrl Pts',(26.8848146808982,12.6954144688681,153.462386743418));
#90193=CARTESIAN_POINT('Ctrl Pts',(26.8830224554071,12.6959361508752,153.457222835554));
#90194=CARTESIAN_POINT('Ctrl Pts',(26.8779742821994,12.6974055759806,153.442677622656));
#90195=CARTESIAN_POINT('Ctrl Pts',(26.8722166021153,12.699089141154,153.428386396435));
#90196=CARTESIAN_POINT('Ctrl Pts',(26.8657855267457,12.700980714358,153.414430480138));
#90197=CARTESIAN_POINT('Ctrl Pts',(26.8632008765685,12.7017409379188,153.408821595238));
#90198=CARTESIAN_POINT('Ctrl Pts',(26.860507107671,12.7025352357299,153.40326444683));
#90199=CARTESIAN_POINT('Ctrl Pts',(26.8577089907892,12.7033627973938,153.397762970209));
#90200=CARTESIAN_POINT('Ctrl Pts',(26.8434713128181,12.7075736852767,153.369769767704));
#90201=CARTESIAN_POINT('Ctrl Pts',(26.826539106381,12.7126442230621,153.343230009335));
#90202=CARTESIAN_POINT('Ctrl Pts',(26.8074888665516,12.7184791208889,153.318537883336));
#90203=CARTESIAN_POINT('Ctrl Pts',(26.7890492187098,12.7241270005001,153.294637181194));
#90204=CARTESIAN_POINT('Ctrl Pts',(26.7686251816549,12.7304910090134,153.272467520466));
#90205=CARTESIAN_POINT('Ctrl Pts',(26.7467118251245,12.7374867495037,153.252349061816));
#90206=CARTESIAN_POINT('Ctrl Pts',(26.7447051617612,12.738127367755,153.250506761946));
#90207=CARTESIAN_POINT('Ctrl Pts',(26.7426846595016,12.7387737898784,153.248680454799));
#90208=CARTESIAN_POINT('Ctrl Pts',(26.7406507833593,12.7394259068857,153.246870287867));
#90209=CARTESIAN_POINT('Ctrl Pts',(26.7219609664006,12.7454183797056,153.230236193034));
#90210=CARTESIAN_POINT('Ctrl Pts',(26.7021655132865,12.751883330314,153.214981265978));
#90211=CARTESIAN_POINT('Ctrl Pts',(26.6815451859053,12.7587610622873,153.201166192582));
#90212=CARTESIAN_POINT('Ctrl Pts',(26.6596871824718,12.7660516104105,153.186521909001));
#90213=CARTESIAN_POINT('Ctrl Pts',(26.6369012258168,12.7738061414819,153.173494523172));
#90214=CARTESIAN_POINT('Ctrl Pts',(26.6134755587766,12.7819706583732,153.162187747804));
#90215=CARTESIAN_POINT('Ctrl Pts',(26.6009612965353,12.7863322377159,153.156147537644));
#90216=CARTESIAN_POINT('Ctrl Pts',(26.5882638090727,12.7908110879768,153.150598972776));
#90217=CARTESIAN_POINT('Ctrl Pts',(26.5754238802881,12.7954005301352,153.145562771898));
#90218=CARTESIAN_POINT('Ctrl Pts',(26.5512362102307,12.8040460541516,153.13607565034));
#90219=CARTESIAN_POINT('Ctrl Pts',(26.5262911060842,12.8131811825813,153.128328353012));
#90220=CARTESIAN_POINT('Ctrl Pts',(26.500936708412,12.822692741828,153.12238823827));
#90221=CARTESIAN_POINT('Ctrl Pts',(26.477347025937,12.8315422781244,153.116861567023));
#90222=CARTESIAN_POINT('Ctrl Pts',(26.453401570454,12.8407182262646,153.112899483272));
#90223=CARTESIAN_POINT('Ctrl Pts',(26.4293898763036,12.8501313371653,153.110597998101));
#90224=CARTESIAN_POINT('Ctrl Pts',(26.4132055677847,12.8564759411731,153.1090467562));
#90225=CARTESIAN_POINT('Ctrl Pts',(26.3969913673361,12.8629283194239,153.108250755187));
#90226=CARTESIAN_POINT('Ctrl Pts',(26.3808433549,12.8694598796034,153.108250755187));
#90227=CARTESIAN_POINT('Ctrl Pts',(21.9224216884311,18.0678585669597,152.608250755187));
#90228=CARTESIAN_POINT('Ctrl Pts',(21.9224216884311,18.0678585669597,153.108250755187));
#90229=CARTESIAN_POINT('Ctrl Pts',(21.5010931458411,17.798633272459,153.108250755187));
#90230=CARTESIAN_POINT('Ctrl Pts',(21.8529692250382,18.1765493392546,152.60825077749));
#90231=CARTESIAN_POINT('Ctrl Pts',(21.8877231275685,18.1221606460453,153.094787604517));
#90232=CARTESIAN_POINT('Ctrl Pts',(21.4752187820791,17.8645045048257,153.108250755187));
#90233=CARTESIAN_POINT('Ctrl Pts',(21.7851621994479,18.2856761107434,152.633710236017));
#90234=CARTESIAN_POINT('Ctrl Pts',(21.8494711012016,18.1820886305035,153.093185957657));
#90235=CARTESIAN_POINT('Ctrl Pts',(21.4507281499402,17.9311502346664,153.120980492262));
#90236=CARTESIAN_POINT('Ctrl Pts',(21.6607280584935,18.4909268139007,152.732462696752));
#90237=CARTESIAN_POINT('Ctrl Pts',(21.7732901420723,18.3028399523544,153.122507989483));
#90238=CARTESIAN_POINT('Ctrl Pts',(21.4070763536337,18.0572865403012,153.170356729309));
#90239=CARTESIAN_POINT('Ctrl Pts',(21.6047379954083,18.5859573989266,152.805334639289));
#90240=CARTESIAN_POINT('Ctrl Pts',(21.7357414624187,18.3630692431353,153.152707467856));
#90241=CARTESIAN_POINT('Ctrl Pts',(21.388124909213,18.1161056718009,153.206792695945));
#90242=CARTESIAN_POINT('Ctrl Pts',(21.5115995501989,18.7468303826906,152.988630571688));
#90243=CARTESIAN_POINT('Ctrl Pts',(21.6706947362434,18.4687247489851,153.244147548454));
#90244=CARTESIAN_POINT('Ctrl Pts',(21.3573191318963,18.2161018881959,153.29844066473));
#90245=CARTESIAN_POINT('Ctrl Pts',(21.4742934531536,18.8128807906121,153.099898214101));
#90246=CARTESIAN_POINT('Ctrl Pts',(21.6427661294028,18.5147847472079,153.30558183398));
#90247=CARTESIAN_POINT('Ctrl Pts',(21.345396035639,18.2573986678047,153.354074484501));
#90248=CARTESIAN_POINT('Ctrl Pts',(21.4242056493653,18.9022051021532,153.342371533405));
#90249=CARTESIAN_POINT('Ctrl Pts',(21.6050533759232,18.5773697525719,153.446616730793));
#90250=CARTESIAN_POINT('Ctrl Pts',(21.3295538767565,18.3133407705917,153.475311144439));
#90251=CARTESIAN_POINT('Ctrl Pts',(21.4110300989696,18.9260953737276,153.475893601961));
#90252=CARTESIAN_POINT('Ctrl Pts',(21.5946552032658,18.5948279601094,153.527930080756));
#90253=CARTESIAN_POINT('Ctrl Pts',(21.3254880800282,18.3283596898632,153.542072178464));
#90254=CARTESIAN_POINT('Ctrl Pts',(21.4110300971907,18.9260953769367,153.608250755187));
#90255=CARTESIAN_POINT('Ctrl Pts',(21.5946552018854,18.5948279624256,153.608250755187));
#90256=CARTESIAN_POINT('Ctrl Pts',(21.3254880807602,18.3283596905879,153.608250755187));
#90257=CARTESIAN_POINT('',(21.3254880807602,18.3283596905879,153.608250755187));
#90258=CARTESIAN_POINT('Origin',(20.9737205673745,18.6836899827478,153.608250755187));
#90259=CARTESIAN_POINT('Ctrl Pts',(21.5010931458411,17.798633272459,153.108250755187));
#90260=CARTESIAN_POINT('Ctrl Pts',(21.4905730502976,17.8254154443586,153.108250755187));
#90261=CARTESIAN_POINT('Ctrl Pts',(21.4803463693722,17.8521593410534,153.110350857061));
#90262=CARTESIAN_POINT('Ctrl Pts',(21.4704609701153,17.8786538141028,153.114447252937));
#90263=CARTESIAN_POINT('Ctrl Pts',(21.4603139997298,17.9058493401941,153.118652040884));
#90264=CARTESIAN_POINT('Ctrl Pts',(21.4505262446712,17.9327832401005,153.124960207408));
#90265=CARTESIAN_POINT('Ctrl Pts',(21.4411536697561,17.9592354635942,153.13331284971));
#90266=CARTESIAN_POINT('Ctrl Pts',(21.43698585605,17.9709982865785,153.137027117921));
#90267=CARTESIAN_POINT('Ctrl Pts',(21.4329002292475,17.9826658616096,153.141146354449));
#90268=CARTESIAN_POINT('Ctrl Pts',(21.4289022644077,17.9942183957151,153.145668609543));
#90269=CARTESIAN_POINT('Ctrl Pts',(21.4200063910211,18.0199239446167,153.155731081412));
#90270=CARTESIAN_POINT('Ctrl Pts',(21.4115784694086,18.0449504539261,153.167751327949));
#90271=CARTESIAN_POINT('Ctrl Pts',(21.4036467411062,18.0690479409556,153.181631702462));
#90272=CARTESIAN_POINT('Ctrl Pts',(21.3960731025622,18.0920575108276,153.19488542667));
#90273=CARTESIAN_POINT('Ctrl Pts',(21.3889517927388,18.1142208889259,153.209835861403));
#90274=CARTESIAN_POINT('Ctrl Pts',(21.3823199823874,18.1352871692309,153.226428438647));
#90275=CARTESIAN_POINT('Ctrl Pts',(21.3797305551073,18.143512615681,153.232907102826));
#90276=CARTESIAN_POINT('Ctrl Pts',(21.3772159005764,18.1515703676921,153.239636401772));
#90277=CARTESIAN_POINT('Ctrl Pts',(21.3747788264842,18.1594436001056,153.246614074428));
#90278=CARTESIAN_POINT('Ctrl Pts',(21.374086775673,18.1616793453772,153.248595509476));
#90279=CARTESIAN_POINT('Ctrl Pts',(21.3734011788201,18.1638995706237,153.250596415344));
#90280=CARTESIAN_POINT('Ctrl Pts',(21.3727221102163,18.1661038480104,153.252616665764));
#90281=CARTESIAN_POINT('Ctrl Pts',(21.3657201020249,18.1888325800269,153.273447860005));
#90282=CARTESIAN_POINT('Ctrl Pts',(21.3593972300783,18.2098942489177,153.296424536252));
#90283=CARTESIAN_POINT('Ctrl Pts',(21.3538250978631,18.2287912078363,153.321170461488));
#90284=CARTESIAN_POINT('Ctrl Pts',(21.3485511315198,18.2466769868303,153.344592227481));
#90285=CARTESIAN_POINT('Ctrl Pts',(21.3439497209919,18.2626236397157,153.369599261715));
#90286=CARTESIAN_POINT('Ctrl Pts',(21.3400895512389,18.2761669413073,153.395852653192));
#90287=CARTESIAN_POINT('Ctrl Pts',(21.3391761782763,18.2793714857415,153.402064591911));
#90288=CARTESIAN_POINT('Ctrl Pts',(21.3383043412798,18.2824412753061,153.408346207007));
#90289=CARTESIAN_POINT('Ctrl Pts',(21.3374750195038,18.2853697768887,153.414692806039));
#90290=CARTESIAN_POINT('Ctrl Pts',(21.3340535782225,18.297451572515,153.4408762689));
#90291=CARTESIAN_POINT('Ctrl Pts',(21.3313279236915,18.3072005590295,153.468385102508));
#90292=CARTESIAN_POINT('Ctrl Pts',(21.3293445811899,18.3143466012112,153.49672275683));
#90293=CARTESIAN_POINT('Ctrl Pts',(21.3274524666984,18.3211639461519,153.523756961136));
#90294=CARTESIAN_POINT('Ctrl Pts',(21.3262359632126,18.3256122792073,153.551545730234));
#90295=CARTESIAN_POINT('Ctrl Pts',(21.3257408437783,18.3274298612427,153.579619100729));
#90296=CARTESIAN_POINT('Ctrl Pts',(21.3255729780825,18.3280460957344,153.589137119097));
#90297=CARTESIAN_POINT('Ctrl Pts',(21.3254880807602,18.3283596905879,153.598687494769));
#90298=CARTESIAN_POINT('Ctrl Pts',(21.3254880807602,18.3283596905879,153.608250755187));
#90299=CARTESIAN_POINT('Origin',(27.2605408299763,12.3331954212528,171.608250755187));
#90300=CARTESIAN_POINT('',(26.9087733165906,12.6885257134127,171.108250755187));
#90301=CARTESIAN_POINT('Origin',(27.2605408299763,12.3331954212528,171.108250755187));
#90302=CARTESIAN_POINT('',(26.9087733165906,12.6885257134127,153.108250755187));
#90303=CARTESIAN_POINT('Origin',(37.8448101558397,24.2184812945555,153.608250755187));
#90304=CARTESIAN_POINT('',(16.8785276479032,2.7588499853016,153.608250755187));
#90305=CARTESIAN_POINT('',(16.5267601345175,3.11418027746145,153.108250755187));
#90306=CARTESIAN_POINT('Origin',(16.5267601345175,3.11418027746145,153.608250755187));
#90307=CARTESIAN_POINT('',(16.5267601345175,3.11418027746145,153.108250755187));
#90308=CARTESIAN_POINT('',(27.1812285825866,12.9582491609851,153.608250755187));
#90309=CARTESIAN_POINT('Origin',(32.9650599467808,29.147654687411,153.608250755187));
#90310=CARTESIAN_POINT('',(11.6470099254586,8.043353670317,153.108250755187));
#90311=CARTESIAN_POINT('',(11.2952424120729,8.39868396247686,153.608250755187));
#90312=CARTESIAN_POINT('Origin',(11.6470099254586,8.04335367031701,153.608250755187));
#90313=CARTESIAN_POINT('',(11.2952424120729,8.39868396247685,153.608250755187));
#90314=CARTESIAN_POINT('',(21.949710860142,18.2427528460005,153.108250755187));
#90315=CARTESIAN_POINT('Origin',(20.9737205673745,18.6836899827478,171.608250755187));
#90316=CARTESIAN_POINT('',(21.3254880807602,18.3283596905879,171.108250755187));
#90317=CARTESIAN_POINT('Origin',(20.9737205673745,18.6836899827478,171.108250755187));
#90318=CARTESIAN_POINT('',(21.3254880807602,18.3283596905879,153.108250755187));
#90319=CARTESIAN_POINT('Ctrl Pts',(26.9087733165906,12.6885257134127,171.108250755187));
#90320=CARTESIAN_POINT('Ctrl Pts',(27.1779404377158,12.9549939852504,171.108250755187));
#90321=CARTESIAN_POINT('Ctrl Pts',(27.5073406548652,12.768040044578,171.108250755187));
#90322=CARTESIAN_POINT('Ctrl Pts',(26.9087733340747,12.6885257307215,171.241737242521));
#90323=CARTESIAN_POINT('Ctrl Pts',(27.177940450083,12.9549939974924,171.189238482122));
#90324=CARTESIAN_POINT('Ctrl Pts',(27.5073406604818,12.7680400413903,171.174993997722));
#90325=CARTESIAN_POINT('Ctrl Pts',(26.9289558292315,12.7085058627054,171.375809742194));
#90326=CARTESIAN_POINT('Ctrl Pts',(27.1924226045785,12.9693309442371,171.270872142595));
#90327=CARTESIAN_POINT('Ctrl Pts',(27.5205585322336,12.7762529890485,171.242030250225));
#90328=CARTESIAN_POINT('Ctrl Pts',(27.0054626143324,12.784245539693,171.620480252948));
#90329=CARTESIAN_POINT('Ctrl Pts',(27.2458363457333,13.0222091235587,171.414405744627));
#90330=CARTESIAN_POINT('Ctrl Pts',(27.5708445650066,12.8073151622189,171.364365502532));
#90331=CARTESIAN_POINT('Ctrl Pts',(27.0619560851888,12.8401725692881,171.731805299994));
#90332=CARTESIAN_POINT('Ctrl Pts',(27.2853253179226,13.0613021529443,171.477100056791));
#90333=CARTESIAN_POINT('Ctrl Pts',(27.608034085531,12.8302288792103,171.420028028856));
#90334=CARTESIAN_POINT('Ctrl Pts',(27.1998136024674,12.9766478350469,171.914243767979));
#90335=CARTESIAN_POINT('Ctrl Pts',(27.3778758818511,13.1529247431196,171.570720798637));
#90336=CARTESIAN_POINT('Ctrl Pts',(27.6992900235444,12.8859483002505,171.511247260317));
#90337=CARTESIAN_POINT('Ctrl Pts',(27.2823137807828,13.0583208114866,171.986819299416));
#90338=CARTESIAN_POINT('Ctrl Pts',(27.4322874234685,13.2067907182887,171.602133212335));
#90339=CARTESIAN_POINT('Ctrl Pts',(27.7541210219345,12.9192082849093,171.547535027057));
#90340=CARTESIAN_POINT('Ctrl Pts',(27.458765263205,13.2330030735239,172.083342412463));
#90341=CARTESIAN_POINT('Ctrl Pts',(27.541996530637,13.3153998086924,171.630196458045));
#90342=CARTESIAN_POINT('Ctrl Pts',(27.8721997120763,12.9900408536816,171.595796584069));
#90343=CARTESIAN_POINT('Ctrl Pts',(27.5549119618052,13.3281857411239,172.108250746497));
#90344=CARTESIAN_POINT('Ctrl Pts',(27.5989314668852,13.3717638772494,171.626173327528));
#90345=CARTESIAN_POINT('Ctrl Pts',(27.9369238543391,13.0284859943162,171.608250755187));
#90346=CARTESIAN_POINT('Ctrl Pts',(27.6489098612225,13.4212411548363,172.108250755187));
#90347=CARTESIAN_POINT('Ctrl Pts',(27.6489098612225,13.4212411548363,171.608250755187));
#90348=CARTESIAN_POINT('Ctrl Pts',(28.0006773746082,13.0659108626764,171.608250755187));
#90349=CARTESIAN_POINT('',(27.6489098612224,13.4212411548363,172.108250755187));
#90350=CARTESIAN_POINT('Origin',(28.0006773746082,13.0659108626764,172.108250755187));
#90351=CARTESIAN_POINT('Ctrl Pts',(27.6489098612224,13.4212411548363,172.108250755187));
#90352=CARTESIAN_POINT('Ctrl Pts',(27.6221197748791,13.3947196837871,172.10825075271));
#90353=CARTESIAN_POINT('Ctrl Pts',(27.595366665669,13.368234819114,172.106231383603));
#90354=CARTESIAN_POINT('Ctrl Pts',(27.5688036575348,13.3419381494357,172.102298699115));
#90355=CARTESIAN_POINT('Ctrl Pts',(27.5414606876917,13.3148693384654,172.098250540381));
#90356=CARTESIAN_POINT('Ctrl Pts',(27.5143182183118,13.2879990176061,172.092175073618));
#90357=CARTESIAN_POINT('Ctrl Pts',(27.4875298095769,13.2614792073432,172.084134831723));
#90358=CARTESIAN_POINT('Ctrl Pts',(27.4607131615435,13.234931440928,172.076086114118));
#90359=CARTESIAN_POINT('Ctrl Pts',(27.4342503195365,13.2087339330439,172.066068297256));
#90360=CARTESIAN_POINT('Ctrl Pts',(27.4082967712959,13.1830406124086,172.054093236391));
#90361=CARTESIAN_POINT('Ctrl Pts',(27.3955823048237,13.1704536296674,172.048226735654));
#90362=CARTESIAN_POINT('Ctrl Pts',(27.3829901821132,13.1579877639881,172.041889749808));
#90363=CARTESIAN_POINT('Ctrl Pts',(27.3705399239133,13.1456623403913,172.035079401128));
#90364=CARTESIAN_POINT('Ctrl Pts',(27.3703156689721,13.1454403339799,172.034956732641));
#90365=CARTESIAN_POINT('Ctrl Pts',(27.3700914459051,13.1452183591231,172.034833904296));
#90366=CARTESIAN_POINT('Ctrl Pts',(27.3698672547917,13.1449964158994,172.034710916136));
#90367=CARTESIAN_POINT('Ctrl Pts',(27.2819022951275,13.0579134516647,171.98645454965));
#90368=CARTESIAN_POINT('Ctrl Pts',(27.1996383705023,12.9764743600704,171.914009179875));
#90369=CARTESIAN_POINT('Ctrl Pts',(27.1308853210348,12.908410674588,171.823023819991));
#90370=CARTESIAN_POINT('Ctrl Pts',(27.1307685101586,12.9082950349356,171.822869236599));
#90371=CARTESIAN_POINT('Ctrl Pts',(27.1306517350126,12.9081794306553,171.822714595501));
#90372=CARTESIAN_POINT('Ctrl Pts',(27.1305349956251,12.9080638617748,171.822559896743));
#90373=CARTESIAN_POINT('Ctrl Pts',(27.0617656524892,12.8399840459953,171.731429283186));
#90374=CARTESIAN_POINT('Ctrl Pts',(27.0053994467863,12.7841830055056,171.620275542505));
#90375=CARTESIAN_POINT('Ctrl Pts',(26.9672095752599,12.7463760511325,171.498144778716));
#90376=CARTESIAN_POINT('Ctrl Pts',(26.9671771612793,12.7463439621561,171.498041119185));
#90377=CARTESIAN_POINT('Ctrl Pts',(26.9671447602716,12.7463118860226,171.497937451223));
#90378=CARTESIAN_POINT('Ctrl Pts',(26.9671123722381,12.7462798227331,171.497833774838));
#90379=CARTESIAN_POINT('Ctrl Pts',(26.9560651316504,12.7353433491563,171.462470776877));
#90380=CARTESIAN_POINT('Ctrl Pts',(26.9465607587732,12.725934273468,171.426245512338));
#90381=CARTESIAN_POINT('Ctrl Pts',(26.9386061022959,12.7180593756882,171.389360653073));
#90382=CARTESIAN_POINT('Ctrl Pts',(26.9306441693041,12.7101772743531,171.352442053416));
#90383=CARTESIAN_POINT('Ctrl Pts',(26.9242345978251,12.7038319695175,171.314861536714));
#90384=CARTESIAN_POINT('Ctrl Pts',(26.9194191830746,12.6990648373308,171.276805373256));
#90385=CARTESIAN_POINT('Ctrl Pts',(26.9147383382688,12.6944309258006,171.239812714414));
#90386=CARTESIAN_POINT('Ctrl Pts',(26.9115637593677,12.6912881773473,171.202369605235));
#90387=CARTESIAN_POINT('Ctrl Pts',(26.9099682233711,12.6897086392599,171.164646810882));
#90388=CARTESIAN_POINT('Ctrl Pts',(26.9091757117165,12.6889240738564,171.145909687915));
#90389=CARTESIAN_POINT('Ctrl Pts',(26.9087733190599,12.6885257158573,171.127103649704));
#90390=CARTESIAN_POINT('Ctrl Pts',(26.9087733165906,12.6885257134127,171.108250755187));
#90391=CARTESIAN_POINT('Origin',(14.0868850299881,5.57876697388923,153.608250755187));
#90392=CARTESIAN_POINT('Origin',(14.0868850299881,5.57876697388923,153.608250755187));
#90393=CARTESIAN_POINT('Origin',(14.0868850299881,5.57876697388923,153.108250755187));
#90394=CARTESIAN_POINT('Ctrl Pts',(22.0656246253921,19.0610751320115,172.108250755187));
#90395=CARTESIAN_POINT('Ctrl Pts',(22.0656246253921,19.0610751320115,171.608250755187));
#90396=CARTESIAN_POINT('Ctrl Pts',(21.7138571120063,19.4164054241714,171.608250755187));
#90397=CARTESIAN_POINT('Ctrl Pts',(21.970440150776,18.9668450404955,172.108250736963));
#90398=CARTESIAN_POINT('Ctrl Pts',(22.0150140548495,19.0109720168265,171.626400023775));
#90399=CARTESIAN_POINT('Ctrl Pts',(21.6753131026798,19.352235470221,171.608250755187));
#90400=CARTESIAN_POINT('Ctrl Pts',(21.8758188843882,18.873172510106,172.083590099036));
#90401=CARTESIAN_POINT('Ctrl Pts',(21.9589405696991,18.9554607618996,171.630295894894));
#90402=CARTESIAN_POINT('Ctrl Pts',(21.6368349074759,19.2889233489516,171.595920429989));
#90403=CARTESIAN_POINT('Ctrl Pts',(21.6980773333364,18.6972131145286,171.986236425372));
#90404=CARTESIAN_POINT('Ctrl Pts',(21.8484160221931,18.8460444073025,171.601943545762));
#90405=CARTESIAN_POINT('Ctrl Pts',(21.5642889040396,19.1707080971489,171.547243587402));
#90406=CARTESIAN_POINT('Ctrl Pts',(21.6164317208276,18.616386135448,171.914220536541));
#90407=CARTESIAN_POINT('Ctrl Pts',(21.7945323741985,18.7927010327448,171.570727890217));
#90408=CARTESIAN_POINT('Ctrl Pts',(21.530827148552,19.1167826550556,171.511235647295));
#90409=CARTESIAN_POINT('Ctrl Pts',(21.4781632900135,18.4795040762473,171.73102847759));
#90410=CARTESIAN_POINT('Ctrl Pts',(21.7016983911598,18.7007978652084,171.476689446385));
#90411=CARTESIAN_POINT('Ctrl Pts',(21.474021706278,19.0258237386761,171.419639614958));
#90412=CARTESIAN_POINT('Ctrl Pts',(21.4218647858374,18.4237700584664,171.619640310305));
#90413=CARTESIAN_POINT('Ctrl Pts',(21.6623323229597,18.6618265074946,171.413915961975));
#90414=CARTESIAN_POINT('Ctrl Pts',(21.450814218412,18.9889959729158,171.363945533082));
#90415=CARTESIAN_POINT('Ctrl Pts',(21.345712062812,18.3483808934915,171.37578205691));
#90416=CARTESIAN_POINT('Ctrl Pts',(21.6091642396647,18.6091915229033,171.270846895345));
#90417=CARTESIAN_POINT('Ctrl Pts',(21.4193928793478,18.9392570552062,171.242016405712));
#90418=CARTESIAN_POINT('Ctrl Pts',(21.3254880824681,18.3283596922787,171.241710900386));
#90419=CARTESIAN_POINT('Ctrl Pts',(21.5946552031017,18.5948279636278,171.189221495563));
#90420=CARTESIAN_POINT('Ctrl Pts',(21.4110300968858,18.9260953774867,171.17498082804));
#90421=CARTESIAN_POINT('Ctrl Pts',(21.3254880807602,18.3283596905879,171.108250755187));
#90422=CARTESIAN_POINT('Ctrl Pts',(21.5946552018854,18.5948279624256,171.108250755187));
#90423=CARTESIAN_POINT('Ctrl Pts',(21.4110300971907,18.9260953769367,171.108250755187));
#90424=CARTESIAN_POINT('',(22.0656246253921,19.0610751320115,172.108250755187));
#90425=CARTESIAN_POINT('Origin',(21.7138571120063,19.4164054241714,172.108250755187));
#90426=CARTESIAN_POINT('Ctrl Pts',(21.3254880807602,18.3283596905879,171.108250755187));
#90427=CARTESIAN_POINT('Ctrl Pts',(21.3254880812526,18.3283596910754,171.146726782705));
#90428=CARTESIAN_POINT('Ctrl Pts',(21.3271964240235,18.3300508975486,171.185041427676));
#90429=CARTESIAN_POINT('Ctrl Pts',(21.3305183422912,18.333339538009,171.22298649035));
#90430=CARTESIAN_POINT('Ctrl Pts',(21.3321922826555,18.3349967094283,171.242107301556));
#90431=CARTESIAN_POINT('Ctrl Pts',(21.334276539325,18.3370600938913,171.261134517834));
#90432=CARTESIAN_POINT('Ctrl Pts',(21.3367624462568,18.3395211258692,171.280042307355));
#90433=CARTESIAN_POINT('Ctrl Pts',(21.3418914454626,18.3445988023093,171.319053436934));
#90434=CARTESIAN_POINT('Ctrl Pts',(21.3487258208062,18.3513648861209,171.357556066236));
#90435=CARTESIAN_POINT('Ctrl Pts',(21.357163993125,18.3597187357998,171.395315415654));
#90436=CARTESIAN_POINT('Ctrl Pts',(21.3599099796439,18.3624372816807,171.407603226396));
#90437=CARTESIAN_POINT('Ctrl Pts',(21.3628260701827,18.365324228437,171.419812520361));
#90438=CARTESIAN_POINT('Ctrl Pts',(21.3659095386159,18.3683768672509,171.431935680483));
#90439=CARTESIAN_POINT('Ctrl Pts',(21.3706190483618,18.3730392896352,171.450451887793));
#90440=CARTESIAN_POINT('Ctrl Pts',(21.3757178706185,18.3780870998679,171.46876644342));
#90441=CARTESIAN_POINT('Ctrl Pts',(21.3811942208671,18.3835085796861,171.486850966306));
#90442=CARTESIAN_POINT('Ctrl Pts',(21.3822539081404,18.3845576493959,171.490350366066));
#90443=CARTESIAN_POINT('Ctrl Pts',(21.3833277549178,18.3856207337022,171.493841420748));
#90444=CARTESIAN_POINT('Ctrl Pts',(21.3844155368878,18.3866976107387,171.497323013247));
#90445=CARTESIAN_POINT('Ctrl Pts',(21.3857871789431,18.3880555021843,171.501713138128));
#90446=CARTESIAN_POINT('Ctrl Pts',(21.387181459874,18.3894358011567,171.506090294806));
#90447=CARTESIAN_POINT('Ctrl Pts',(21.3885977255394,18.3908378605866,171.510452436845));
#90448=CARTESIAN_POINT('Ctrl Pts',(21.4016701057897,18.4037791147949,171.550715772199));
#90449=CARTESIAN_POINT('Ctrl Pts',(21.4166313641888,18.4185899911857,171.58974450264));
#90450=CARTESIAN_POINT('Ctrl Pts',(21.4333457746744,18.4351365211234,171.627226319309));
#90451=CARTESIAN_POINT('Ctrl Pts',(21.4409833846734,18.4426974185065,171.644353546022));
#90452=CARTESIAN_POINT('Ctrl Pts',(21.4489871451359,18.4506208105774,171.661157055623));
#90453=CARTESIAN_POINT('Ctrl Pts',(21.4573442130695,18.4588939974157,171.677603438498));
#90454=CARTESIAN_POINT('Ctrl Pts',(21.4757377303701,18.4771028963323,171.713801161234));
#90455=CARTESIAN_POINT('Ctrl Pts',(21.4958432302445,18.497006759284,171.748272860834));
#90456=CARTESIAN_POINT('Ctrl Pts',(21.5175216452097,18.5184678018636,171.78069958324));
#90457=CARTESIAN_POINT('Ctrl Pts',(21.5271409181195,18.5279906210289,171.795088157907));
#90458=CARTESIAN_POINT('Ctrl Pts',(21.5370700702229,18.5378202177446,171.809073466704));
#90459=CARTESIAN_POINT('Ctrl Pts',(21.547297552772,18.5479451527243,171.8226244363));
#90460=CARTESIAN_POINT('Ctrl Pts',(21.547411296165,18.5480577556501,171.822775141349));
#90461=CARTESIAN_POINT('Ctrl Pts',(21.5475250755806,18.5481703942374,171.822925793229));
#90462=CARTESIAN_POINT('Ctrl Pts',(21.5476388910036,18.5482830684709,171.82307639192));
#90463=CARTESIAN_POINT('Ctrl Pts',(21.6089370659646,18.6089666269991,171.904185126494));
#90464=CARTESIAN_POINT('Ctrl Pts',(21.6800387968247,18.6793554444288,171.969901908548));
#90465=CARTESIAN_POINT('Ctrl Pts',(21.757287760541,18.7558298584533,172.017635952684));
#90466=CARTESIAN_POINT('Ctrl Pts',(21.767078251159,18.7655221830751,172.02368573884));
#90467=CARTESIAN_POINT('Ctrl Pts',(21.776967510281,18.7753122858817,172.029446612593));
#90468=CARTESIAN_POINT('Ctrl Pts',(21.7869481132028,18.7851928166143,172.034913246513));
#90469=CARTESIAN_POINT('Ctrl Pts',(21.7870212219941,18.785265192368,172.034953290086));
#90470=CARTESIAN_POINT('Ctrl Pts',(21.7870943346886,18.7853375719858,172.034993317412));
#90471=CARTESIAN_POINT('Ctrl Pts',(21.7871674512835,18.7854099554649,172.035033328492));
#90472=CARTESIAN_POINT('Ctrl Pts',(21.8164243108428,18.8143734662146,172.051043353842));
#90473=CARTESIAN_POINT('Ctrl Pts',(21.8462312070523,18.8438814985796,172.064416117585));
#90474=CARTESIAN_POINT('Ctrl Pts',(21.8764714094513,18.8738184925171,172.07518031916));
#90475=CARTESIAN_POINT('Ctrl Pts',(21.9072499164823,18.9042883936849,172.086136133856));
#90476=CARTESIAN_POINT('Ctrl Pts',(21.9384778938109,18.9352032584609,172.094389922825));
#90477=CARTESIAN_POINT('Ctrl Pts',(21.9700412343799,18.9664501239016,172.09991854538));
#90478=CARTESIAN_POINT('Ctrl Pts',(22.001604574949,18.9976969893423,172.105447167935));
#90479=CARTESIAN_POINT('Ctrl Pts',(22.03350392535,19.029276495556,172.108250749037));
#90480=CARTESIAN_POINT('Ctrl Pts',(22.0656246253921,19.0610751320115,172.108250755187));
#90481=CARTESIAN_POINT('Origin',(38.5483451826112,23.5078207102358,172.108250755187));
#90482=CARTESIAN_POINT('',(38.1965776692254,23.8631510023956,172.108250755187));
#90483=CARTESIAN_POINT('',(27.5329960959723,12.6029188688252,171.608250755187));
#90484=CARTESIAN_POINT('Origin',(32.2615249200093,29.8583152717307,172.108250755187));
#90485=CARTESIAN_POINT('',(32.2615249200093,29.8583152717307,171.608250755187));
#90486=CARTESIAN_POINT('',(21.5979433467562,18.5980831381603,172.108250755187));
#90487=CARTESIAN_POINT('Origin',(35.4049350513103,26.6830679909832,173.108250755187));
#90488=CARTESIAN_POINT('Origin',(35.4049350513103,26.6830679909832,153.108250755187));
#90489=CARTESIAN_POINT('Origin',(14.0868850299881,5.57876697388923,153.108250755187));
#90490=CARTESIAN_POINT('',(11.2952424120729,8.39868396247686,153.108250755187));
#90491=CARTESIAN_POINT('',(16.8785276479032,2.7588499853016,153.108250755187));
#90492=CARTESIAN_POINT('Origin',(32.6132924333951,29.5029849795709,153.108250755187));
#90493=CARTESIAN_POINT('Origin',(38.1965776692254,23.8631510023956,153.108250755187));
#90494=CARTESIAN_POINT('Origin',(35.4049350513103,26.6830679909832,171.608250755187));
#90495=CARTESIAN_POINT('Origin',(-32.1551898441603,24.2184812945555,172.608250755187));
#90496=CARTESIAN_POINT('',(-53.4732398654825,3.11418027746144,173.108250755187));
#90497=CARTESIAN_POINT('',(-53.1214723520968,2.75884998530159,172.608250755187));
#90498=CARTESIAN_POINT('Origin',(-53.4732398654825,3.11418027746144,172.608250755187));
#90499=CARTESIAN_POINT('',(-31.8034223307746,23.8631510023956,172.608250755187));
#90500=CARTESIAN_POINT('',(-32.1551898441603,24.2184812945555,173.108250755187));
#90501=CARTESIAN_POINT('Origin',(-55.9131149700119,5.57876697388922,172.608250755187));
#90502=CARTESIAN_POINT('',(-58.3529900745414,8.04335367031699,173.108250755187));
#90503=CARTESIAN_POINT('',(-58.7047575879271,8.39868396247685,172.608250755187));
#90504=CARTESIAN_POINT('Origin',(-58.3529900745414,8.04335367031699,172.608250755187));
#90505=CARTESIAN_POINT('Origin',(-55.9131149700119,5.57876697388922,172.608250755187));
#90506=CARTESIAN_POINT('Origin',(-55.9131149700119,5.57876697388922,173.108250755187));
#90507=CARTESIAN_POINT('Origin',(-37.0349400532192,29.147654687411,172.608250755187));
#90508=CARTESIAN_POINT('',(-37.3867075666049,29.5029849795709,172.608250755187));
#90509=CARTESIAN_POINT('',(-37.0349400532192,29.147654687411,173.108250755187));
#90510=CARTESIAN_POINT('Origin',(-34.5950649486897,26.6830679909832,152.608250755187));
#90511=CARTESIAN_POINT('',(-48.4989068541589,17.798633272459,153.108250755187));
#90512=CARTESIAN_POINT('Origin',(-48.4989068541589,17.798633272459,152.608250755187));
#90513=CARTESIAN_POINT('',(-43.6191566451,12.8694598796034,153.108250755187));
#90514=CARTESIAN_POINT('Origin',(-43.6191566451,12.8694598796034,152.608250755187));
#90515=CARTESIAN_POINT('Origin',(-34.5950649486897,26.6830679909832,153.108250755187));
#90516=CARTESIAN_POINT('Ctrl Pts',(-42.4926593451348,12.768040044578,153.608250755187));
#90517=CARTESIAN_POINT('Ctrl Pts',(-42.8220595622842,12.9549939852504,153.608250755187));
#90518=CARTESIAN_POINT('Ctrl Pts',(-43.0912266834094,12.6885257134127,153.608250755187));
#90519=CARTESIAN_POINT('Ctrl Pts',(-42.4926593657982,12.7680400563057,153.475551801171));
#90520=CARTESIAN_POINT('Ctrl Pts',(-42.8220595770889,12.954993994298,153.527723751245));
#90521=CARTESIAN_POINT('Ctrl Pts',(-43.091226688129,12.6885257087404,153.541901279333));
#90522=CARTESIAN_POINT('Ctrl Pts',(-42.516334861811,12.7814084763897,153.342399703391));
#90523=CARTESIAN_POINT('Ctrl Pts',(-42.8393599279114,12.9655349563554,153.446619353193));
#90524=CARTESIAN_POINT('Ctrl Pts',(-43.1061533482757,12.6927270912809,153.475325227732));
#90525=CARTESIAN_POINT('Ctrl Pts',(-42.605696122326,12.8327090607542,153.098820706789));
#90526=CARTESIAN_POINT('Ctrl Pts',(-42.9019404776233,13.0041108087007,153.3049590945));
#90527=CARTESIAN_POINT('Ctrl Pts',(-43.1622755982328,12.7092343374352,153.353535732545));
#90528=CARTESIAN_POINT('Ctrl Pts',(-42.6714790802343,12.8707492134964,152.987832794725));
#90529=CARTESIAN_POINT('Ctrl Pts',(-42.947776152444,13.0325418769712,153.243730625338));
#90530=CARTESIAN_POINT('Ctrl Pts',(-43.2035187758124,12.7215983775455,153.298041773782));
#90531=CARTESIAN_POINT('Ctrl Pts',(-42.8311845880579,12.9653805575584,152.805062971569));
#90532=CARTESIAN_POINT('Ctrl Pts',(-43.052608043633,13.0985506777718,153.152596157915));
#90533=CARTESIAN_POINT('Ctrl Pts',(-43.303060007586,12.7533719782572,153.206656864552));
#90534=CARTESIAN_POINT('Ctrl Pts',(-42.9264438528075,13.0228217613015,152.731827736181));
#90535=CARTESIAN_POINT('Ctrl Pts',(-43.112910695034,13.1369984402745,153.1222986856));
#90536=CARTESIAN_POINT('Ctrl Pts',(-43.3621762677728,12.7730921439476,153.170039246316));
#90537=CARTESIAN_POINT('Ctrl Pts',(-43.1289947753635,13.1484367358318,152.633922888492));
#90538=CARTESIAN_POINT('Ctrl Pts',(-43.2320211493329,13.2138353374619,153.093277185672));
#90539=CARTESIAN_POINT('Ctrl Pts',(-43.4869794975497,12.8177036267268,153.121086821207));
#90540=CARTESIAN_POINT('Ctrl Pts',(-43.2390141265139,13.2183592414294,152.608250765972));
#90541=CARTESIAN_POINT('Ctrl Pts',(-43.2924143454201,13.2532442939382,153.094953472492));
#90542=CARTESIAN_POINT('Ctrl Pts',(-43.5543441470683,12.8432444717964,153.108250755187));
#90543=CARTESIAN_POINT('Ctrl Pts',(-43.3456993209664,13.2880540647967,152.608250755187));
#90544=CARTESIAN_POINT('Ctrl Pts',(-43.3456993209664,13.2880540647967,153.108250755187));
#90545=CARTESIAN_POINT('Ctrl Pts',(-43.6191566451,12.8694598796034,153.108250755187));
#90546=CARTESIAN_POINT('',(-43.0912266834095,12.6885257134127,153.608250755187));
#90547=CARTESIAN_POINT('Origin',(-42.7394591700237,12.3331954212528,153.608250755187));
#90548=CARTESIAN_POINT('Ctrl Pts',(-43.0912266834094,12.6885257134127,153.608250755187));
#90549=CARTESIAN_POINT('Ctrl Pts',(-43.0912266834094,12.6885257134127,153.585611929926));
#90550=CARTESIAN_POINT('Ctrl Pts',(-43.0929604304944,12.6890138059483,153.563154237037));
#90551=CARTESIAN_POINT('Ctrl Pts',(-43.0962864633818,12.6899636529501,153.541035429073));
#90552=CARTESIAN_POINT('Ctrl Pts',(-43.0997704532087,12.6909586092248,153.517866174726));
#90553=CARTESIAN_POINT('Ctrl Pts',(-43.1050015895489,12.6924601686109,153.495067766215));
#90554=CARTESIAN_POINT('Ctrl Pts',(-43.1118701614209,12.6944521653039,153.472807844568));
#90555=CARTESIAN_POINT('Ctrl Pts',(-43.11348251584,12.6949197741068,153.46758246676));
#90556=CARTESIAN_POINT('Ctrl Pts',(-43.1151853191043,12.695414468869,153.46238674341));
#90557=CARTESIAN_POINT('Ctrl Pts',(-43.1169775445928,12.6959361508754,153.457222835554));
#90558=CARTESIAN_POINT('Ctrl Pts',(-43.1220257178005,12.6974055759807,153.442677622656));
#90559=CARTESIAN_POINT('Ctrl Pts',(-43.1277833978846,12.6990891411541,153.428386396435));
#90560=CARTESIAN_POINT('Ctrl Pts',(-43.1342144732543,12.700980714358,153.414430480138));
#90561=CARTESIAN_POINT('Ctrl Pts',(-43.1367991234315,12.7017409379188,153.408821595238));
#90562=CARTESIAN_POINT('Ctrl Pts',(-43.1394928923291,12.7025352357298,153.40326444683));
#90563=CARTESIAN_POINT('Ctrl Pts',(-43.1422910092109,12.7033627973937,153.397762970209));
#90564=CARTESIAN_POINT('Ctrl Pts',(-43.1565286871827,12.7075736852767,153.369769767703));
#90565=CARTESIAN_POINT('Ctrl Pts',(-43.1734608936206,12.7126442230623,153.343230009333));
#90566=CARTESIAN_POINT('Ctrl Pts',(-43.1925111334509,12.7184791208895,153.318537883333));
#90567=CARTESIAN_POINT('Ctrl Pts',(-43.210950781292,12.7241270005005,153.294637181192));
#90568=CARTESIAN_POINT('Ctrl Pts',(-43.2313748183461,12.7304910090136,153.272467520466));
#90569=CARTESIAN_POINT('Ctrl Pts',(-43.2532881748755,12.7374867495036,153.252349061816));
#90570=CARTESIAN_POINT('Ctrl Pts',(-43.2552948382388,12.738127367755,153.250506761946));
#90571=CARTESIAN_POINT('Ctrl Pts',(-43.2573153404985,12.7387737898784,153.248680454799));
#90572=CARTESIAN_POINT('Ctrl Pts',(-43.2593492166407,12.7394259068856,153.246870287867));
#90573=CARTESIAN_POINT('Ctrl Pts',(-43.2780390336002,12.7454183797058,153.230236193034));
#90574=CARTESIAN_POINT('Ctrl Pts',(-43.2978344867151,12.7518833303144,153.214981265976));
#90575=CARTESIAN_POINT('Ctrl Pts',(-43.3184548140972,12.7587610622881,153.201166192581));
#90576=CARTESIAN_POINT('Ctrl Pts',(-43.3403128175315,12.7660516104115,153.186521908999));
#90577=CARTESIAN_POINT('Ctrl Pts',(-43.3630987741874,12.7738061414832,153.173494523169));
#90578=CARTESIAN_POINT('Ctrl Pts',(-43.3865244412286,12.7819706583749,153.162187747801));
#90579=CARTESIAN_POINT('Ctrl Pts',(-43.3990387034681,12.786332237717,153.156147537642));
#90580=CARTESIAN_POINT('Ctrl Pts',(-43.4117361909291,12.7908110879773,153.150598972776));
#90581=CARTESIAN_POINT('Ctrl Pts',(-43.424576119712,12.7954005301352,153.145562771898));
#90582=CARTESIAN_POINT('Ctrl Pts',(-43.4487637897704,12.804046054152,153.136075650339));
#90583=CARTESIAN_POINT('Ctrl Pts',(-43.473708893918,12.813181182582,153.128328353011));
#90584=CARTESIAN_POINT('Ctrl Pts',(-43.4990632915912,12.8226927418291,153.122388238269));
#90585=CARTESIAN_POINT('Ctrl Pts',(-43.5226529740675,12.831542278126,153.116861567022));
#90586=CARTESIAN_POINT('Ctrl Pts',(-43.5465984295517,12.8407182262666,153.112899483271));
#90587=CARTESIAN_POINT('Ctrl Pts',(-43.5706101237033,12.8501313371678,153.1105979981));
#90588=CARTESIAN_POINT('Ctrl Pts',(-43.5867944322199,12.8564759411747,153.1090467562));
#90589=CARTESIAN_POINT('Ctrl Pts',(-43.6030086326662,12.8629283194247,153.108250755187));
#90590=CARTESIAN_POINT('Ctrl Pts',(-43.6191566451001,12.8694598796034,153.108250755187));
#90591=CARTESIAN_POINT('Ctrl Pts',(-48.0775783115689,18.0678585669597,152.608250755187));
#90592=CARTESIAN_POINT('Ctrl Pts',(-48.0775783115689,18.0678585669597,153.108250755187));
#90593=CARTESIAN_POINT('Ctrl Pts',(-48.4989068541589,17.798633272459,153.108250755187));
#90594=CARTESIAN_POINT('Ctrl Pts',(-48.1470307749619,18.1765493392547,152.60825077749));
#90595=CARTESIAN_POINT('Ctrl Pts',(-48.1122768724314,18.1221606460454,153.094787604517));
#90596=CARTESIAN_POINT('Ctrl Pts',(-48.5247812179203,17.864504504826,153.108250755187));
#90597=CARTESIAN_POINT('Ctrl Pts',(-48.214837800552,18.2856761107432,152.633710236017));
#90598=CARTESIAN_POINT('Ctrl Pts',(-48.150528898798,18.1820886305035,153.093185957657));
#90599=CARTESIAN_POINT('Ctrl Pts',(-48.5492718500596,17.9311502346665,153.120980492262));
#90600=CARTESIAN_POINT('Ctrl Pts',(-48.3392719415066,18.4909268139009,152.732462696752));
#90601=CARTESIAN_POINT('Ctrl Pts',(-48.2267098579281,18.3028399523544,153.122507989483));
#90602=CARTESIAN_POINT('Ctrl Pts',(-48.5929236463666,18.0572865403011,153.170356729309));
#90603=CARTESIAN_POINT('Ctrl Pts',(-48.3952620045917,18.5859573989267,152.805334639289));
#90604=CARTESIAN_POINT('Ctrl Pts',(-48.2642585375815,18.3630692431352,153.152707467858));
#90605=CARTESIAN_POINT('Ctrl Pts',(-48.6118750907876,18.1161056718007,153.206792695945));
#90606=CARTESIAN_POINT('Ctrl Pts',(-48.488400449801,18.7468303826905,152.988630571688));
#90607=CARTESIAN_POINT('Ctrl Pts',(-48.3293052637564,18.468724748985,153.244147548452));
#90608=CARTESIAN_POINT('Ctrl Pts',(-48.6426808681032,18.2161018881961,153.29844066473));
#90609=CARTESIAN_POINT('Ctrl Pts',(-48.5257065468464,18.8128807906121,153.099898214101));
#90610=CARTESIAN_POINT('Ctrl Pts',(-48.357233870597,18.5147847472079,153.30558183398));
#90611=CARTESIAN_POINT('Ctrl Pts',(-48.6546039643613,18.2573986678045,153.354074484501));
#90612=CARTESIAN_POINT('Ctrl Pts',(-48.5757943506347,18.9022051021532,153.342371533405));
#90613=CARTESIAN_POINT('Ctrl Pts',(-48.3949466240771,18.5773697525719,153.446616730793));
#90614=CARTESIAN_POINT('Ctrl Pts',(-48.6704461232433,18.3133407705919,153.475311144438));
#90615=CARTESIAN_POINT('Ctrl Pts',(-48.5889699010307,18.926095373728,153.475893601961));
#90616=CARTESIAN_POINT('Ctrl Pts',(-48.4053447967376,18.5948279601089,153.527930080756));
#90617=CARTESIAN_POINT('Ctrl Pts',(-48.6745119199733,18.3283596898617,153.542072178464));
#90618=CARTESIAN_POINT('Ctrl Pts',(-48.5889699028093,18.9260953769367,153.608250755187));
#90619=CARTESIAN_POINT('Ctrl Pts',(-48.4053447981146,18.5948279624256,153.608250755187));
#90620=CARTESIAN_POINT('Ctrl Pts',(-48.6745119192398,18.3283596905879,153.608250755187));
#90621=CARTESIAN_POINT('',(-48.6745119192398,18.3283596905879,153.608250755187));
#90622=CARTESIAN_POINT('Origin',(-49.0262794326256,18.6836899827478,153.608250755187));
#90623=CARTESIAN_POINT('Ctrl Pts',(-48.4989068541589,17.798633272459,153.108250755187));
#90624=CARTESIAN_POINT('Ctrl Pts',(-48.5094269497017,17.8254154443576,153.108250755187));
#90625=CARTESIAN_POINT('Ctrl Pts',(-48.5196536306266,17.8521593410513,153.110350857061));
#90626=CARTESIAN_POINT('Ctrl Pts',(-48.5295390298831,17.8786538140997,153.114447252937));
#90627=CARTESIAN_POINT('Ctrl Pts',(-48.5396860002682,17.9058493401896,153.118652040883));
#90628=CARTESIAN_POINT('Ctrl Pts',(-48.5494737553264,17.9327832400945,153.124960207407));
#90629=CARTESIAN_POINT('Ctrl Pts',(-48.5588463302412,17.9592354635869,153.133312849708));
#90630=CARTESIAN_POINT('Ctrl Pts',(-48.5630141439483,17.9709982865737,153.13702711792));
#90631=CARTESIAN_POINT('Ctrl Pts',(-48.5670997707517,17.9826658616072,153.141146354448));
#90632=CARTESIAN_POINT('Ctrl Pts',(-48.5710977355924,17.994218395715,153.145668609543));
#90633=CARTESIAN_POINT('Ctrl Pts',(-48.5799936089787,18.0199239446154,153.155731081411));
#90634=CARTESIAN_POINT('Ctrl Pts',(-48.5884215305909,18.0449504539237,153.167751327948));
#90635=CARTESIAN_POINT('Ctrl Pts',(-48.5963532588931,18.0690479409521,153.18163170246));
#90636=CARTESIAN_POINT('Ctrl Pts',(-48.6039268974369,18.0920575108232,153.194885426667));
#90637=CARTESIAN_POINT('Ctrl Pts',(-48.6110482072602,18.1142208889207,153.209835861399));
#90638=CARTESIAN_POINT('Ctrl Pts',(-48.6176800176114,18.1352871692251,153.226428438643));
#90639=CARTESIAN_POINT('Ctrl Pts',(-48.6202694448921,18.143512615677,153.232907102823));
#90640=CARTESIAN_POINT('Ctrl Pts',(-48.6227840994235,18.15157036769,153.23963640177));
#90641=CARTESIAN_POINT('Ctrl Pts',(-48.6252211735162,18.1594436001053,153.246614074428));
#90642=CARTESIAN_POINT('Ctrl Pts',(-48.6259132243274,18.1616793453769,153.248595509476));
#90643=CARTESIAN_POINT('Ctrl Pts',(-48.6265988211803,18.1638995706234,153.250596415344));
#90644=CARTESIAN_POINT('Ctrl Pts',(-48.6272778897841,18.1661038480101,153.252616665764));
#90645=CARTESIAN_POINT('Ctrl Pts',(-48.6342798979749,18.1888325800255,153.273447860004));
#90646=CARTESIAN_POINT('Ctrl Pts',(-48.6406027699211,18.2098942489154,153.29642453625));
#90647=CARTESIAN_POINT('Ctrl Pts',(-48.6461749021359,18.2287912078335,153.321170461484));
#90648=CARTESIAN_POINT('Ctrl Pts',(-48.6514488684785,18.2466769868256,153.344592227475));
#90649=CARTESIAN_POINT('Ctrl Pts',(-48.6560502790058,18.2626236397099,153.369599261704));
#90650=CARTESIAN_POINT('Ctrl Pts',(-48.6599104487583,18.2761669413009,153.395852653178));
#90651=CARTESIAN_POINT('Ctrl Pts',(-48.6608238217216,18.2793714857378,153.402064591901));
#90652=CARTESIAN_POINT('Ctrl Pts',(-48.6616956587186,18.2824412753048,153.408346207002));
#90653=CARTESIAN_POINT('Ctrl Pts',(-48.6625249804952,18.2853697768896,153.414692806039));
#90654=CARTESIAN_POINT('Ctrl Pts',(-48.6659464217758,18.2974515725152,153.440876268898));
#90655=CARTESIAN_POINT('Ctrl Pts',(-48.6686720763068,18.3072005590288,153.468385102503));
#90656=CARTESIAN_POINT('Ctrl Pts',(-48.6706554188086,18.3143466012101,153.496722756822));
#90657=CARTESIAN_POINT('Ctrl Pts',(-48.6725475333005,18.3211639461509,153.523756961128));
#90658=CARTESIAN_POINT('Ctrl Pts',(-48.6737640367869,18.3256122792063,153.551545730225));
#90659=CARTESIAN_POINT('Ctrl Pts',(-48.6742591562215,18.3274298612422,153.579619100719));
#90660=CARTESIAN_POINT('Ctrl Pts',(-48.6744270219174,18.3280460957343,153.589137119091));
#90661=CARTESIAN_POINT('Ctrl Pts',(-48.6745119192398,18.3283596905879,153.598687494766));
#90662=CARTESIAN_POINT('Ctrl Pts',(-48.6745119192398,18.3283596905879,153.608250755187));
#90663=CARTESIAN_POINT('Origin',(-42.7394591700237,12.3331954212528,171.608250755187));
#90664=CARTESIAN_POINT('',(-43.0912266834095,12.6885257134127,171.108250755187));
#90665=CARTESIAN_POINT('Origin',(-42.7394591700237,12.3331954212528,171.108250755187));
#90666=CARTESIAN_POINT('',(-43.0912266834095,12.6885257134127,153.108250755187));
#90667=CARTESIAN_POINT('Origin',(-32.1551898441603,24.2184812945555,153.608250755187));
#90668=CARTESIAN_POINT('',(-53.1214723520968,2.75884998530159,153.608250755187));
#90669=CARTESIAN_POINT('',(-53.4732398654825,3.11418027746144,153.108250755187));
#90670=CARTESIAN_POINT('Origin',(-53.4732398654825,3.11418027746144,153.608250755187));
#90671=CARTESIAN_POINT('',(-53.4732398654825,3.11418027746144,153.108250755187));
#90672=CARTESIAN_POINT('',(-42.8187714174134,12.9582491609851,153.608250755187));
#90673=CARTESIAN_POINT('Origin',(-37.0349400532192,29.147654687411,153.608250755187));
#90674=CARTESIAN_POINT('',(-58.3529900745414,8.04335367031699,153.108250755187));
#90675=CARTESIAN_POINT('',(-58.7047575879271,8.39868396247685,153.608250755187));
#90676=CARTESIAN_POINT('Origin',(-58.3529900745414,8.043353670317,153.608250755187));
#90677=CARTESIAN_POINT('',(-58.7047575879271,8.39868396247684,153.608250755187));
#90678=CARTESIAN_POINT('',(-48.050289139858,18.2427528460005,153.108250755187));
#90679=CARTESIAN_POINT('Origin',(-49.0262794326255,18.6836899827478,171.608250755187));
#90680=CARTESIAN_POINT('',(-48.6745119192398,18.3283596905879,171.108250755187));
#90681=CARTESIAN_POINT('Origin',(-49.0262794326256,18.6836899827478,171.108250755187));
#90682=CARTESIAN_POINT('',(-48.6745119192398,18.3283596905879,153.108250755187));
#90683=CARTESIAN_POINT('Ctrl Pts',(-43.0912266834094,12.6885257134127,171.108250755187));
#90684=CARTESIAN_POINT('Ctrl Pts',(-42.8220595622842,12.9549939852504,171.108250755187));
#90685=CARTESIAN_POINT('Ctrl Pts',(-42.4926593451348,12.768040044578,171.108250755187));
#90686=CARTESIAN_POINT('Ctrl Pts',(-43.0912266659252,12.6885257307216,171.241737242521));
#90687=CARTESIAN_POINT('Ctrl Pts',(-42.8220595499177,12.9549939974934,171.189238482122));
#90688=CARTESIAN_POINT('Ctrl Pts',(-42.4926593395179,12.76804004139,171.174993997722));
#90689=CARTESIAN_POINT('Ctrl Pts',(-43.0710441707684,12.7085058627055,171.375809742194));
#90690=CARTESIAN_POINT('Ctrl Pts',(-42.8075773954216,12.9693309442371,171.270872142595));
#90691=CARTESIAN_POINT('Ctrl Pts',(-42.4794414677661,12.7762529890484,171.242030250225));
#90692=CARTESIAN_POINT('Ctrl Pts',(-42.9945373856677,12.7842455396928,171.620480252948));
#90693=CARTESIAN_POINT('Ctrl Pts',(-42.7541636542667,13.0222091235587,171.414405744627));
#90694=CARTESIAN_POINT('Ctrl Pts',(-42.4291554349937,12.807315162219,171.364365502532));
#90695=CARTESIAN_POINT('Ctrl Pts',(-42.9380439148113,12.840172569288,171.731805299994));
#90696=CARTESIAN_POINT('Ctrl Pts',(-42.7146746820777,13.061302152944,171.477100056791));
#90697=CARTESIAN_POINT('Ctrl Pts',(-42.3919659144686,12.83022887921,171.420028028856));
#90698=CARTESIAN_POINT('Ctrl Pts',(-42.8001863975324,12.976647835047,171.914243767979));
#90699=CARTESIAN_POINT('Ctrl Pts',(-42.6221241181486,13.1529247431198,171.570720798637));
#90700=CARTESIAN_POINT('Ctrl Pts',(-42.300709976456,12.8859483002507,171.511247260317));
#90701=CARTESIAN_POINT('Ctrl Pts',(-42.7176862192175,13.0583208114862,171.986819299416));
#90702=CARTESIAN_POINT('Ctrl Pts',(-42.5677125765317,13.2067907182888,171.602133212335));
#90703=CARTESIAN_POINT('Ctrl Pts',(-42.245878978066,12.9192082849093,171.547535027057));
#90704=CARTESIAN_POINT('Ctrl Pts',(-42.5412347367947,13.2330030735242,172.083342412463));
#90705=CARTESIAN_POINT('Ctrl Pts',(-42.4580034693628,13.3153998086923,171.630196458045));
#90706=CARTESIAN_POINT('Ctrl Pts',(-42.1278002879233,12.9900408536815,171.595796584069));
#90707=CARTESIAN_POINT('Ctrl Pts',(-42.4450880381951,13.3281857411236,172.108250746497));
#90708=CARTESIAN_POINT('Ctrl Pts',(-42.4010685331158,13.3717638772503,171.626173327528));
#90709=CARTESIAN_POINT('Ctrl Pts',(-42.0630761456614,13.0284859943164,171.608250755187));
#90710=CARTESIAN_POINT('Ctrl Pts',(-42.3510901387775,13.4212411548363,172.108250755187));
#90711=CARTESIAN_POINT('Ctrl Pts',(-42.3510901387775,13.4212411548362,171.608250755187));
#90712=CARTESIAN_POINT('Ctrl Pts',(-41.9993226253918,13.0659108626764,171.608250755187));
#90713=CARTESIAN_POINT('',(-42.3510901387776,13.4212411548362,172.108250755187));
#90714=CARTESIAN_POINT('Origin',(-41.9993226253918,13.0659108626764,172.108250755187));
#90715=CARTESIAN_POINT('Ctrl Pts',(-42.3510901387776,13.4212411548362,172.108250755187));
#90716=CARTESIAN_POINT('Ctrl Pts',(-42.3778802251244,13.3947196837837,172.10825075271));
#90717=CARTESIAN_POINT('Ctrl Pts',(-42.404633334338,13.368234819107,172.106231383602));
#90718=CARTESIAN_POINT('Ctrl Pts',(-42.4311963424757,13.3419381494253,172.102298699113));
#90719=CARTESIAN_POINT('Ctrl Pts',(-42.4585393123223,13.3148693384515,172.098250540379));
#90720=CARTESIAN_POINT('Ctrl Pts',(-42.4856817817057,13.2879990175887,172.092175073614));
#90721=CARTESIAN_POINT('Ctrl Pts',(-42.512470190444,13.2614792073225,172.084134831717));
#90722=CARTESIAN_POINT('Ctrl Pts',(-42.5392868384809,13.2349314409038,172.076086114109));
#90723=CARTESIAN_POINT('Ctrl Pts',(-42.5657496804913,13.2087339330164,172.066068297245));
#90724=CARTESIAN_POINT('Ctrl Pts',(-42.591703228735,13.183040612378,172.054093236376));
#90725=CARTESIAN_POINT('Ctrl Pts',(-42.6044176951968,13.1704536296472,172.048226735644));
#90726=CARTESIAN_POINT('Ctrl Pts',(-42.6170098178969,13.157987763978,172.041889749803));
#90727=CARTESIAN_POINT('Ctrl Pts',(-42.6294600760868,13.1456623403912,172.035079401128));
#90728=CARTESIAN_POINT('Ctrl Pts',(-42.6296843310279,13.1454403339798,172.034956732641));
#90729=CARTESIAN_POINT('Ctrl Pts',(-42.6299085540949,13.1452183591231,172.034833904296));
#90730=CARTESIAN_POINT('Ctrl Pts',(-42.6301327452084,13.1449964158994,172.034710916136));
#90731=CARTESIAN_POINT('Ctrl Pts',(-42.7180977048726,13.0579134516646,171.98645454965));
#90732=CARTESIAN_POINT('Ctrl Pts',(-42.8003616294977,12.9764743600703,171.914009179875));
#90733=CARTESIAN_POINT('Ctrl Pts',(-42.8691146789652,12.908410674588,171.823023819991));
#90734=CARTESIAN_POINT('Ctrl Pts',(-42.8692314898414,12.9082950349356,171.822869236599));
#90735=CARTESIAN_POINT('Ctrl Pts',(-42.8693482649874,12.9081794306552,171.822714595501));
#90736=CARTESIAN_POINT('Ctrl Pts',(-42.8694650043749,12.9080638617748,171.822559896743));
#90737=CARTESIAN_POINT('Ctrl Pts',(-42.9382343475108,12.8399840459953,171.731429283186));
#90738=CARTESIAN_POINT('Ctrl Pts',(-42.9946005532137,12.7841830055056,171.620275542505));
#90739=CARTESIAN_POINT('Ctrl Pts',(-43.0327904247401,12.7463760511325,171.498144778716));
#90740=CARTESIAN_POINT('Ctrl Pts',(-43.0328228387206,12.7463439621562,171.498041119184));
#90741=CARTESIAN_POINT('Ctrl Pts',(-43.0328552397283,12.7463118860226,171.497937451222));
#90742=CARTESIAN_POINT('Ctrl Pts',(-43.0328876277619,12.7462798227331,171.497833774838));
#90743=CARTESIAN_POINT('Ctrl Pts',(-43.0439348683491,12.7353433491568,171.462470776879));
#90744=CARTESIAN_POINT('Ctrl Pts',(-43.053439241226,12.7259342734689,171.426245512341));
#90745=CARTESIAN_POINT('Ctrl Pts',(-43.061393897703,12.7180593756894,171.389360653077));
#90746=CARTESIAN_POINT('Ctrl Pts',(-43.0693558306946,12.7101772743544,171.352442053422));
#90747=CARTESIAN_POINT('Ctrl Pts',(-43.0757654021736,12.7038319695189,171.314861536722));
#90748=CARTESIAN_POINT('Ctrl Pts',(-43.0805808169241,12.6990648373321,171.276805373266));
#90749=CARTESIAN_POINT('Ctrl Pts',(-43.08526166173,12.6944309258018,171.239812714425));
#90750=CARTESIAN_POINT('Ctrl Pts',(-43.0884362406313,12.6912881773483,171.202369605247));
#90751=CARTESIAN_POINT('Ctrl Pts',(-43.0900317766283,12.6897086392606,171.164646810896));
#90752=CARTESIAN_POINT('Ctrl Pts',(-43.0908242882833,12.6889240738566,171.145909687925));
#90753=CARTESIAN_POINT('Ctrl Pts',(-43.0912266809401,12.6885257158573,171.127103649709));
#90754=CARTESIAN_POINT('Ctrl Pts',(-43.0912266834094,12.6885257134127,171.108250755187));
#90755=CARTESIAN_POINT('Origin',(-55.9131149700119,5.57876697388922,153.608250755187));
#90756=CARTESIAN_POINT('Origin',(-55.9131149700119,5.57876697388922,153.608250755187));
#90757=CARTESIAN_POINT('Origin',(-55.9131149700119,5.57876697388922,153.108250755187));
#90758=CARTESIAN_POINT('Ctrl Pts',(-47.9343753746079,19.0610751320115,172.108250755187));
#90759=CARTESIAN_POINT('Ctrl Pts',(-47.9343753746079,19.0610751320115,171.608250755187));
#90760=CARTESIAN_POINT('Ctrl Pts',(-48.2861428879937,19.4164054241714,171.608250755187));
#90761=CARTESIAN_POINT('Ctrl Pts',(-48.0295598492238,18.9668450404957,172.108250736963));
#90762=CARTESIAN_POINT('Ctrl Pts',(-47.9849859451505,19.0109720168265,171.626400023775));
#90763=CARTESIAN_POINT('Ctrl Pts',(-48.32468689732,19.3522354702212,171.608250755187));
#90764=CARTESIAN_POINT('Ctrl Pts',(-48.1241811156121,18.8731725101058,172.083590099036));
#90765=CARTESIAN_POINT('Ctrl Pts',(-48.0410594303009,18.9554607618994,171.630295894894));
#90766=CARTESIAN_POINT('Ctrl Pts',(-48.3631650925245,19.2889233489514,171.595920429989));
#90767=CARTESIAN_POINT('Ctrl Pts',(-48.3019226666633,18.6972131145288,171.986236425372));
#90768=CARTESIAN_POINT('Ctrl Pts',(-48.151583977807,18.8460444073028,171.601943545762));
#90769=CARTESIAN_POINT('Ctrl Pts',(-48.43571109596,19.1707080971491,171.547243587402));
#90770=CARTESIAN_POINT('Ctrl Pts',(-48.3835682791724,18.616386135448,171.914220536541));
#90771=CARTESIAN_POINT('Ctrl Pts',(-48.2054676258018,18.7927010327451,171.570727890217));
#90772=CARTESIAN_POINT('Ctrl Pts',(-48.4691728514479,19.1167826550556,171.511235647295));
#90773=CARTESIAN_POINT('Ctrl Pts',(-48.5218367099866,18.4795040762473,171.73102847759));
#90774=CARTESIAN_POINT('Ctrl Pts',(-48.29830160884,18.7007978652082,171.476689446385));
#90775=CARTESIAN_POINT('Ctrl Pts',(-48.5259782937221,19.0258237386761,171.419639614957));
#90776=CARTESIAN_POINT('Ctrl Pts',(-48.5781352141625,18.4237700584665,171.619640310305));
#90777=CARTESIAN_POINT('Ctrl Pts',(-48.3376676770396,18.6618265074951,171.413915961973));
#90778=CARTESIAN_POINT('Ctrl Pts',(-48.5491857815886,18.9889959729155,171.363945533081));
#90779=CARTESIAN_POINT('Ctrl Pts',(-48.6542879371882,18.3483808934914,171.37578205691));
#90780=CARTESIAN_POINT('Ctrl Pts',(-48.390835760336,18.6091915229028,171.270846895347));
#90781=CARTESIAN_POINT('Ctrl Pts',(-48.5806071206517,18.9392570552066,171.242016405713));
#90782=CARTESIAN_POINT('Ctrl Pts',(-48.6745119175319,18.3283596922787,171.241710900385));
#90783=CARTESIAN_POINT('Ctrl Pts',(-48.4053447968997,18.5948279636275,171.189221495561));
#90784=CARTESIAN_POINT('Ctrl Pts',(-48.5889699031145,18.9260953774872,171.174980828039));
#90785=CARTESIAN_POINT('Ctrl Pts',(-48.6745119192398,18.3283596905879,171.108250755187));
#90786=CARTESIAN_POINT('Ctrl Pts',(-48.4053447981146,18.5948279624256,171.108250755187));
#90787=CARTESIAN_POINT('Ctrl Pts',(-48.5889699028093,18.9260953769367,171.108250755187));
#90788=CARTESIAN_POINT('',(-47.9343753746079,19.0610751320115,172.108250755187));
#90789=CARTESIAN_POINT('Origin',(-48.2861428879937,19.4164054241714,172.108250755187));
#90790=CARTESIAN_POINT('Ctrl Pts',(-48.6745119192398,18.3283596905879,171.108250755187));
#90791=CARTESIAN_POINT('Ctrl Pts',(-48.6745119187474,18.3283596910754,171.146726782702));
#90792=CARTESIAN_POINT('Ctrl Pts',(-48.6728035759767,18.3300508975484,171.185041427672));
#90793=CARTESIAN_POINT('Ctrl Pts',(-48.6694816577094,18.3333395380085,171.222986490344));
#90794=CARTESIAN_POINT('Ctrl Pts',(-48.6678077173449,18.3349967094278,171.242107301551));
#90795=CARTESIAN_POINT('Ctrl Pts',(-48.6657234606753,18.337060093891,171.261134517832));
#90796=CARTESIAN_POINT('Ctrl Pts',(-48.6632375537432,18.3395211258692,171.280042307355));
#90797=CARTESIAN_POINT('Ctrl Pts',(-48.6581085545367,18.34459880231,171.319053436939));
#90798=CARTESIAN_POINT('Ctrl Pts',(-48.6512741791919,18.3513648861228,171.357556066246));
#90799=CARTESIAN_POINT('Ctrl Pts',(-48.6428360068715,18.3597187358033,171.39531541567));
#90800=CARTESIAN_POINT('Ctrl Pts',(-48.6400900203536,18.3624372816831,171.407603226407));
#90801=CARTESIAN_POINT('Ctrl Pts',(-48.637173929816,18.3653242284384,171.419812520366));
#90802=CARTESIAN_POINT('Ctrl Pts',(-48.6340904613841,18.3683768672509,171.431935680483));
#90803=CARTESIAN_POINT('Ctrl Pts',(-48.6293809516382,18.3730392896352,171.450451887793));
#90804=CARTESIAN_POINT('Ctrl Pts',(-48.6242821293815,18.3780870998679,171.46876644342));
#90805=CARTESIAN_POINT('Ctrl Pts',(-48.6188057791329,18.3835085796861,171.486850966306));
#90806=CARTESIAN_POINT('Ctrl Pts',(-48.6177460918596,18.3845576493959,171.490350366066));
#90807=CARTESIAN_POINT('Ctrl Pts',(-48.6166722450822,18.3856207337022,171.493841420748));
#90808=CARTESIAN_POINT('Ctrl Pts',(-48.6155844631122,18.3866976107387,171.497323013247));
#90809=CARTESIAN_POINT('Ctrl Pts',(-48.6142128210569,18.3880555021843,171.501713138128));
#90810=CARTESIAN_POINT('Ctrl Pts',(-48.612818540126,18.3894358011566,171.506090294806));
#90811=CARTESIAN_POINT('Ctrl Pts',(-48.6114022744607,18.3908378605866,171.510452436845));
#90812=CARTESIAN_POINT('Ctrl Pts',(-48.5983298942098,18.4037791147954,171.550715772201));
#90813=CARTESIAN_POINT('Ctrl Pts',(-48.5833686358101,18.4185899911868,171.589744502643));
#90814=CARTESIAN_POINT('Ctrl Pts',(-48.5666542253237,18.4351365211253,171.627226319313));
#90815=CARTESIAN_POINT('Ctrl Pts',(-48.5590166153253,18.4426974185078,171.644353546025));
#90816=CARTESIAN_POINT('Ctrl Pts',(-48.5510128548635,18.450620810578,171.661157055624));
#90817=CARTESIAN_POINT('Ctrl Pts',(-48.5426557869305,18.4588939974157,171.677603438498));
#90818=CARTESIAN_POINT('Ctrl Pts',(-48.524262269629,18.4771028963332,171.713801161236));
#90819=CARTESIAN_POINT('Ctrl Pts',(-48.5041567697535,18.4970067592859,171.748272860838));
#90820=CARTESIAN_POINT('Ctrl Pts',(-48.4824783547872,18.5184678018667,171.780699583245));
#90821=CARTESIAN_POINT('Ctrl Pts',(-48.4728590818784,18.527990621031,171.79508815791));
#90822=CARTESIAN_POINT('Ctrl Pts',(-48.462929929776,18.5378202177457,171.809073466706));
#90823=CARTESIAN_POINT('Ctrl Pts',(-48.4527024472281,18.5479451527243,171.8226244363));
#90824=CARTESIAN_POINT('Ctrl Pts',(-48.4525887038351,18.5480577556501,171.822775141349));
#90825=CARTESIAN_POINT('Ctrl Pts',(-48.4524749244194,18.5481703942374,171.822925793229));
#90826=CARTESIAN_POINT('Ctrl Pts',(-48.4523611089964,18.5482830684709,171.82307639192));
#90827=CARTESIAN_POINT('Ctrl Pts',(-48.3910629342879,18.6089666267492,171.90418512616));
#90828=CARTESIAN_POINT('Ctrl Pts',(-48.3199612037609,18.679355443849,171.969901908007));
#90829=CARTESIAN_POINT('Ctrl Pts',(-48.2427122404135,18.7558298575084,172.017635952094));
#90830=CARTESIAN_POINT('Ctrl Pts',(-48.2329217494837,18.7655221824388,172.023685738466));
#90831=CARTESIAN_POINT('Ctrl Pts',(-48.2230324900434,18.7753122855606,172.029446612416));
#90832=CARTESIAN_POINT('Ctrl Pts',(-48.2130518867972,18.7851928166143,172.034913246513));
#90833=CARTESIAN_POINT('Ctrl Pts',(-48.2129787780059,18.785265192368,172.034953290086));
#90834=CARTESIAN_POINT('Ctrl Pts',(-48.2129056653114,18.7853375719858,172.034993317412));
#90835=CARTESIAN_POINT('Ctrl Pts',(-48.2128325487165,18.7854099554649,172.035033328492));
#90836=CARTESIAN_POINT('Ctrl Pts',(-48.1835756891614,18.8143734662104,172.051043353839));
#90837=CARTESIAN_POINT('Ctrl Pts',(-48.1537687929565,18.843881498571,172.064416117581));
#90838=CARTESIAN_POINT('Ctrl Pts',(-48.123528590562,18.873818492504,172.075180319155));
#90839=CARTESIAN_POINT('Ctrl Pts',(-48.0927500835289,18.9042883936738,172.086136133853));
#90840=CARTESIAN_POINT('Ctrl Pts',(-48.0615221061982,18.935203258452,172.094389922823));
#90841=CARTESIAN_POINT('Ctrl Pts',(-48.0299587656269,18.9664501238949,172.099918545379));
#90842=CARTESIAN_POINT('Ctrl Pts',(-47.9983954250556,18.9976969893378,172.105447167934));
#90843=CARTESIAN_POINT('Ctrl Pts',(-47.9664960746524,19.0292764955537,172.108250749037));
#90844=CARTESIAN_POINT('Ctrl Pts',(-47.9343753746079,19.0610751320115,172.108250755187));
#90845=CARTESIAN_POINT('Origin',(-31.4516548173888,23.5078207102358,172.108250755187));
#90846=CARTESIAN_POINT('',(-31.8034223307746,23.8631510023956,172.108250755187));
#90847=CARTESIAN_POINT('',(-42.4670039040277,12.6029188688252,171.608250755187));
#90848=CARTESIAN_POINT('Origin',(-37.7384750799907,29.8583152717307,172.108250755187));
#90849=CARTESIAN_POINT('',(-37.7384750799907,29.8583152717307,171.608250755187));
#90850=CARTESIAN_POINT('',(-48.4020566532438,18.5980831381603,172.108250755187));
#90851=CARTESIAN_POINT('Origin',(-34.5950649486897,26.6830679909832,173.108250755187));
#90852=CARTESIAN_POINT('Origin',(-34.5950649486897,26.6830679909832,153.108250755187));
#90853=CARTESIAN_POINT('Origin',(-55.9131149700119,5.57876697388922,153.108250755187));
#90854=CARTESIAN_POINT('',(-58.7047575879271,8.39868396247685,153.108250755187));
#90855=CARTESIAN_POINT('',(-53.1214723520968,2.75884998530159,153.108250755187));
#90856=CARTESIAN_POINT('Origin',(-37.3867075666049,29.5029849795709,153.108250755187));
#90857=CARTESIAN_POINT('Origin',(-31.8034223307746,23.8631510023956,153.108250755187));
#90858=CARTESIAN_POINT('Origin',(-34.5950649486897,26.6830679909832,171.608250755187));
#90859=CARTESIAN_POINT('Origin',(-102.15518984416,24.2184812945555,172.608250755187));
#90860=CARTESIAN_POINT('',(-123.473239865483,3.11418027746143,173.108250755187));
#90861=CARTESIAN_POINT('',(-123.121472352097,2.75884998530158,172.608250755187));
#90862=CARTESIAN_POINT('Origin',(-123.473239865483,3.11418027746143,172.608250755187));
#90863=CARTESIAN_POINT('',(-101.803422330775,23.8631510023956,172.608250755187));
#90864=CARTESIAN_POINT('',(-102.15518984416,24.2184812945555,173.108250755187));
#90865=CARTESIAN_POINT('Origin',(-125.913114970012,5.57876697388921,172.608250755187));
#90866=CARTESIAN_POINT('',(-128.352990074541,8.04335367031698,173.108250755187));
#90867=CARTESIAN_POINT('',(-128.704757587927,8.39868396247684,172.608250755187));
#90868=CARTESIAN_POINT('Origin',(-128.352990074541,8.04335367031698,172.608250755187));
#90869=CARTESIAN_POINT('Origin',(-125.913114970012,5.57876697388921,172.608250755187));
#90870=CARTESIAN_POINT('Origin',(-125.913114970012,5.57876697388921,173.108250755187));
#90871=CARTESIAN_POINT('Origin',(-107.034940053219,29.147654687411,172.608250755187));
#90872=CARTESIAN_POINT('',(-107.386707566605,29.5029849795709,172.608250755187));
#90873=CARTESIAN_POINT('',(-107.034940053219,29.147654687411,173.108250755187));
#90874=CARTESIAN_POINT('Origin',(-104.59506494869,26.6830679909832,152.608250755187));
#90875=CARTESIAN_POINT('',(-118.498906854159,17.798633272459,153.108250755187));
#90876=CARTESIAN_POINT('Origin',(-118.498906854159,17.798633272459,152.608250755187));
#90877=CARTESIAN_POINT('',(-113.6191566451,12.8694598796034,153.108250755187));
#90878=CARTESIAN_POINT('Origin',(-113.6191566451,12.8694598796034,152.608250755187));
#90879=CARTESIAN_POINT('Origin',(-104.59506494869,26.6830679909832,153.108250755187));
#90880=CARTESIAN_POINT('Ctrl Pts',(-112.492659345135,12.768040044578,153.608250755187));
#90881=CARTESIAN_POINT('Ctrl Pts',(-112.822059562284,12.9549939852504,153.608250755187));
#90882=CARTESIAN_POINT('Ctrl Pts',(-113.091226683409,12.6885257134127,153.608250755187));
#90883=CARTESIAN_POINT('Ctrl Pts',(-112.492659365801,12.7680400563074,153.475551801171));
#90884=CARTESIAN_POINT('Ctrl Pts',(-112.822059577098,12.9549939942945,153.527723751245));
#90885=CARTESIAN_POINT('Ctrl Pts',(-113.091226688129,12.6885257087402,153.541901279333));
#90886=CARTESIAN_POINT('Ctrl Pts',(-112.516334861812,12.7814084763901,153.342399703391));
#90887=CARTESIAN_POINT('Ctrl Pts',(-112.839359927912,12.9655349563554,153.446619353193));
#90888=CARTESIAN_POINT('Ctrl Pts',(-113.106153348276,12.6927270912805,153.475325227732));
#90889=CARTESIAN_POINT('Ctrl Pts',(-112.605696122325,12.8327090607538,153.098820706789));
#90890=CARTESIAN_POINT('Ctrl Pts',(-112.901940477622,13.0041108087007,153.3049590945));
#90891=CARTESIAN_POINT('Ctrl Pts',(-113.162275598232,12.7092343374356,153.353535732545));
#90892=CARTESIAN_POINT('Ctrl Pts',(-112.671479080234,12.8707492134964,152.987832794727));
#90893=CARTESIAN_POINT('Ctrl Pts',(-112.947776152446,13.0325418769711,153.243730625338));
#90894=CARTESIAN_POINT('Ctrl Pts',(-113.203518775813,12.7215983775457,153.298041773782));
#90895=CARTESIAN_POINT('Ctrl Pts',(-112.831184588058,12.9653805575584,152.805062971567));
#90896=CARTESIAN_POINT('Ctrl Pts',(-113.052608043631,13.0985506777719,153.152596157915));
#90897=CARTESIAN_POINT('Ctrl Pts',(-113.303060007586,12.7533719782569,153.206656864552));
#90898=CARTESIAN_POINT('Ctrl Pts',(-112.926443852807,13.0228217613013,152.731827736181));
#90899=CARTESIAN_POINT('Ctrl Pts',(-113.112910695034,13.1369984402749,153.1222986856));
#90900=CARTESIAN_POINT('Ctrl Pts',(-113.362176267773,12.7730921439476,153.170039246316));
#90901=CARTESIAN_POINT('Ctrl Pts',(-113.128994775364,13.148436735832,152.633922888492));
#90902=CARTESIAN_POINT('Ctrl Pts',(-113.232021149333,13.2138353374614,153.093277185672));
#90903=CARTESIAN_POINT('Ctrl Pts',(-113.486979497549,12.8177036267268,153.121086821207));
#90904=CARTESIAN_POINT('Ctrl Pts',(-113.239014126514,13.2183592414292,152.608250765972));
#90905=CARTESIAN_POINT('Ctrl Pts',(-113.29241434542,13.2532442939391,153.094953472492));
#90906=CARTESIAN_POINT('Ctrl Pts',(-113.554344147068,12.8432444717975,153.108250755187));
#90907=CARTESIAN_POINT('Ctrl Pts',(-113.345699320966,13.2880540647967,152.608250755187));
#90908=CARTESIAN_POINT('Ctrl Pts',(-113.345699320966,13.2880540647967,153.108250755187));
#90909=CARTESIAN_POINT('Ctrl Pts',(-113.6191566451,12.8694598796034,153.108250755187));
#90910=CARTESIAN_POINT('',(-113.091226683409,12.6885257134127,153.608250755187));
#90911=CARTESIAN_POINT('Origin',(-112.739459170024,12.3331954212528,153.608250755187));
#90912=CARTESIAN_POINT('Ctrl Pts',(-113.091226683409,12.6885257134127,153.608250755187));
#90913=CARTESIAN_POINT('Ctrl Pts',(-113.091226683409,12.6885257134127,153.585611929932));
#90914=CARTESIAN_POINT('Ctrl Pts',(-113.092960430494,12.6890138059481,153.563154237047));
#90915=CARTESIAN_POINT('Ctrl Pts',(-113.09628646338,12.6899636529493,153.541035429088));
#90916=CARTESIAN_POINT('Ctrl Pts',(-113.099770453205,12.6909586092235,153.517866174747));
#90917=CARTESIAN_POINT('Ctrl Pts',(-113.105001589543,12.6924601686088,153.495067766241));
#90918=CARTESIAN_POINT('Ctrl Pts',(-113.111870161412,12.694452165301,153.472807844599));
#90919=CARTESIAN_POINT('Ctrl Pts',(-113.113482515834,12.6949197741047,153.46758246678));
#90920=CARTESIAN_POINT('Ctrl Pts',(-113.115185319101,12.6954144688678,153.46238674342));
#90921=CARTESIAN_POINT('Ctrl Pts',(-113.116977544593,12.6959361508752,153.457222835554));
#90922=CARTESIAN_POINT('Ctrl Pts',(-113.122025717801,12.6974055759806,153.442677622656));
#90923=CARTESIAN_POINT('Ctrl Pts',(-113.127783397885,12.699089141154,153.428386396435));
#90924=CARTESIAN_POINT('Ctrl Pts',(-113.134214473254,12.700980714358,153.414430480138));
#90925=CARTESIAN_POINT('Ctrl Pts',(-113.136799123432,12.7017409379188,153.408821595238));
#90926=CARTESIAN_POINT('Ctrl Pts',(-113.139492892329,12.7025352357299,153.40326444683));
#90927=CARTESIAN_POINT('Ctrl Pts',(-113.142291009211,12.7033627973938,153.397762970209));
#90928=CARTESIAN_POINT('Ctrl Pts',(-113.156528687181,12.7075736852766,153.369769767705));
#90929=CARTESIAN_POINT('Ctrl Pts',(-113.173460893617,12.7126442230616,153.343230009338));
#90930=CARTESIAN_POINT('Ctrl Pts',(-113.192511133445,12.7184791208881,153.31853788334));
#90931=CARTESIAN_POINT('Ctrl Pts',(-113.210950781288,12.7241270004995,153.294637181197));
#90932=CARTESIAN_POINT('Ctrl Pts',(-113.231374818344,12.7304910090131,153.272467520468));
#90933=CARTESIAN_POINT('Ctrl Pts',(-113.253288174875,12.7374867495037,153.252349061816));
#90934=CARTESIAN_POINT('Ctrl Pts',(-113.255294838239,12.738127367755,153.250506761946));
#90935=CARTESIAN_POINT('Ctrl Pts',(-113.257315340498,12.7387737898784,153.248680454799));
#90936=CARTESIAN_POINT('Ctrl Pts',(-113.259349216641,12.7394259068857,153.246870287867));
#90937=CARTESIAN_POINT('Ctrl Pts',(-113.278039033598,12.745418379705,153.230236193036));
#90938=CARTESIAN_POINT('Ctrl Pts',(-113.29783448671,12.7518833303128,153.21498126598));
#90939=CARTESIAN_POINT('Ctrl Pts',(-113.318454814089,12.7587610622854,153.201166192586));
#90940=CARTESIAN_POINT('Ctrl Pts',(-113.340312817521,12.766051610408,153.186521909005));
#90941=CARTESIAN_POINT('Ctrl Pts',(-113.363098774174,12.7738061414787,153.173494523177));
#90942=CARTESIAN_POINT('Ctrl Pts',(-113.386524441212,12.7819706583693,153.162187747809));
#90943=CARTESIAN_POINT('Ctrl Pts',(-113.399038703457,12.7863322377132,153.156147537647));
#90944=CARTESIAN_POINT('Ctrl Pts',(-113.411736190924,12.7908110879754,153.150598972778));
#90945=CARTESIAN_POINT('Ctrl Pts',(-113.424576119712,12.7954005301353,153.145562771898));
#90946=CARTESIAN_POINT('Ctrl Pts',(-113.448763789768,12.8040460541511,153.13607565034));
#90947=CARTESIAN_POINT('Ctrl Pts',(-113.473708893912,12.8131811825802,153.128328353013));
#90948=CARTESIAN_POINT('Ctrl Pts',(-113.499063291583,12.8226927418264,153.122388238271));
#90949=CARTESIAN_POINT('Ctrl Pts',(-113.522652974056,12.8315422781222,153.116861567024));
#90950=CARTESIAN_POINT('Ctrl Pts',(-113.546598429537,12.8407182262617,153.112899483273));
#90951=CARTESIAN_POINT('Ctrl Pts',(-113.570610123686,12.8501313371616,153.110597998102));
#90952=CARTESIAN_POINT('Ctrl Pts',(-113.586794432208,12.8564759411706,153.109046756201));
#90953=CARTESIAN_POINT('Ctrl Pts',(-113.60300863266,12.8629283194227,153.108250755187));
#90954=CARTESIAN_POINT('Ctrl Pts',(-113.6191566451,12.8694598796034,153.108250755187));
#90955=CARTESIAN_POINT('Ctrl Pts',(-118.077578311569,18.0678585669597,152.608250755187));
#90956=CARTESIAN_POINT('Ctrl Pts',(-118.077578311569,18.0678585669597,153.108250755187));
#90957=CARTESIAN_POINT('Ctrl Pts',(-118.498906854159,17.798633272459,153.108250755187));
#90958=CARTESIAN_POINT('Ctrl Pts',(-118.147030774962,18.1765493392544,152.60825077749));
#90959=CARTESIAN_POINT('Ctrl Pts',(-118.112276872432,18.1221606460463,153.094787604524));
#90960=CARTESIAN_POINT('Ctrl Pts',(-118.524781217919,17.8645045048263,153.108250755187));
#90961=CARTESIAN_POINT('Ctrl Pts',(-118.214837800552,18.2856761107436,152.633710236017));
#90962=CARTESIAN_POINT('Ctrl Pts',(-118.150528898799,18.1820886305035,153.093185957657));
#90963=CARTESIAN_POINT('Ctrl Pts',(-118.54927185006,17.9311502346664,153.120980492262));
#90964=CARTESIAN_POINT('Ctrl Pts',(-118.339271941506,18.4909268139004,152.732462696752));
#90965=CARTESIAN_POINT('Ctrl Pts',(-118.226709857927,18.3028399523544,153.122507989483));
#90966=CARTESIAN_POINT('Ctrl Pts',(-118.592923646367,18.0572865403011,153.170356729309));
#90967=CARTESIAN_POINT('Ctrl Pts',(-118.395262004592,18.5859573989267,152.805334639289));
#90968=CARTESIAN_POINT('Ctrl Pts',(-118.264258537582,18.3630692431351,153.152707467856));
#90969=CARTESIAN_POINT('Ctrl Pts',(-118.611875090787,18.1161056718008,153.206792695945));
#90970=CARTESIAN_POINT('Ctrl Pts',(-118.488400449801,18.7468303826905,152.988630571688));
#90971=CARTESIAN_POINT('Ctrl Pts',(-118.329305263756,18.4687247489854,153.244147548454));
#90972=CARTESIAN_POINT('Ctrl Pts',(-118.642680868104,18.216101888196,153.298440664731));
#90973=CARTESIAN_POINT('Ctrl Pts',(-118.525706546847,18.8128807906123,153.099898214101));
#90974=CARTESIAN_POINT('Ctrl Pts',(-118.357233870597,18.5147847472074,153.30558183398));
#90975=CARTESIAN_POINT('Ctrl Pts',(-118.654603964361,18.2573986678045,153.354074484501));
#90976=CARTESIAN_POINT('Ctrl Pts',(-118.575794350635,18.902205102153,153.342371533405));
#90977=CARTESIAN_POINT('Ctrl Pts',(-118.394946624077,18.5773697525724,153.446616730793));
#90978=CARTESIAN_POINT('Ctrl Pts',(-118.670446123243,18.3133407705919,153.475311144438));
#90979=CARTESIAN_POINT('Ctrl Pts',(-118.588969901031,18.9260953737285,153.475893601961));
#90980=CARTESIAN_POINT('Ctrl Pts',(-118.405344796735,18.5948279601087,153.527930080756));
#90981=CARTESIAN_POINT('Ctrl Pts',(-118.674511919973,18.3283596898625,153.542072178464));
#90982=CARTESIAN_POINT('Ctrl Pts',(-118.588969902809,18.9260953769367,153.608250755187));
#90983=CARTESIAN_POINT('Ctrl Pts',(-118.405344798115,18.5948279624256,153.608250755187));
#90984=CARTESIAN_POINT('Ctrl Pts',(-118.67451191924,18.3283596905879,153.608250755187));
#90985=CARTESIAN_POINT('',(-118.67451191924,18.3283596905879,153.608250755187));
#90986=CARTESIAN_POINT('Origin',(-119.026279432626,18.6836899827478,153.608250755187));
#90987=CARTESIAN_POINT('Ctrl Pts',(-118.498906854159,17.798633272459,153.108250755187));
#90988=CARTESIAN_POINT('Ctrl Pts',(-118.509426949702,17.825415444359,153.108250755187));
#90989=CARTESIAN_POINT('Ctrl Pts',(-118.519653630627,17.852159341054,153.110350857061));
#90990=CARTESIAN_POINT('Ctrl Pts',(-118.529539029884,17.8786538141036,153.114447252937));
#90991=CARTESIAN_POINT('Ctrl Pts',(-118.53968600027,17.9058493401947,153.118652040884));
#90992=CARTESIAN_POINT('Ctrl Pts',(-118.549473755328,17.9327832401008,153.124960207408));
#90993=CARTESIAN_POINT('Ctrl Pts',(-118.558846330244,17.9592354635942,153.13331284971));
#90994=CARTESIAN_POINT('Ctrl Pts',(-118.56301414395,17.9709982865785,153.137027117921));
#90995=CARTESIAN_POINT('Ctrl Pts',(-118.567099770752,17.9826658616096,153.141146354449));
#90996=CARTESIAN_POINT('Ctrl Pts',(-118.571097735592,17.994218395715,153.145668609543));
#90997=CARTESIAN_POINT('Ctrl Pts',(-118.579993608979,18.0199239446165,153.155731081412));
#90998=CARTESIAN_POINT('Ctrl Pts',(-118.588421530591,18.0449504539258,153.167751327949));
#90999=CARTESIAN_POINT('Ctrl Pts',(-118.596353258894,18.0690479409552,153.181631702461));
#91000=CARTESIAN_POINT('Ctrl Pts',(-118.603926897438,18.0920575108272,153.19488542667));
#91001=CARTESIAN_POINT('Ctrl Pts',(-118.611048207261,18.1142208889254,153.209835861402));
#91002=CARTESIAN_POINT('Ctrl Pts',(-118.617680017612,18.1352871692305,153.226428438647));
#91003=CARTESIAN_POINT('Ctrl Pts',(-118.620269444893,18.1435126156807,153.232907102825));
#91004=CARTESIAN_POINT('Ctrl Pts',(-118.622784099424,18.151570367692,153.239636401772));
#91005=CARTESIAN_POINT('Ctrl Pts',(-118.625221173516,18.1594436001056,153.246614074428));
#91006=CARTESIAN_POINT('Ctrl Pts',(-118.625913224327,18.1616793453773,153.248595509476));
#91007=CARTESIAN_POINT('Ctrl Pts',(-118.62659882118,18.1638995706237,153.250596415344));
#91008=CARTESIAN_POINT('Ctrl Pts',(-118.627277889784,18.1661038480104,153.252616665764));
#91009=CARTESIAN_POINT('Ctrl Pts',(-118.634279897975,18.1888325800265,153.273447860005));
#91010=CARTESIAN_POINT('Ctrl Pts',(-118.640602769921,18.2098942489168,153.296424536251));
#91011=CARTESIAN_POINT('Ctrl Pts',(-118.646174902136,18.2287912078352,153.321170461487));
#91012=CARTESIAN_POINT('Ctrl Pts',(-118.65144886848,18.2466769868291,153.344592227479));
#91013=CARTESIAN_POINT('Ctrl Pts',(-118.656050279007,18.2626236397145,153.369599261712));
#91014=CARTESIAN_POINT('Ctrl Pts',(-118.65991044876,18.2761669413062,153.395852653189));
#91015=CARTESIAN_POINT('Ctrl Pts',(-118.660823821723,18.2793714857411,153.402064591909));
#91016=CARTESIAN_POINT('Ctrl Pts',(-118.661695658719,18.2824412753062,153.408346207006));
#91017=CARTESIAN_POINT('Ctrl Pts',(-118.662524980496,18.2853697768892,153.414692806039));
#91018=CARTESIAN_POINT('Ctrl Pts',(-118.665946421777,18.2974515725156,153.4408762689));
#91019=CARTESIAN_POINT('Ctrl Pts',(-118.668672076308,18.3072005590298,153.468385102507));
#91020=CARTESIAN_POINT('Ctrl Pts',(-118.670655418809,18.3143466012114,153.496722756828));
#91021=CARTESIAN_POINT('Ctrl Pts',(-118.672547533301,18.3211639461522,153.523756961136));
#91022=CARTESIAN_POINT('Ctrl Pts',(-118.673764036787,18.3256122792076,153.551545730234));
#91023=CARTESIAN_POINT('Ctrl Pts',(-118.674259156222,18.3274298612428,153.579619100731));
#91024=CARTESIAN_POINT('Ctrl Pts',(-118.674427021917,18.3280460957345,153.589137119098));
#91025=CARTESIAN_POINT('Ctrl Pts',(-118.67451191924,18.3283596905879,153.59868749477));
#91026=CARTESIAN_POINT('Ctrl Pts',(-118.67451191924,18.3283596905879,153.608250755187));
#91027=CARTESIAN_POINT('Origin',(-112.739459170024,12.3331954212528,171.608250755187));
#91028=CARTESIAN_POINT('',(-113.091226683409,12.6885257134127,171.108250755187));
#91029=CARTESIAN_POINT('Origin',(-112.739459170024,12.3331954212528,171.108250755187));
#91030=CARTESIAN_POINT('',(-113.091226683409,12.6885257134127,153.108250755187));
#91031=CARTESIAN_POINT('Origin',(-102.15518984416,24.2184812945555,153.608250755187));
#91032=CARTESIAN_POINT('',(-123.121472352097,2.75884998530158,153.608250755187));
#91033=CARTESIAN_POINT('',(-123.473239865483,3.11418027746143,153.108250755187));
#91034=CARTESIAN_POINT('Origin',(-123.473239865483,3.11418027746144,153.608250755187));
#91035=CARTESIAN_POINT('',(-123.473239865483,3.11418027746143,153.108250755187));
#91036=CARTESIAN_POINT('',(-112.818771417413,12.9582491609851,153.608250755187));
#91037=CARTESIAN_POINT('Origin',(-107.034940053219,29.147654687411,153.608250755187));
#91038=CARTESIAN_POINT('',(-128.352990074541,8.04335367031699,153.108250755187));
#91039=CARTESIAN_POINT('',(-128.704757587927,8.39868396247684,153.608250755187));
#91040=CARTESIAN_POINT('Origin',(-128.352990074541,8.04335367031699,153.608250755187));
#91041=CARTESIAN_POINT('',(-128.704757587927,8.39868396247683,153.608250755187));
#91042=CARTESIAN_POINT('',(-118.050289139858,18.2427528460005,153.108250755187));
#91043=CARTESIAN_POINT('Origin',(-119.026279432626,18.6836899827478,171.608250755187));
#91044=CARTESIAN_POINT('',(-118.67451191924,18.3283596905879,171.108250755187));
#91045=CARTESIAN_POINT('Origin',(-119.026279432626,18.6836899827478,171.108250755187));
#91046=CARTESIAN_POINT('',(-118.67451191924,18.3283596905879,153.108250755187));
#91047=CARTESIAN_POINT('Ctrl Pts',(-113.091226683409,12.6885257134127,171.108250755187));
#91048=CARTESIAN_POINT('Ctrl Pts',(-112.822059562284,12.9549939852504,171.108250755187));
#91049=CARTESIAN_POINT('Ctrl Pts',(-112.492659345135,12.768040044578,171.108250755187));
#91050=CARTESIAN_POINT('Ctrl Pts',(-113.091226665924,12.6885257307224,171.241737242521));
#91051=CARTESIAN_POINT('Ctrl Pts',(-112.822059549918,12.9549939974928,171.189238482124));
#91052=CARTESIAN_POINT('Ctrl Pts',(-112.492659339517,12.7680400413896,171.174993997723));
#91053=CARTESIAN_POINT('Ctrl Pts',(-113.071044170768,12.7085058627058,171.375809742194));
#91054=CARTESIAN_POINT('Ctrl Pts',(-112.807577395421,12.9693309442375,171.270872142593));
#91055=CARTESIAN_POINT('Ctrl Pts',(-112.479441467766,12.7762529890477,171.242030250224));
#91056=CARTESIAN_POINT('Ctrl Pts',(-112.994537385668,12.7842455396925,171.620480252948));
#91057=CARTESIAN_POINT('Ctrl Pts',(-112.754163654268,13.0222091235583,171.414405744629));
#91058=CARTESIAN_POINT('Ctrl Pts',(-112.429155434994,12.8073151622197,171.364365502534));
#91059=CARTESIAN_POINT('Ctrl Pts',(-112.938043914811,12.8401725692882,171.731805299994));
#91060=CARTESIAN_POINT('Ctrl Pts',(-112.714674682077,13.0613021529447,171.477100056791));
#91061=CARTESIAN_POINT('Ctrl Pts',(-112.391965914469,12.8302288792103,171.420028028857));
#91062=CARTESIAN_POINT('Ctrl Pts',(-112.800186397533,12.9766478350468,171.914243767979));
#91063=CARTESIAN_POINT('Ctrl Pts',(-112.62212411815,13.1529247431191,171.570720798637));
#91064=CARTESIAN_POINT('Ctrl Pts',(-112.300709976456,12.8859483002505,171.511247260317));
#91065=CARTESIAN_POINT('Ctrl Pts',(-112.717686219217,13.0583208114866,171.986819299416));
#91066=CARTESIAN_POINT('Ctrl Pts',(-112.567712576532,13.2067907182878,171.602133212335));
#91067=CARTESIAN_POINT('Ctrl Pts',(-112.245878978066,12.9192082849092,171.547535027057));
#91068=CARTESIAN_POINT('Ctrl Pts',(-112.541234736795,13.2330030735238,172.083342412463));
#91069=CARTESIAN_POINT('Ctrl Pts',(-112.458003469363,13.3153998086934,171.630196458045));
#91070=CARTESIAN_POINT('Ctrl Pts',(-112.127800287923,12.9900408536816,171.595796584069));
#91071=CARTESIAN_POINT('Ctrl Pts',(-112.445088038195,13.3281857411239,172.108250746497));
#91072=CARTESIAN_POINT('Ctrl Pts',(-112.401068533116,13.3717638772499,171.626173327527));
#91073=CARTESIAN_POINT('Ctrl Pts',(-112.063076145661,13.0284859943151,171.608250755187));
#91074=CARTESIAN_POINT('Ctrl Pts',(-112.351090138778,13.4212411548363,172.108250755187));
#91075=CARTESIAN_POINT('Ctrl Pts',(-112.351090138778,13.4212411548362,171.608250755187));
#91076=CARTESIAN_POINT('Ctrl Pts',(-111.999322625392,13.0659108626764,171.608250755187));
#91077=CARTESIAN_POINT('',(-112.351090138778,13.4212411548362,172.108250755187));
#91078=CARTESIAN_POINT('Origin',(-111.999322625392,13.0659108626764,172.108250755187));
#91079=CARTESIAN_POINT('Ctrl Pts',(-112.351090138778,13.4212411548362,172.108250755187));
#91080=CARTESIAN_POINT('Ctrl Pts',(-112.37788022512,13.3947196837876,172.10825075271));
#91081=CARTESIAN_POINT('Ctrl Pts',(-112.40463333433,13.3682348191149,172.106231383603));
#91082=CARTESIAN_POINT('Ctrl Pts',(-112.431196342464,13.3419381494371,172.102298699115));
#91083=CARTESIAN_POINT('Ctrl Pts',(-112.458539312306,13.3148693384673,172.098250540382));
#91084=CARTESIAN_POINT('Ctrl Pts',(-112.485681781686,13.2879990176084,172.092175073619));
#91085=CARTESIAN_POINT('Ctrl Pts',(-112.51247019042,13.261479207346,172.084134831724));
#91086=CARTESIAN_POINT('Ctrl Pts',(-112.539286838453,13.2349314409313,172.076086114119));
#91087=CARTESIAN_POINT('Ctrl Pts',(-112.56574968046,13.2087339330476,172.066068297258));
#91088=CARTESIAN_POINT('Ctrl Pts',(-112.5917032287,13.1830406124129,172.054093236393));
#91089=CARTESIAN_POINT('Ctrl Pts',(-112.604417695173,13.1704536296702,172.048226735655));
#91090=CARTESIAN_POINT('Ctrl Pts',(-112.617009817885,13.1579877639894,172.041889749809));
#91091=CARTESIAN_POINT('Ctrl Pts',(-112.629460076087,13.1456623403912,172.035079401128));
#91092=CARTESIAN_POINT('Ctrl Pts',(-112.629684331028,13.1454403339799,172.034956732641));
#91093=CARTESIAN_POINT('Ctrl Pts',(-112.629908554095,13.1452183591231,172.034833904296));
#91094=CARTESIAN_POINT('Ctrl Pts',(-112.630132745208,13.1449964158994,172.034710916136));
#91095=CARTESIAN_POINT('Ctrl Pts',(-112.718097704872,13.0579134516647,171.98645454965));
#91096=CARTESIAN_POINT('Ctrl Pts',(-112.800361629498,12.9764743600703,171.914009179875));
#91097=CARTESIAN_POINT('Ctrl Pts',(-112.869114678965,12.908410674588,171.823023819991));
#91098=CARTESIAN_POINT('Ctrl Pts',(-112.869231489841,12.9082950349356,171.822869236599));
#91099=CARTESIAN_POINT('Ctrl Pts',(-112.869348264987,12.9081794306553,171.822714595501));
#91100=CARTESIAN_POINT('Ctrl Pts',(-112.869465004375,12.9080638617748,171.822559896743));
#91101=CARTESIAN_POINT('Ctrl Pts',(-112.938234347511,12.8399840459954,171.731429283186));
#91102=CARTESIAN_POINT('Ctrl Pts',(-112.994600553214,12.7841830055055,171.620275542505));
#91103=CARTESIAN_POINT('Ctrl Pts',(-113.03279042474,12.7463760511326,171.498144778716));
#91104=CARTESIAN_POINT('Ctrl Pts',(-113.032822838721,12.7463439621563,171.498041119184));
#91105=CARTESIAN_POINT('Ctrl Pts',(-113.032855239728,12.7463118860227,171.497937451222));
#91106=CARTESIAN_POINT('Ctrl Pts',(-113.032887627762,12.7462798227332,171.497833774838));
#91107=CARTESIAN_POINT('Ctrl Pts',(-113.043934868349,12.735343349157,171.462470776879));
#91108=CARTESIAN_POINT('Ctrl Pts',(-113.053439241226,12.7259342734692,171.426245512342));
#91109=CARTESIAN_POINT('Ctrl Pts',(-113.061393897703,12.7180593756897,171.389360653078));
#91110=CARTESIAN_POINT('Ctrl Pts',(-113.069355830694,12.7101772743547,171.352442053422));
#91111=CARTESIAN_POINT('Ctrl Pts',(-113.075765402173,12.7038319695192,171.314861536721));
#91112=CARTESIAN_POINT('Ctrl Pts',(-113.080580816924,12.6990648373324,171.276805373265));
#91113=CARTESIAN_POINT('Ctrl Pts',(-113.08526166173,12.694430925802,171.239812714423));
#91114=CARTESIAN_POINT('Ctrl Pts',(-113.088436240631,12.6912881773485,171.202369605244));
#91115=CARTESIAN_POINT('Ctrl Pts',(-113.090031776628,12.6897086392607,171.164646810892));
#91116=CARTESIAN_POINT('Ctrl Pts',(-113.090824288283,12.6889240738568,171.145909687922));
#91117=CARTESIAN_POINT('Ctrl Pts',(-113.09122668094,12.6885257158574,171.127103649708));
#91118=CARTESIAN_POINT('Ctrl Pts',(-113.091226683409,12.6885257134127,171.108250755187));
#91119=CARTESIAN_POINT('Origin',(-125.913114970012,5.57876697388921,153.608250755187));
#91120=CARTESIAN_POINT('Origin',(-125.913114970012,5.57876697388921,153.608250755187));
#91121=CARTESIAN_POINT('Origin',(-125.913114970012,5.57876697388921,153.108250755187));
#91122=CARTESIAN_POINT('Ctrl Pts',(-117.934375374608,19.0610751320115,172.108250755187));
#91123=CARTESIAN_POINT('Ctrl Pts',(-117.934375374608,19.0610751320115,171.608250755187));
#91124=CARTESIAN_POINT('Ctrl Pts',(-118.286142887994,19.4164054241713,171.608250755187));
#91125=CARTESIAN_POINT('Ctrl Pts',(-118.029559849224,18.9668450404955,172.108250736963));
#91126=CARTESIAN_POINT('Ctrl Pts',(-117.984985945151,19.0109720168266,171.626400023775));
#91127=CARTESIAN_POINT('Ctrl Pts',(-118.324686897321,19.3522354702217,171.608250755187));
#91128=CARTESIAN_POINT('Ctrl Pts',(-118.124181115612,18.873172510106,172.083590099036));
#91129=CARTESIAN_POINT('Ctrl Pts',(-118.0410594303,18.9554607618992,171.630295894894));
#91130=CARTESIAN_POINT('Ctrl Pts',(-118.363165092524,19.2889233489514,171.595920429989));
#91131=CARTESIAN_POINT('Ctrl Pts',(-118.301922666664,18.6972131145286,171.986236425372));
#91132=CARTESIAN_POINT('Ctrl Pts',(-118.151583977807,18.846044407303,171.601943545762));
#91133=CARTESIAN_POINT('Ctrl Pts',(-118.43571109596,19.1707080971491,171.547243587402));
#91134=CARTESIAN_POINT('Ctrl Pts',(-118.383568279172,18.6163861354481,171.914220536541));
#91135=CARTESIAN_POINT('Ctrl Pts',(-118.205467625802,18.7927010327455,171.570727890218));
#91136=CARTESIAN_POINT('Ctrl Pts',(-118.469172851448,19.1167826550558,171.511235647295));
#91137=CARTESIAN_POINT('Ctrl Pts',(-118.521836709987,18.4795040762472,171.73102847759));
#91138=CARTESIAN_POINT('Ctrl Pts',(-118.29830160884,18.7007978652077,171.476689446383));
#91139=CARTESIAN_POINT('Ctrl Pts',(-118.525978293722,19.0258237386759,171.419639614957));
#91140=CARTESIAN_POINT('Ctrl Pts',(-118.578135214163,18.4237700584662,171.619640310305));
#91141=CARTESIAN_POINT('Ctrl Pts',(-118.337667677041,18.6618265074946,171.413915961975));
#91142=CARTESIAN_POINT('Ctrl Pts',(-118.549185781588,18.988995972916,171.363945533082));
#91143=CARTESIAN_POINT('Ctrl Pts',(-118.654287937188,18.3483808934916,171.37578205691));
#91144=CARTESIAN_POINT('Ctrl Pts',(-118.390835760335,18.6091915229033,171.270846895345));
#91145=CARTESIAN_POINT('Ctrl Pts',(-118.580607120652,18.9392570552061,171.242016405712));
#91146=CARTESIAN_POINT('Ctrl Pts',(-118.674511917534,18.3283596922771,171.241710900386));
#91147=CARTESIAN_POINT('Ctrl Pts',(-118.405344796902,18.5948279636271,171.189221495563));
#91148=CARTESIAN_POINT('Ctrl Pts',(-118.588969903115,18.926095377489,171.17498082804));
#91149=CARTESIAN_POINT('Ctrl Pts',(-118.67451191924,18.3283596905879,171.108250755187));
#91150=CARTESIAN_POINT('Ctrl Pts',(-118.405344798115,18.5948279624256,171.108250755187));
#91151=CARTESIAN_POINT('Ctrl Pts',(-118.588969902809,18.9260953769367,171.108250755187));
#91152=CARTESIAN_POINT('',(-117.934375374608,19.0610751320115,172.108250755187));
#91153=CARTESIAN_POINT('Origin',(-118.286142887994,19.4164054241713,172.108250755187));
#91154=CARTESIAN_POINT('Ctrl Pts',(-118.67451191924,18.3283596905879,171.108250755187));
#91155=CARTESIAN_POINT('Ctrl Pts',(-118.674511918748,18.3283596910749,171.146726782688));
#91156=CARTESIAN_POINT('Ctrl Pts',(-118.672803575978,18.3300508975469,171.185041427643));
#91157=CARTESIAN_POINT('Ctrl Pts',(-118.669481657713,18.3333395380046,171.222986490301));
#91158=CARTESIAN_POINT('Ctrl Pts',(-118.667807717348,18.3349967094246,171.242107301523));
#91159=CARTESIAN_POINT('Ctrl Pts',(-118.665723460677,18.3370600938892,171.261134517818));
#91160=CARTESIAN_POINT('Ctrl Pts',(-118.663237553743,18.3395211258692,171.280042307355));
#91161=CARTESIAN_POINT('Ctrl Pts',(-118.658108554535,18.3445988023115,171.31905343695));
#91162=CARTESIAN_POINT('Ctrl Pts',(-118.651274179188,18.3513648861267,171.357556066268));
#91163=CARTESIAN_POINT('Ctrl Pts',(-118.642836006864,18.3597187358104,171.395315415702));
#91164=CARTESIAN_POINT('Ctrl Pts',(-118.640090020348,18.3624372816882,171.407603226428));
#91165=CARTESIAN_POINT('Ctrl Pts',(-118.637173929813,18.365324228441,171.419812520377));
#91166=CARTESIAN_POINT('Ctrl Pts',(-118.634090461384,18.3683768672509,171.431935680483));
#91167=CARTESIAN_POINT('Ctrl Pts',(-118.629380951638,18.3730392896352,171.450451887793));
#91168=CARTESIAN_POINT('Ctrl Pts',(-118.624282129381,18.3780870998679,171.46876644342));
#91169=CARTESIAN_POINT('Ctrl Pts',(-118.618805779133,18.3835085796861,171.486850966306));
#91170=CARTESIAN_POINT('Ctrl Pts',(-118.61774609186,18.3845576493959,171.490350366066));
#91171=CARTESIAN_POINT('Ctrl Pts',(-118.616672245082,18.3856207337022,171.493841420748));
#91172=CARTESIAN_POINT('Ctrl Pts',(-118.615584463112,18.3866976107387,171.497323013247));
#91173=CARTESIAN_POINT('Ctrl Pts',(-118.614212821057,18.3880555021842,171.501713138128));
#91174=CARTESIAN_POINT('Ctrl Pts',(-118.612818540126,18.3894358011566,171.506090294806));
#91175=CARTESIAN_POINT('Ctrl Pts',(-118.611402274461,18.3908378605866,171.510452436845));
#91176=CARTESIAN_POINT('Ctrl Pts',(-118.59832989421,18.403779114795,171.550715772199));
#91177=CARTESIAN_POINT('Ctrl Pts',(-118.583368635811,18.4185899911859,171.589744502641));
#91178=CARTESIAN_POINT('Ctrl Pts',(-118.566654225325,18.4351365211238,171.62722631931));
#91179=CARTESIAN_POINT('Ctrl Pts',(-118.559016615326,18.4426974185068,171.644353546023));
#91180=CARTESIAN_POINT('Ctrl Pts',(-118.551012854864,18.4506208105775,171.661157055623));
#91181=CARTESIAN_POINT('Ctrl Pts',(-118.542655786931,18.4588939974157,171.677603438498));
#91182=CARTESIAN_POINT('Ctrl Pts',(-118.52426226963,18.4771028963319,171.713801161233));
#91183=CARTESIAN_POINT('Ctrl Pts',(-118.504156769756,18.4970067592832,171.748272860833));
#91184=CARTESIAN_POINT('Ctrl Pts',(-118.482478354792,18.5184678018624,171.780699583238));
#91185=CARTESIAN_POINT('Ctrl Pts',(-118.472859081881,18.527990621028,171.795088157906));
#91186=CARTESIAN_POINT('Ctrl Pts',(-118.462929929778,18.5378202177442,171.809073466704));
#91187=CARTESIAN_POINT('Ctrl Pts',(-118.452702447228,18.5479451527244,171.8226244363));
#91188=CARTESIAN_POINT('Ctrl Pts',(-118.452588703835,18.5480577556501,171.822775141349));
#91189=CARTESIAN_POINT('Ctrl Pts',(-118.452474924419,18.5481703942374,171.822925793229));
#91190=CARTESIAN_POINT('Ctrl Pts',(-118.452361108996,18.5482830684709,171.82307639192));
#91191=CARTESIAN_POINT('Ctrl Pts',(-118.391062933909,18.6089666271241,171.904185126661));
#91192=CARTESIAN_POINT('Ctrl Pts',(-118.319961202882,18.6793554447188,171.969901908819));
#91193=CARTESIAN_POINT('Ctrl Pts',(-118.242712238982,18.7558298589259,172.017635952979));
#91194=CARTESIAN_POINT('Ctrl Pts',(-118.23292174852,18.7655221833933,172.023685739028));
#91195=CARTESIAN_POINT('Ctrl Pts',(-118.223032489557,18.7753122860422,172.029446612682));
#91196=CARTESIAN_POINT('Ctrl Pts',(-118.213051886797,18.7851928166143,172.034913246513));
#91197=CARTESIAN_POINT('Ctrl Pts',(-118.212978778006,18.785265192368,172.034953290086));
#91198=CARTESIAN_POINT('Ctrl Pts',(-118.212905665311,18.7853375719858,172.034993317412));
#91199=CARTESIAN_POINT('Ctrl Pts',(-118.212832548717,18.7854099554649,172.035033328492));
#91200=CARTESIAN_POINT('Ctrl Pts',(-118.183575689157,18.8143734662143,172.051043353842));
#91201=CARTESIAN_POINT('Ctrl Pts',(-118.153768792948,18.843881498579,172.064416117585));
#91202=CARTESIAN_POINT('Ctrl Pts',(-118.12352859055,18.8738184925162,172.07518031916));
#91203=CARTESIAN_POINT('Ctrl Pts',(-118.092750083519,18.9042883936841,172.086136133856));
#91204=CARTESIAN_POINT('Ctrl Pts',(-118.06152210619,18.9352032584602,172.094389922825));
#91205=CARTESIAN_POINT('Ctrl Pts',(-118.029958765621,18.9664501239011,172.09991854538));
#91206=CARTESIAN_POINT('Ctrl Pts',(-117.998395425051,18.997696989342,172.105447167935));
#91207=CARTESIAN_POINT('Ctrl Pts',(-117.96649607465,19.0292764955558,172.108250749037));
#91208=CARTESIAN_POINT('Ctrl Pts',(-117.934375374608,19.0610751320115,172.108250755187));
#91209=CARTESIAN_POINT('Origin',(-101.451654817389,23.5078207102358,172.108250755187));
#91210=CARTESIAN_POINT('',(-101.803422330775,23.8631510023956,172.108250755187));
#91211=CARTESIAN_POINT('',(-112.467003904028,12.6029188688252,171.608250755187));
#91212=CARTESIAN_POINT('Origin',(-107.738475079991,29.8583152717307,172.108250755187));
#91213=CARTESIAN_POINT('',(-107.738475079991,29.8583152717307,171.608250755187));
#91214=CARTESIAN_POINT('',(-118.402056653244,18.5980831381603,172.108250755187));
#91215=CARTESIAN_POINT('Origin',(-104.59506494869,26.6830679909832,173.108250755187));
#91216=CARTESIAN_POINT('Origin',(-104.59506494869,26.6830679909832,153.108250755187));
#91217=CARTESIAN_POINT('Origin',(-125.913114970012,5.57876697388921,153.108250755187));
#91218=CARTESIAN_POINT('',(-128.704757587927,8.39868396247684,153.108250755187));
#91219=CARTESIAN_POINT('',(-123.121472352097,2.75884998530158,153.108250755187));
#91220=CARTESIAN_POINT('Origin',(-107.386707566605,29.5029849795709,153.108250755187));
#91221=CARTESIAN_POINT('Origin',(-101.803422330775,23.8631510023956,153.108250755187));
#91222=CARTESIAN_POINT('Origin',(-104.59506494869,26.6830679909832,171.608250755187));
#91223=CARTESIAN_POINT('Origin',(-104.59506494869,26.6830679909832,173.608250755187));
#91224=CARTESIAN_POINT('',(-205.7,24.8757620423259,173.608250755187));
#91225=CARTESIAN_POINT('Origin',(35.4049350513103,26.6830679909832,173.608250755187));
#91226=CARTESIAN_POINT('',(-205.7,24.8757620423259,173.608250755187));
#91227=CARTESIAN_POINT('Origin',(-34.5950649486897,26.6830679909832,173.608250755187));
#91228=CARTESIAN_POINT('',(-205.7,24.8757620423259,173.608250755187));
#91229=CARTESIAN_POINT('Origin',(190.,54.4,211.4));
#91230=CARTESIAN_POINT('',(190.5,54.4,41.));
#91231=CARTESIAN_POINT('Origin',(190.,54.4,41.));
#91232=CARTESIAN_POINT('',(190.5,54.4,102.225104347672));
#91233=CARTESIAN_POINT('Origin',(190.,54.4,102.225104347672));
#91234=CARTESIAN_POINT('',(190.5,54.4,211.4));
#91235=CARTESIAN_POINT('Origin',(160.5,54.4,102.225104347672));
#91236=CARTESIAN_POINT('',(190.499797482064,54.4,102.335336081499));
#91237=CARTESIAN_POINT('Origin',(189.999800857363,54.4,102.333498885935));
#91238=CARTESIAN_POINT('Origin',(160.5,54.4,102.225104347672));
#91239=CARTESIAN_POINT('Ctrl Pts',(189.5,54.85,40.282055052823));
#91240=CARTESIAN_POINT('Ctrl Pts',(190.217944947177,54.85,40.282055052823));
#91241=CARTESIAN_POINT('Ctrl Pts',(190.217944947177,54.85,41.));
#91242=CARTESIAN_POINT('Ctrl Pts',(189.5,54.7133945031366,40.));
#91243=CARTESIAN_POINT('Ctrl Pts',(190.5,54.7133945031366,40.));
#91244=CARTESIAN_POINT('Ctrl Pts',(190.5,54.7133945031366,41.));
#91245=CARTESIAN_POINT('Ctrl Pts',(189.5,54.4,40.));
#91246=CARTESIAN_POINT('Ctrl Pts',(190.5,54.4,40.));
#91247=CARTESIAN_POINT('Ctrl Pts',(190.5,54.4,41.));
#91248=CARTESIAN_POINT('',(189.5,54.4,40.));
#91249=CARTESIAN_POINT('Origin',(189.5,54.4,41.));
#91250=CARTESIAN_POINT('Origin',(189.5,54.4,40.5));
#91251=CARTESIAN_POINT('Ctrl Pts',(190.219194548401,54.8501814482227,101.816662400769));
#91252=CARTESIAN_POINT('Ctrl Pts',(190.501623088573,54.7136847329578,101.817606429853));
#91253=CARTESIAN_POINT('Ctrl Pts',(190.501623088584,54.4000000000002,101.817606429849));
#91254=CARTESIAN_POINT('Ctrl Pts',(190.200871934805,54.8501814482482,107.235732213123));
#91255=CARTESIAN_POINT('Ctrl Pts',(190.483296758343,54.7136847330045,107.23763909223));
#91256=CARTESIAN_POINT('Ctrl Pts',(190.483296758234,54.399999999995,107.23763909227));
#91257=CARTESIAN_POINT('Ctrl Pts',(190.158430844455,54.8501814482705,112.654414896875));
#91258=CARTESIAN_POINT('Ctrl Pts',(190.440853585033,54.713684733061,112.657855156237));
#91259=CARTESIAN_POINT('Ctrl Pts',(190.440853584981,54.4000000000751,112.657855156188));
#91260=CARTESIAN_POINT('Ctrl Pts',(189.981599530965,54.8501814482032,120.693291671663));
#91261=CARTESIAN_POINT('Ctrl Pts',(190.263931815988,54.7136847329145,120.700844105146));
#91262=CARTESIAN_POINT('Ctrl Pts',(190.263931816014,54.3999999999636,120.700844105169));
#91263=CARTESIAN_POINT('Ctrl Pts',(189.905525199068,54.8501814482593,123.31496616946));
#91264=CARTESIAN_POINT('Ctrl Pts',(190.187813351298,54.7136847330329,123.324152150651));
#91265=CARTESIAN_POINT('Ctrl Pts',(190.187813351256,54.4000000000363,123.324152150649));
#91266=CARTESIAN_POINT('Ctrl Pts',(189.696750321874,54.850181448191,128.556852744112));
#91267=CARTESIAN_POINT('Ctrl Pts',(189.978874876793,54.7136847328917,128.570146301895));
#91268=CARTESIAN_POINT('Ctrl Pts',(189.978874876835,54.3999999999636,128.570146301897));
#91269=CARTESIAN_POINT('Ctrl Pts',(189.564190785202,54.8501814482593,131.177068260088));
#91270=CARTESIAN_POINT('Ctrl Pts',(189.846197509667,54.7136847330329,131.192833544529));
#91271=CARTESIAN_POINT('Ctrl Pts',(189.84619750958,54.4000000000363,131.192833544524));
#91272=CARTESIAN_POINT('Ctrl Pts',(189.21373904357,54.850181448191,136.415271144211));
#91273=CARTESIAN_POINT('Ctrl Pts',(189.495332574474,54.7136847328916,136.437212434963));
#91274=CARTESIAN_POINT('Ctrl Pts',(189.495332574561,54.3999999999636,136.437212434969));
#91275=CARTESIAN_POINT('Ctrl Pts',(188.995975118318,54.8501814482251,139.034428718839));
#91276=CARTESIAN_POINT('Ctrl Pts',(189.277277045309,54.7136847329623,139.060072711156));
#91277=CARTESIAN_POINT('Ctrl Pts',(189.277277045221,54.3999999999999,139.060072711146));
#91278=CARTESIAN_POINT('Ctrl Pts',(188.432225703268,54.8501814482251,144.264463671248));
#91279=CARTESIAN_POINT('Ctrl Pts',(188.71253077521,54.7136847329623,144.299355721209));
#91280=CARTESIAN_POINT('Ctrl Pts',(188.712530775298,54.3999999999999,144.299355721219));
#91281=CARTESIAN_POINT('Ctrl Pts',(188.087304668474,54.8501814482349,146.868271499025));
#91282=CARTESIAN_POINT('Ctrl Pts',(188.366914065688,54.7136847329872,146.908694703911));
#91283=CARTESIAN_POINT('Ctrl Pts',(188.366914065557,54.4000000000363,146.908694703889));
#91284=CARTESIAN_POINT('Ctrl Pts',(187.208321751508,54.8501814482154,152.042290376387));
#91285=CARTESIAN_POINT('Ctrl Pts',(187.485593746244,54.7136847329374,152.096472398439));
#91286=CARTESIAN_POINT('Ctrl Pts',(187.485593746376,54.3999999999636,152.096472398462));
#91287=CARTESIAN_POINT('Ctrl Pts',(186.674882433875,54.8501814482251,154.612621948317));
#91288=CARTESIAN_POINT('Ctrl Pts',(186.950529717102,54.7136847329623,154.675038288882));
#91289=CARTESIAN_POINT('Ctrl Pts',(186.950529716886,54.3999999999999,154.675038288824));
#91290=CARTESIAN_POINT('Ctrl Pts',(185.829068982087,54.8501814482251,157.793689708649));
#91291=CARTESIAN_POINT('Ctrl Pts',(186.101340342461,54.7136847329623,157.868802749258));
#91292=CARTESIAN_POINT('Ctrl Pts',(186.101340342515,54.3999999999999,157.868802749272));
#91293=CARTESIAN_POINT('Ctrl Pts',(185.650840070459,54.850181448231,158.428289553895));
#91294=CARTESIAN_POINT('Ctrl Pts',(185.922366535571,54.713684732974,158.50606230595));
#91295=CARTESIAN_POINT('Ctrl Pts',(185.922366535509,54.4000000000045,158.506062305931));
#91296=CARTESIAN_POINT('Ctrl Pts',(185.274189105931,54.8501814482193,159.693888916717));
#91297=CARTESIAN_POINT('Ctrl Pts',(185.544055877709,54.7136847329506,159.77723846825));
#91298=CARTESIAN_POINT('Ctrl Pts',(185.544055877772,54.3999999999954,159.777238468269));
#91299=CARTESIAN_POINT('Ctrl Pts',(185.075603523205,54.8501814482251,160.325278084653));
#91300=CARTESIAN_POINT('Ctrl Pts',(185.344554566279,54.7136847329623,160.411547100408));
#91301=CARTESIAN_POINT('Ctrl Pts',(185.344554566236,54.3999999999999,160.411547100394));
#91302=CARTESIAN_POINT('Ctrl Pts',(184.449826482446,54.8501814482251,162.202753795278));
#91303=CARTESIAN_POINT('Ctrl Pts',(184.715740727713,54.7136847329623,162.298133906292));
#91304=CARTESIAN_POINT('Ctrl Pts',(184.715740727799,54.3999999999999,162.298133906321));
#91305=CARTESIAN_POINT('Ctrl Pts',(183.991757248688,54.8501814482251,163.43542835655));
#91306=CARTESIAN_POINT('Ctrl Pts',(184.255257809005,54.7136847329623,163.537370813413));
#91307=CARTESIAN_POINT('Ctrl Pts',(184.255257808904,54.3999999999999,163.53737081337));
#91308=CARTESIAN_POINT('Ctrl Pts',(182.473253277925,54.8501814482251,167.066305711601));
#91309=CARTESIAN_POINT('Ctrl Pts',(182.727934619225,54.7136847329623,167.189335701864));
#91310=CARTESIAN_POINT('Ctrl Pts',(182.727934619428,54.3999999999999,167.189335701949));
#91311=CARTESIAN_POINT('Ctrl Pts',(181.268987344943,54.8501814481749,169.397698176221));
#91312=CARTESIAN_POINT('Ctrl Pts',(181.515620921969,54.7136847328548,169.536771595712));
#91313=CARTESIAN_POINT('Ctrl Pts',(181.515620921781,54.3999999999268,169.536771595573));
#91314=CARTESIAN_POINT('Ctrl Pts',(179.441582135828,54.8501814482377,172.160422815342));
#91315=CARTESIAN_POINT('Ctrl Pts',(179.674375772127,54.7136847329892,172.32041986224));
#91316=CARTESIAN_POINT('Ctrl Pts',(179.674375772174,54.4000000000182,172.320419862275));
#91317=CARTESIAN_POINT('Ctrl Pts',(179.058647571677,54.8501814482279,172.707019013959));
#91318=CARTESIAN_POINT('Ctrl Pts',(179.288478943293,54.7136847329684,172.871248799738));
#91319=CARTESIAN_POINT('Ctrl Pts',(179.288478943292,54.4000000000046,172.871248799737));
#91320=CARTESIAN_POINT('Ctrl Pts',(178.268178494805,54.8501814482224,173.771202442769));
#91321=CARTESIAN_POINT('Ctrl Pts',(178.491798868746,54.7136847329563,173.943793897587));
#91322=CARTESIAN_POINT('Ctrl Pts',(178.491798868747,54.3999999999954,173.943793897587));
#91323=CARTESIAN_POINT('Ctrl Pts',(177.860133057982,54.8501814482298,174.289776895294));
#91324=CARTESIAN_POINT('Ctrl Pts',(178.080501288023,54.7136847329709,174.466503936161));
#91325=CARTESIAN_POINT('Ctrl Pts',(178.080501288033,54.4,174.466503936169));
#91326=CARTESIAN_POINT('Ctrl Pts',(176.597748388822,54.8501814482161,175.805008910674));
#91327=CARTESIAN_POINT('Ctrl Pts',(176.80798357003,54.7136847329453,175.993898583381));
#91328=CARTESIAN_POINT('Ctrl Pts',(176.807983570011,54.4,175.993898583365));
#91329=CARTESIAN_POINT('Ctrl Pts',(175.705080835993,54.850181448236,176.761087998022));
#91330=CARTESIAN_POINT('Ctrl Pts',(175.908054306141,54.713684732986,176.957753246188));
#91331=CARTESIAN_POINT('Ctrl Pts',(175.908054306173,54.400000000018,176.957753246221));
#91332=CARTESIAN_POINT('Ctrl Pts',(173.820641754199,54.8501814482143,178.567587618226));
#91333=CARTESIAN_POINT('Ctrl Pts',(174.008563362028,54.7136847329387,178.778682191129));
#91334=CARTESIAN_POINT('Ctrl Pts',(174.008563361996,54.399999999982,178.778682191095));
#91335=CARTESIAN_POINT('Ctrl Pts',(172.828892835169,54.8501814482297,179.418025890271));
#91336=CARTESIAN_POINT('Ctrl Pts',(173.009030242955,54.7136847329708,179.635772395387));
#91337=CARTESIAN_POINT('Ctrl Pts',(173.009030242992,54.4,179.635772395448));
#91338=CARTESIAN_POINT('Ctrl Pts',(171.270964235975,54.8501814482229,180.618253074959));
#91339=CARTESIAN_POINT('Ctrl Pts',(171.43944285178,54.7136847329581,180.844981505819));
#91340=CARTESIAN_POINT('Ctrl Pts',(171.439442851761,54.4,180.844981505789));
#91341=CARTESIAN_POINT('Ctrl Pts',(170.739952716052,54.8501814482214,181.005775429243));
#91342=CARTESIAN_POINT('Ctrl Pts',(170.904547815832,54.7136847329552,181.235334021093));
#91343=CARTESIAN_POINT('Ctrl Pts',(170.904547815849,54.4,181.235334021119));
#91344=CARTESIAN_POINT('Ctrl Pts',(169.655345316385,54.850181448229,181.756533782417));
#91345=CARTESIAN_POINT('Ctrl Pts',(169.812238466112,54.7136847329695,181.991423615145));
#91346=CARTESIAN_POINT('Ctrl Pts',(169.812238466095,54.4,181.991423615119));
#91347=CARTESIAN_POINT('Ctrl Pts',(169.100565571154,54.8501814482237,182.120500287617));
#91348=CARTESIAN_POINT('Ctrl Pts',(169.253632525607,54.7136847329595,182.357896135585));
#91349=CARTESIAN_POINT('Ctrl Pts',(169.253632525641,54.4,182.357896135649));
#91350=CARTESIAN_POINT('Ctrl Pts',(166.286156024425,54.8501814482313,183.87344972053));
#91351=CARTESIAN_POINT('Ctrl Pts',(166.420470654194,54.7136847329738,184.122525416709));
#91352=CARTESIAN_POINT('Ctrl Pts',(166.420470654058,54.4,184.122525416454));
#91353=CARTESIAN_POINT('Ctrl Pts',(163.940300566172,54.8501814482033,185.044287598079));
#91354=CARTESIAN_POINT('Ctrl Pts',(164.06114669688,54.7136847329148,185.299869237578));
#91355=CARTESIAN_POINT('Ctrl Pts',(164.061146696941,54.3999999999638,185.299869237723));
#91356=CARTESIAN_POINT('Ctrl Pts',(159.119184755956,54.8501814482469,187.065920062995));
#91357=CARTESIAN_POINT('Ctrl Pts',(159.216773571118,54.7136847330098,187.331254163407));
#91358=CARTESIAN_POINT('Ctrl Pts',(159.216773571057,54.4000000000361,187.331254163262));
#91359=CARTESIAN_POINT('Ctrl Pts',(156.643629215511,54.850181448213,187.916140584353));
#91360=CARTESIAN_POINT('Ctrl Pts',(156.731364791414,54.7136847329395,188.184741416756));
#91361=CARTESIAN_POINT('Ctrl Pts',(156.731364791459,54.4,188.184741416887));
#91362=CARTESIAN_POINT('Ctrl Pts',(152.861957700333,54.8501814482313,189.022509905896));
#91363=CARTESIAN_POINT('Ctrl Pts',(152.937045612347,54.7136847329737,189.294810950442));
#91364=CARTESIAN_POINT('Ctrl Pts',(152.937045612325,54.4,189.294810950376));
#91365=CARTESIAN_POINT('Ctrl Pts',(151.588783040648,54.8501814482142,189.363028174597));
#91366=CARTESIAN_POINT('Ctrl Pts',(151.660004270742,54.7136847329384,189.636355189729));
#91367=CARTESIAN_POINT('Ctrl Pts',(151.660004270758,54.3999999999818,189.636355189793));
#91368=CARTESIAN_POINT('Ctrl Pts',(149.037627503664,54.8501814482361,189.99264387881));
#91369=CARTESIAN_POINT('Ctrl Pts',(149.10175078131,54.7136847329862,190.267722642176));
#91370=CARTESIAN_POINT('Ctrl Pts',(149.101750781294,54.4000000000181,190.267722642112));
#91371=CARTESIAN_POINT('Ctrl Pts',(147.757825267386,54.8501814482032,190.282313053568));
#91372=CARTESIAN_POINT('Ctrl Pts',(147.818710308861,54.7136847329145,190.558119250698));
#91373=CARTESIAN_POINT('Ctrl Pts',(147.818710308865,54.3999999999636,190.558119250731));
#91374=CARTESIAN_POINT('Ctrl Pts',(143.907886586798,54.8501814482689,191.088733427083));
#91375=CARTESIAN_POINT('Ctrl Pts',(143.959822853609,54.7136847330577,191.36641406294));
#91376=CARTESIAN_POINT('Ctrl Pts',(143.9598228536,54.4000000000726,191.366414062873));
#91377=CARTESIAN_POINT('Ctrl Pts',(141.327319087948,54.8501814482045,191.543506604474));
#91378=CARTESIAN_POINT('Ctrl Pts',(141.374302221674,54.7136847329135,191.822034897082));
#91379=CARTESIAN_POINT('Ctrl Pts',(141.374302221683,54.3999999999455,191.822034897143));
#91380=CARTESIAN_POINT('Ctrl Pts',(135.976046370232,54.8501814482472,192.362205111029));
#91381=CARTESIAN_POINT('Ctrl Pts',(136.014207098472,54.7136847330143,192.642083155408));
#91382=CARTESIAN_POINT('Ctrl Pts',(136.014207098463,54.400000000058,192.642083155343));
#91383=CARTESIAN_POINT('Ctrl Pts',(133.203932918804,54.8501814482507,192.717861291362));
#91384=CARTESIAN_POINT('Ctrl Pts',(133.238324066358,54.7136847330163,192.998208138289));
#91385=CARTESIAN_POINT('Ctrl Pts',(133.238324066359,54.4000000000337,192.998208138274));
#91386=CARTESIAN_POINT('Ctrl Pts',(130.423832944263,54.8501814482199,193.026279994343));
#91387=CARTESIAN_POINT('Ctrl Pts',(130.454964793654,54.713684732951,193.306989106035));
#91388=CARTESIAN_POINT('Ctrl Pts',(130.454964793654,54.3999999999926,193.306989106039));
#91389=CARTESIAN_POINT('',(130.970210996039,54.4,193.249273457296));
#91390=CARTESIAN_POINT('Origin',(130.914017984099,54.4,192.752441145644));
#91391=CARTESIAN_POINT('Ctrl Pts',(190.499797482064,54.4,102.3353360815));
#91392=CARTESIAN_POINT('Ctrl Pts',(190.262688257762,54.4,166.865108618385));
#91393=CARTESIAN_POINT('Ctrl Pts',(186.165595197882,54.4,187.00653358103));
#91394=CARTESIAN_POINT('Ctrl Pts',(130.970210995984,54.4,193.249273456807));
#91395=CARTESIAN_POINT('Origin',(-205.7,54.4,40.5));
#91396=CARTESIAN_POINT('',(-189.5,54.4,40.));
#91397=CARTESIAN_POINT('Origin',(-189.5,54.4,40.5));
#91398=CARTESIAN_POINT('',(189.5,54.4,40.));
#91399=CARTESIAN_POINT('Ctrl Pts',(127.255088949806,54.5666666666668,193.698954356396));
#91400=CARTESIAN_POINT('Ctrl Pts',(127.245376536202,54.7908851649001,193.620278369648));
#91401=CARTESIAN_POINT('Ctrl Pts',(127.217936735184,54.8708716449131,193.398000621877));
#91402=CARTESIAN_POINT('Ctrl Pts',(127.879084413169,54.5518028860853,193.627218234101));
#91403=CARTESIAN_POINT('Ctrl Pts',(127.874066995385,54.7851572329741,193.55278227821));
#91404=CARTESIAN_POINT('Ctrl Pts',(127.842033796868,54.8694502963056,193.324965268805));
#91405=CARTESIAN_POINT('Ctrl Pts',(128.500935272669,54.5302082089312,193.550095813408));
#91406=CARTESIAN_POINT('Ctrl Pts',(128.501328716631,54.7766711456716,193.482509467744));
#91407=CARTESIAN_POINT('Ctrl Pts',(128.464930906231,54.8673636527269,193.246434626864));
#91408=CARTESIAN_POINT('Ctrl Pts',(129.739491935211,54.4743280441491,193.395855537281));
#91409=CARTESIAN_POINT('Ctrl Pts',(129.743550596673,54.7536109502607,193.352491272635));
#91410=CARTESIAN_POINT('Ctrl Pts',(129.704532450547,54.8618212857288,193.094336154531));
#91411=CARTESIAN_POINT('Ctrl Pts',(130.356219027086,54.4400417824632,193.318717527232));
#91412=CARTESIAN_POINT('Ctrl Pts',(130.368680695371,54.7386547278232,193.292148787355));
#91413=CARTESIAN_POINT('Ctrl Pts',(130.326591494069,54.8583196432092,193.020261309429));
#91414=CARTESIAN_POINT('Ctrl Pts',(130.970210995984,54.4,193.249273456807));
#91415=CARTESIAN_POINT('Ctrl Pts',(130.970210995984,54.7201169082854,193.249273456807));
#91416=CARTESIAN_POINT('Ctrl Pts',(130.937537062709,54.85409895477,192.960385831121));
#91417=CARTESIAN_POINT('',(127.255088949811,54.5666666666664,193.698954356395));
#91418=CARTESIAN_POINT('Origin',(127.197333301155,54.4,193.231101273397));
#91419=CARTESIAN_POINT('Ctrl Pts',(130.970210995984,54.4,193.249273456807));
#91420=CARTESIAN_POINT('Ctrl Pts',(130.614606575102,54.4231909138639,193.289493231166));
#91421=CARTESIAN_POINT('Ctrl Pts',(130.259170754114,54.4443808577405,193.332166063808));
#91422=CARTESIAN_POINT('Ctrl Pts',(129.903752824151,54.4635009794963,193.375799905195));
#91423=CARTESIAN_POINT('Ctrl Pts',(129.642584059729,54.4775508575514,193.407862993411));
#91424=CARTESIAN_POINT('Ctrl Pts',(129.381424839028,54.4904830162573,193.440446446569));
#91425=CARTESIAN_POINT('Ctrl Pts',(129.12021360394,54.5022681265401,193.472975675345));
#91426=CARTESIAN_POINT('Ctrl Pts',(128.658090984803,54.5231177888026,193.530524855399));
#91427=CARTESIAN_POINT('Ctrl Pts',(128.19579463262,54.5403791895002,193.587914070895));
#91428=CARTESIAN_POINT('Ctrl Pts',(127.733073441423,54.5539583293988,193.642989461962));
#91429=CARTESIAN_POINT('Ctrl Pts',(127.573799286481,54.5586324313707,193.661947068696));
#91430=CARTESIAN_POINT('Ctrl Pts',(127.414474664831,54.5628700456414,193.680630964935));
#91431=CARTESIAN_POINT('Ctrl Pts',(127.255088949811,54.5666666666666,193.698954356395));
#91432=CARTESIAN_POINT('Ctrl Pts',(-190.217944947177,54.85,41.));
#91433=CARTESIAN_POINT('Ctrl Pts',(-190.217944947177,54.85,40.282055052823));
#91434=CARTESIAN_POINT('Ctrl Pts',(-189.5,54.85,40.282055052823));
#91435=CARTESIAN_POINT('Ctrl Pts',(-190.5,54.7133945031366,41.));
#91436=CARTESIAN_POINT('Ctrl Pts',(-190.5,54.7133945031366,40.));
#91437=CARTESIAN_POINT('Ctrl Pts',(-189.5,54.7133945031366,40.));
#91438=CARTESIAN_POINT('Ctrl Pts',(-190.5,54.4,41.));
#91439=CARTESIAN_POINT('Ctrl Pts',(-190.5,54.4,40.));
#91440=CARTESIAN_POINT('Ctrl Pts',(-189.5,54.4,40.));
#91441=CARTESIAN_POINT('',(-190.5,54.4,41.));
#91442=CARTESIAN_POINT('Origin',(-190.,54.4,41.));
#91443=CARTESIAN_POINT('Origin',(-189.5,54.4,41.));
#91444=CARTESIAN_POINT('Ctrl Pts',(123.160667751337,54.5666666666683,194.071736241466));
#91445=CARTESIAN_POINT('Ctrl Pts',(123.155832932771,54.798164012315,193.990032495164));
#91446=CARTESIAN_POINT('Ctrl Pts',(123.142055633115,54.8749333564381,193.757209488378));
#91447=CARTESIAN_POINT('Ctrl Pts',(123.844835624837,54.5829842777358,194.02547137401));
#91448=CARTESIAN_POINT('Ctrl Pts',(123.833025706398,54.8039632931889,193.938950966455));
#91449=CARTESIAN_POINT('Ctrl Pts',(123.819972220688,54.8762595151111,193.713054829141));
#91450=CARTESIAN_POINT('Ctrl Pts',(124.52750939263,54.5910529953054,193.97017604454));
#91451=CARTESIAN_POINT('Ctrl Pts',(124.520341811565,54.8067875878841,193.881257473471));
#91452=CARTESIAN_POINT('Ctrl Pts',(124.502450477311,54.8769102936331,193.659297116951));
#91453=CARTESIAN_POINT('Ctrl Pts',(125.891907678889,54.5910540215352,193.846078596068));
#91454=CARTESIAN_POINT('Ctrl Pts',(125.882915036185,54.8067879458432,193.757325735115));
#91455=CARTESIAN_POINT('Ctrl Pts',(125.860468063284,54.8769103762644,193.53578017915));
#91456=CARTESIAN_POINT('Ctrl Pts',(126.573706760202,54.5829737705273,193.777260604719));
#91457=CARTESIAN_POINT('Ctrl Pts',(126.56969460559,54.8039598662694,193.690031299387));
#91458=CARTESIAN_POINT('Ctrl Pts',(126.5417369025,54.8762586984535,193.465488140134));
#91459=CARTESIAN_POINT('Ctrl Pts',(127.255088949806,54.5666666666668,193.698954356396));
#91460=CARTESIAN_POINT('Ctrl Pts',(127.245061240287,54.7981640123145,193.617724296245));
#91461=CARTESIAN_POINT('Ctrl Pts',(127.216486277851,54.8749333564379,193.38625110558));
#91462=CARTESIAN_POINT('',(123.160667751337,54.5666666666683,194.071736241466));
#91463=CARTESIAN_POINT('Origin',(123.132821104816,54.4,193.601154913214));
#91464=CARTESIAN_POINT('Ctrl Pts',(127.255088949811,54.5666666666664,193.698954356395));
#91465=CARTESIAN_POINT('Ctrl Pts',(126.574306561438,54.5829594156373,193.777191674042));
#91466=CARTESIAN_POINT('Ctrl Pts',(125.892275665928,54.5910531277812,193.84604432789));
#91467=CARTESIAN_POINT('Ctrl Pts',(124.527367138449,54.5910538890815,193.970189781285));
#91468=CARTESIAN_POINT('Ctrl Pts',(123.844381692399,54.5829734511008,194.025502069948));
#91469=CARTESIAN_POINT('Ctrl Pts',(123.160667751337,54.5666666666683,194.071736241466));
#91470=CARTESIAN_POINT('Origin',(-190.,54.4,211.4));
#91471=CARTESIAN_POINT('',(-190.5,54.4,102.225104347671));
#91472=CARTESIAN_POINT('Origin',(-190.,54.4,102.225104347671));
#91473=CARTESIAN_POINT('',(-190.5,54.4,211.4));
#91474=CARTESIAN_POINT('Ctrl Pts',(119.431296799848,54.3999999999989,194.307271119568));
#91475=CARTESIAN_POINT('Ctrl Pts',(119.431296799848,54.7201173502107,194.307271119569));
#91476=CARTESIAN_POINT('Ctrl Pts',(119.4100538882,54.8540992171485,194.017318164862));
#91477=CARTESIAN_POINT('Ctrl Pts',(120.046537134136,54.4400570466082,194.262196579538));
#91478=CARTESIAN_POINT('Ctrl Pts',(120.029404725024,54.7386619686269,194.238375307498));
#91479=CARTESIAN_POINT('Ctrl Pts',(120.020823595006,54.8583214617764,193.963377414171));
#91480=CARTESIAN_POINT('Ctrl Pts',(120.665937074624,54.4743442642813,194.225052062148));
#91481=CARTESIAN_POINT('Ctrl Pts',(120.654018808206,54.7536182484867,194.18314784127));
#91482=CARTESIAN_POINT('Ctrl Pts',(120.645146597598,54.8618231409601,193.922220259519));
#91483=CARTESIAN_POINT('Ctrl Pts',(121.910047618945,54.5302211315643,194.150963131627));
#91484=CARTESIAN_POINT('Ctrl Pts',(121.897385648962,54.7766766101539,194.084574079458));
#91485=CARTESIAN_POINT('Ctrl Pts',(121.890278416236,54.8673650949516,193.845817355955));
#91486=CARTESIAN_POINT('Ctrl Pts',(122.534757882391,54.5518089947801,194.114036622563));
#91487=CARTESIAN_POINT('Ctrl Pts',(122.526207616594,54.7851599104661,194.039920256715));
#91488=CARTESIAN_POINT('Ctrl Pts',(122.516416141673,54.8694510563384,193.810074102007));
#91489=CARTESIAN_POINT('Ctrl Pts',(123.160667751337,54.5666666666683,194.071736241466));
#91490=CARTESIAN_POINT('Ctrl Pts',(123.155984945507,54.7908854465423,193.992601363026));
#91491=CARTESIAN_POINT('Ctrl Pts',(123.142754938,54.8708718087829,193.769027062935));
#91492=CARTESIAN_POINT('',(119.431296819576,54.4000000000025,194.307271388221));
#91493=CARTESIAN_POINT('Origin',(119.394763063948,54.4,193.80860761966));
#91494=CARTESIAN_POINT('Ctrl Pts',(123.160667751337,54.5666666666683,194.071736241466));
#91495=CARTESIAN_POINT('Ctrl Pts',(122.709671237679,54.5559610386616,194.102215588969));
#91496=CARTESIAN_POINT('Ctrl Pts',(122.258621784535,54.5417470109889,194.129947833764));
#91497=CARTESIAN_POINT('Ctrl Pts',(121.807669854806,54.5241144990764,194.157003923459));
#91498=CARTESIAN_POINT('Ctrl Pts',(121.634426284557,54.5173405635085,194.167398143478));
#91499=CARTESIAN_POINT('Ctrl Pts',(121.46119731046,54.5100618706114,194.177692942311));
#91500=CARTESIAN_POINT('Ctrl Pts',(121.287992346785,54.5022826979228,194.188007596887));
#91501=CARTESIAN_POINT('Ctrl Pts',(120.937031470456,54.486519955297,194.208907922908));
#91502=CARTESIAN_POINT('Ctrl Pts',(120.58616849523,54.4687032547822,194.229881013872));
#91503=CARTESIAN_POINT('Ctrl Pts',(120.23549875877,54.448899215471,194.252365264865));
#91504=CARTESIAN_POINT('Ctrl Pts',(119.967302221838,54.4337528420937,194.269561497174));
#91505=CARTESIAN_POINT('Ctrl Pts',(119.699218906683,54.4174438633529,194.287642260639));
#91506=CARTESIAN_POINT('Ctrl Pts',(119.431296799848,54.3999999999989,194.307271119568));
#91507=CARTESIAN_POINT('Origin',(-160.5,54.4,102.225104347671));
#91508=CARTESIAN_POINT('',(-190.499797482064,54.4,102.335336081498));
#91509=CARTESIAN_POINT('Origin',(-189.999800857363,54.4,102.333498885934));
#91510=CARTESIAN_POINT('Origin',(-160.5,54.4,102.225104347671));
#91511=CARTESIAN_POINT('Ctrl Pts',(119.509543988169,54.8500347278621,194.018642428937));
#91512=CARTESIAN_POINT('Ctrl Pts',(119.530234140646,54.7134500006186,194.300009508377));
#91513=CARTESIAN_POINT('Ctrl Pts',(119.530234140646,54.4000000000055,194.300009508373));
#91514=CARTESIAN_POINT('Ctrl Pts',(114.504744574281,54.850034727667,194.386640129845));
#91515=CARTESIAN_POINT('Ctrl Pts',(114.521587596702,54.7134500002014,194.668289990076));
#91516=CARTESIAN_POINT('Ctrl Pts',(114.521587596738,54.399999999722,194.668289990278));
#91517=CARTESIAN_POINT('Ctrl Pts',(109.498634847962,54.8500347277534,194.653631857555));
#91518=CARTESIAN_POINT('Ctrl Pts',(109.512638560261,54.7134500003821,194.935420030612));
#91519=CARTESIAN_POINT('Ctrl Pts',(109.512638560238,54.3999999998262,194.935420030681));
#91520=CARTESIAN_POINT('Ctrl Pts',(99.5180232912834,54.8500347279625,195.06907559322));
#91521=CARTESIAN_POINT('Ctrl Pts',(99.5275013045554,54.7134500008372,195.351052148972));
#91522=CARTESIAN_POINT('Ctrl Pts',(99.5275013045778,54.4000000001726,195.351052148903));
#91523=CARTESIAN_POINT('Ctrl Pts',(94.5434725844513,54.8500347278166,195.217450349044));
#91524=CARTESIAN_POINT('Ctrl Pts',(94.5512583514112,54.7134500005197,195.499472957335));
#91525=CARTESIAN_POINT('Ctrl Pts',(94.5512583514102,54.3999999999309,195.499472957289));
#91526=CARTESIAN_POINT('Ctrl Pts',(84.5934911422877,54.8500347278999,195.444079361659));
#91527=CARTESIAN_POINT('Ctrl Pts',(84.5985539486568,54.7134500007011,195.726163990358));
#91528=CARTESIAN_POINT('Ctrl Pts',(84.5985539486579,54.400000000069,195.726163990404));
#91529=CARTESIAN_POINT('Ctrl Pts',(79.6180568875425,54.8500347278166,195.521957077234));
#91530=CARTESIAN_POINT('Ctrl Pts',(79.6220940664667,54.7134500005197,195.804056143501));
#91531=CARTESIAN_POINT('Ctrl Pts',(79.622094066466,54.3999999999309,195.804056143444));
#91532=CARTESIAN_POINT('Ctrl Pts',(69.666675118241,54.8500347279,195.635564432718));
#91533=CARTESIAN_POINT('Ctrl Pts',(69.6690791730593,54.7134500007011,195.917682143204));
#91534=CARTESIAN_POINT('Ctrl Pts',(69.66907917306,54.400000000069,195.91768214326));
#91535=CARTESIAN_POINT('Ctrl Pts',(64.6907256720555,54.8500347278351,195.671107949031));
#91536=CARTESIAN_POINT('Ctrl Pts',(64.6925245012106,54.7134500005671,195.953229373737));
#91537=CARTESIAN_POINT('Ctrl Pts',(64.6925245012109,54.4,195.953229373792));
#91538=CARTESIAN_POINT('Ctrl Pts',(49.7624773894366,54.8500347279047,195.741536462924));
#91539=CARTESIAN_POINT('Ctrl Pts',(49.7628727410856,54.713450000697,196.023664508782));
#91540=CARTESIAN_POINT('Ctrl Pts',(49.7628727410851,54.4,196.023664508672));
#91541=CARTESIAN_POINT('Ctrl Pts',(39.8097639074172,54.850034728025,195.741812920426));
#91542=CARTESIAN_POINT('Ctrl Pts',(39.8097607474161,54.7134500009732,196.023939735264));
#91543=CARTESIAN_POINT('Ctrl Pts',(39.809760747416,54.4000000002762,196.023939735262));
#91544=CARTESIAN_POINT('Ctrl Pts',(19.8716555149193,54.850034727691,195.730534471012));
#91545=CARTESIAN_POINT('Ctrl Pts',(19.8713389735597,54.7134500002464,196.012661108492));
#91546=CARTESIAN_POINT('Ctrl Pts',(19.8713389735597,54.3999999997228,196.012661108494));
#91547=CARTESIAN_POINT('Ctrl Pts',(9.88631306985696,54.8500347271157,195.717789107939));
#91548=CARTESIAN_POINT('Ctrl Pts',(9.8860970633918,54.7134499989911,195.999915879995));
#91549=CARTESIAN_POINT('Ctrl Pts',(9.88609706339176,54.3999999987505,195.999915880082));
#91550=CARTESIAN_POINT('Ctrl Pts',(-0.0989467222038218,54.8500347278657,
195.717873647057));
#91551=CARTESIAN_POINT('Ctrl Pts',(-0.0989445642066252,54.7134500006265,
196.000000418499));
#91552=CARTESIAN_POINT('Ctrl Pts',(-0.0989445642066248,54.4000000000124,
196.000000418498));
#91553=CARTESIAN_POINT('',(1.2169238626783E-14,54.4,196.));
#91554=CARTESIAN_POINT('Origin',(1.20273620013996E-14,54.4,195.5));
#91555=CARTESIAN_POINT('Ctrl Pts',(119.431296799848,54.4,194.307271119568));
#91556=CARTESIAN_POINT('Ctrl Pts',(116.259838254169,54.4000000000022,194.539622653112));
#91557=CARTESIAN_POINT('Ctrl Pts',(113.087577822492,54.4000000000016,194.731577999437));
#91558=CARTESIAN_POINT('Ctrl Pts',(109.914729036557,54.4000000000232,194.893888974244));
#91559=CARTESIAN_POINT('Ctrl Pts',(108.111189387205,54.4000000000355,194.98615125913));
#91560=CARTESIAN_POINT('Ctrl Pts',(106.307459615187,54.4000000000549,195.068835854631));
#91561=CARTESIAN_POINT('Ctrl Pts',(104.503579022491,54.4000000000862,195.143922525206));
#91562=CARTESIAN_POINT('Ctrl Pts',(100.210957862777,54.4000000001608,195.322603216282));
#91563=CARTESIAN_POINT('Ctrl Pts',(95.9174700273534,54.4000000000422,195.457621859572));
#91564=CARTESIAN_POINT('Ctrl Pts',(91.6234160517253,54.4000000000305,195.564117476063));
#91565=CARTESIAN_POINT('Ctrl Pts',(90.9405933301759,54.4000000000286,195.581051968992));
#91566=CARTESIAN_POINT('Ctrl Pts',(90.2577562959791,54.4000000000294,195.597265313742));
#91567=CARTESIAN_POINT('Ctrl Pts',(89.574906150034,54.4000000000342,195.612818473846));
#91568=CARTESIAN_POINT('Ctrl Pts',(84.599074668863,54.4000000000691,195.726152130049));
#91569=CARTESIAN_POINT('Ctrl Pts',(79.622539877546,54.3999999999996,195.804051053958));
#91570=CARTESIAN_POINT('Ctrl Pts',(74.645586619763,54.4000000000343,195.860869143352));
#91571=CARTESIAN_POINT('Ctrl Pts',(69.6694102398991,54.400000000069,195.917678363722));
#91572=CARTESIAN_POINT('Ctrl Pts',(64.6928118455221,54.4,195.953228018159));
#91573=CARTESIAN_POINT('Ctrl Pts',(59.7159739145023,54.4000000000001,195.976707752086));
#91574=CARTESIAN_POINT('Ctrl Pts',(52.1214119494974,54.4000000000002,196.012537388634));
#91575=CARTESIAN_POINT('Ctrl Pts',(44.526289196523,54.400000000161,196.021189119254));
#91576=CARTESIAN_POINT('Ctrl Pts',(36.9310173515837,54.4000000001757,196.020774649485));
#91577=CARTESIAN_POINT('Ctrl Pts',(34.5730357339827,54.4000000001802,196.020645975737));
#91578=CARTESIAN_POINT('Ctrl Pts',(32.2150397510362,54.4000000001706,196.019643606687));
#91579=CARTESIAN_POINT('Ctrl Pts',(29.85704171195,54.400000000138,196.018309750873));
#91580=CARTESIAN_POINT('Ctrl Pts',(19.9046938155966,54.4000000000001,196.012679976427));
#91581=CARTESIAN_POINT('Ctrl Pts',(9.9523497061253,54.4,196.));
#91582=CARTESIAN_POINT('Ctrl Pts',(1.4210854715202E-14,54.4,196.));
#91583=CARTESIAN_POINT('Ctrl Pts',(0.108339742257026,54.8500380311149,195.717866914955));
#91584=CARTESIAN_POINT('Ctrl Pts',(0.108337388749144,54.713455280679,196.00000050967));
#91585=CARTESIAN_POINT('Ctrl Pts',(0.108337388749144,54.4,196.000000509671));
#91586=CARTESIAN_POINT('Ctrl Pts',(-10.6394131523854,54.8500380311152,195.717765695086));
#91587=CARTESIAN_POINT('Ctrl Pts',(-10.6391815802582,54.7134552806797,195.999899290541));
#91588=CARTESIAN_POINT('Ctrl Pts',(-10.6391815802582,54.400000000001,195.999899290448));
#91589=CARTESIAN_POINT('Ctrl Pts',(-21.3873590267281,54.850038031075,195.732769603628));
#91590=CARTESIAN_POINT('Ctrl Pts',(-21.3870266129879,54.7134552805766,196.014903083131));
#91591=CARTESIAN_POINT('Ctrl Pts',(-21.3870266129879,54.3999999998508,196.01490308311));
#91592=CARTESIAN_POINT('Ctrl Pts',(-42.8474989701256,54.8500380311547,195.741830949266));
#91593=CARTESIAN_POINT('Ctrl Pts',(-42.8475924106281,54.7134552807811,196.023964608597));
#91594=CARTESIAN_POINT('Ctrl Pts',(-42.8475924106281,54.4000000001486,196.023964608617));
#91595=CARTESIAN_POINT('Ctrl Pts',(-53.5596885725384,54.8500380310701,195.737760364647));
#91596=CARTESIAN_POINT('Ctrl Pts',(-53.5602852852272,54.7134552805814,196.019895896344));
#91597=CARTESIAN_POINT('Ctrl Pts',(-53.5602852852272,54.3999999999257,196.019895896344));
#91598=CARTESIAN_POINT('Ctrl Pts',(-69.6282502861437,54.8500380311374,195.635215850766));
#91599=CARTESIAN_POINT('Ctrl Pts',(-69.6306526067851,54.7134552807279,195.917339859647));
#91600=CARTESIAN_POINT('Ctrl Pts',(-69.6306526067851,54.4000000000371,195.917339859647));
#91601=CARTESIAN_POINT('Ctrl Pts',(-74.9844840288523,54.85003803109,195.584389730407));
#91602=CARTESIAN_POINT('Ctrl Pts',(-74.9876678043094,54.7134552806324,195.866507396244));
#91603=CARTESIAN_POINT('Ctrl Pts',(-74.9876678043095,54.4,195.866507396251));
#91604=CARTESIAN_POINT('Ctrl Pts',(-85.6970676947234,54.8500380311399,195.422795957478));
#91605=CARTESIAN_POINT('Ctrl Pts',(-85.7023946291779,54.7134552807256,195.704881294905));
#91606=CARTESIAN_POINT('Ctrl Pts',(-85.7023946291778,54.4,195.704881294898));
#91607=CARTESIAN_POINT('Ctrl Pts',(-91.0540074351636,54.8500380310899,195.312362346734));
#91608=CARTESIAN_POINT('Ctrl Pts',(-91.0606918126211,54.7134552806324,195.594422790046));
#91609=CARTESIAN_POINT('Ctrl Pts',(-91.0606918126185,54.4,195.594422789961));
#91610=CARTESIAN_POINT('Ctrl Pts',(-101.765528158601,54.8500380311399,194.988364284601));
#91611=CARTESIAN_POINT('Ctrl Pts',(-101.775903721038,54.7134552807256,195.270313078383));
#91612=CARTESIAN_POINT('Ctrl Pts',(-101.775903721041,54.4,195.270313078468));
#91613=CARTESIAN_POINT('Ctrl Pts',(-107.117526535979,54.85003803109,194.775617671763));
#91614=CARTESIAN_POINT('Ctrl Pts',(-107.130224336239,54.7134552806325,195.057483582586));
#91615=CARTESIAN_POINT('Ctrl Pts',(-107.130224336237,54.4,195.057483582537));
#91616=CARTESIAN_POINT('Ctrl Pts',(-117.808411473944,54.8500380311399,194.172315411311));
#91617=CARTESIAN_POINT('Ctrl Pts',(-117.827505515306,54.7134552807256,194.4538203729));
#91618=CARTESIAN_POINT('Ctrl Pts',(-117.827505515308,54.4,194.453820372949));
#91619=CARTESIAN_POINT('Ctrl Pts',(-123.147427885218,54.8500380310477,193.783642561154));
#91620=CARTESIAN_POINT('Ctrl Pts',(-123.170566875538,54.7134552805327,194.064885467444));
#91621=CARTESIAN_POINT('Ctrl Pts',(-123.170566875529,54.3999999998886,194.064885467356));
#91622=CARTESIAN_POINT('Ctrl Pts',(-131.13843404817,54.8500380311486,192.960571233706));
#91623=CARTESIAN_POINT('Ctrl Pts',(-131.170224675515,54.7134552807522,193.240923023929));
#91624=CARTESIAN_POINT('Ctrl Pts',(-131.170224675519,54.4000000000557,193.240923023973));
#91625=CARTESIAN_POINT('Ctrl Pts',(-133.799137053305,54.850038031115,192.64554864504));
#91626=CARTESIAN_POINT('Ctrl Pts',(-133.834251546657,54.7134552806791,192.925517262509));
#91627=CARTESIAN_POINT('Ctrl Pts',(-133.83425154665,54.4,192.925517262463));
#91628=CARTESIAN_POINT('Ctrl Pts',(-137.784045656388,54.850038031115,192.088101643795));
#91629=CARTESIAN_POINT('Ctrl Pts',(-137.825118822442,54.7134552806791,192.367236705357));
#91630=CARTESIAN_POINT('Ctrl Pts',(-137.825118822446,54.4,192.367236705381));
#91631=CARTESIAN_POINT('Ctrl Pts',(-139.111317684321,54.8500380311093,191.888039824932));
#91632=CARTESIAN_POINT('Ctrl Pts',(-139.154540611851,54.7134552806668,192.16685305033));
#91633=CARTESIAN_POINT('Ctrl Pts',(-139.154540611846,54.3999999999906,192.166853050303));
#91634=CARTESIAN_POINT('Ctrl Pts',(-141.763413284886,54.8500380311205,191.453946490174));
#91635=CARTESIAN_POINT('Ctrl Pts',(-141.811336381098,54.7134552806912,191.731990394955));
#91636=CARTESIAN_POINT('Ctrl Pts',(-141.811336381103,54.4000000000093,191.731990394983));
#91637=CARTESIAN_POINT('Ctrl Pts',(-143.089131113363,54.8500380311149,191.21973202617));
#91638=CARTESIAN_POINT('Ctrl Pts',(-143.13960666561,54.713455280679,191.497328231515));
#91639=CARTESIAN_POINT('Ctrl Pts',(-143.139606665603,54.3999999999999,191.497328231476));
#91640=CARTESIAN_POINT('Ctrl Pts',(-147.049213256429,54.8500380311149,190.458401104656));
#91641=CARTESIAN_POINT('Ctrl Pts',(-147.108057529445,54.713455280679,190.734388412647));
#91642=CARTESIAN_POINT('Ctrl Pts',(-147.10805752946,54.3999999999999,190.734388412724));
#91643=CARTESIAN_POINT('Ctrl Pts',(-149.669664355132,54.8500380311374,189.87321359446));
#91644=CARTESIAN_POINT('Ctrl Pts',(-149.735031156289,54.7134552807278,190.147792646779));
#91645=CARTESIAN_POINT('Ctrl Pts',(-149.735031156257,54.4000000000371,190.147792646636));
#91646=CARTESIAN_POINT('Ctrl Pts',(-153.558016900812,54.8500380311037,188.827413937642));
#91647=CARTESIAN_POINT('Ctrl Pts',(-153.63525005315,54.7134552806546,189.09880145176));
#91648=CARTESIAN_POINT('Ctrl Pts',(-153.635250053166,54.3999999999814,189.098801451831));
#91649=CARTESIAN_POINT('Ctrl Pts',(-154.847024685085,54.8500380311262,188.450588263097));
#91650=CARTESIAN_POINT('Ctrl Pts',(-154.928562946899,54.7134552807035,188.720727975034));
#91651=CARTESIAN_POINT('Ctrl Pts',(-154.928562946869,54.4000000000186,188.720727974942));
#91652=CARTESIAN_POINT('Ctrl Pts',(-157.4077546348,54.8500380311037,187.628297179058));
#91653=CARTESIAN_POINT('Ctrl Pts',(-157.49873505085,54.7134552806546,187.895404865313));
#91654=CARTESIAN_POINT('Ctrl Pts',(-157.49873505088,54.3999999999814,187.895404865405));
#91655=CARTESIAN_POINT('Ctrl Pts',(-158.680882160903,54.8500380311149,187.182323197846));
#91656=CARTESIAN_POINT('Ctrl Pts',(-158.777006808681,54.713455280679,187.447644908254));
#91657=CARTESIAN_POINT('Ctrl Pts',(-158.777006808645,54.3999999999999,187.447644908159));
#91658=CARTESIAN_POINT('Ctrl Pts',(-162.459478912646,54.8500380311149,185.7214999272));
#91659=CARTESIAN_POINT('Ctrl Pts',(-162.572437434655,54.713455280679,185.980313582809));
#91660=CARTESIAN_POINT('Ctrl Pts',(-162.572437434729,54.3999999999999,185.980313583));
#91661=CARTESIAN_POINT('Ctrl Pts',(-164.895955520428,54.850038031131,184.59598819763));
#91662=CARTESIAN_POINT('Ctrl Pts',(-165.021947502474,54.713455280716,184.848989685855));
#91663=CARTESIAN_POINT('Ctrl Pts',(-165.021947502338,54.4000000000369,184.848989685658));
#91664=CARTESIAN_POINT('Ctrl Pts',(-168.378946346957,54.8500380311069,182.593720138746));
#91665=CARTESIAN_POINT('Ctrl Pts',(-168.526867773834,54.7134552806605,182.834115040126));
#91666=CARTESIAN_POINT('Ctrl Pts',(-168.526867773903,54.3999999999815,182.834115040225));
#91667=CARTESIAN_POINT('Ctrl Pts',(-169.511164536588,54.8500380311165,181.873697436862));
#91668=CARTESIAN_POINT('Ctrl Pts',(-169.666776786271,54.7134552806819,182.10923579638));
#91669=CARTESIAN_POINT('Ctrl Pts',(-169.666776786166,54.3999999999999,182.109235796261));
#91670=CARTESIAN_POINT('Ctrl Pts',(-171.158953560921,54.8500380311141,180.701771054281));
#91671=CARTESIAN_POINT('Ctrl Pts',(-171.326425106144,54.7134552806775,180.928874947439));
#91672=CARTESIAN_POINT('Ctrl Pts',(-171.326425106196,54.3999999999999,180.928874947498));
#91673=CARTESIAN_POINT('Ctrl Pts',(-171.699784041561,54.8500380311085,180.29579974264));
#91674=CARTESIAN_POINT('Ctrl Pts',(-171.871260701899,54.7134552806652,180.519901406512));
#91675=CARTESIAN_POINT('Ctrl Pts',(-171.871260701859,54.3999999999906,180.519901406447));
#91676=CARTESIAN_POINT('Ctrl Pts',(-172.763252852148,54.8500380311214,179.450899492048));
#91677=CARTESIAN_POINT('Ctrl Pts',(-172.942780916033,54.7134552806928,179.668604510617));
#91678=CARTESIAN_POINT('Ctrl Pts',(-172.942780916073,54.4000000000093,179.668604510682));
#91679=CARTESIAN_POINT('Ctrl Pts',(-173.284583847363,54.8500380311172,179.01282876578));
#91680=CARTESIAN_POINT('Ctrl Pts',(-173.468148508317,54.7134552806834,179.227145347675));
#91681=CARTESIAN_POINT('Ctrl Pts',(-173.468148508316,54.3999999999999,179.227145347668));
#91682=CARTESIAN_POINT('Ctrl Pts',(-175.810760829173,54.8500380311055,176.765322607494));
#91683=CARTESIAN_POINT('Ctrl Pts',(-176.014168613311,54.7134552806614,176.9619850259));
#91684=CARTESIAN_POINT('Ctrl Pts',(-176.014168613314,54.3999999999999,176.961985025928));
#91685=CARTESIAN_POINT('Ctrl Pts',(-177.597158086212,54.8500380311261,174.763125936056));
#91686=CARTESIAN_POINT('Ctrl Pts',(-177.815415056901,54.7134552807034,174.943121919234));
#91687=CARTESIAN_POINT('Ctrl Pts',(-177.815415056962,54.4000000000186,174.943121919277));
#91688=CARTESIAN_POINT('Ctrl Pts',(-179.542670640116,54.8500380311121,172.013651556169));
#91689=CARTESIAN_POINT('Ctrl Pts',(-179.77599160756,54.7134552806729,172.172358510286));
#91690=CARTESIAN_POINT('Ctrl Pts',(-179.775991607544,54.3999999999953,172.172358510275));
#91691=CARTESIAN_POINT('Ctrl Pts',(-179.917528256893,54.8500380311093,171.451529957781));
#91692=CARTESIAN_POINT('Ctrl Pts',(-180.153696573202,54.7134552806667,171.605961658005));
#91693=CARTESIAN_POINT('Ctrl Pts',(-180.153696573215,54.3999999999906,171.605961658013));
#91694=CARTESIAN_POINT('Ctrl Pts',(-180.639398332045,54.8500380311206,170.303458800956));
#91695=CARTESIAN_POINT('Ctrl Pts',(-180.880916991954,54.7134552806913,170.449381248078));
#91696=CARTESIAN_POINT('Ctrl Pts',(-180.880916991941,54.4000000000093,170.44938124807));
#91697=CARTESIAN_POINT('Ctrl Pts',(-180.986399307621,54.8500380311124,169.717266069453));
#91698=CARTESIAN_POINT('Ctrl Pts',(-181.230420402746,54.7134552806726,169.858953973863));
#91699=CARTESIAN_POINT('Ctrl Pts',(-181.23042040281,54.3999999999906,169.858953973898));
#91700=CARTESIAN_POINT('Ctrl Pts',(-181.975711664719,54.8500380311199,167.9456619586));
#91701=CARTESIAN_POINT('Ctrl Pts',(-182.22665413232,54.7134552806918,168.074955463978));
#91702=CARTESIAN_POINT('Ctrl Pts',(-182.226654132192,54.4000000000186,168.074955463907));
#91703=CARTESIAN_POINT('Ctrl Pts',(-182.571021240997,54.8500380311088,166.740262383191));
#91704=CARTESIAN_POINT('Ctrl Pts',(-182.82582979671,54.7134552806674,166.861660004074));
#91705=CARTESIAN_POINT('Ctrl Pts',(-182.825829796822,54.4,166.861660004124));
#91706=CARTESIAN_POINT('Ctrl Pts',(-184.195262100537,54.8500380311274,163.063230859887));
#91707=CARTESIAN_POINT('Ctrl Pts',(-184.459874896115,54.7134552807022,163.162433189046));
#91708=CARTESIAN_POINT('Ctrl Pts',(-184.459874895891,54.4,163.162433188947));
#91709=CARTESIAN_POINT('Ctrl Pts',(-185.063862954418,54.8500380311274,160.531319247725));
#91710=CARTESIAN_POINT('Ctrl Pts',(-185.332658084472,54.7134552807023,160.617765878873));
#91711=CARTESIAN_POINT('Ctrl Pts',(-185.332658084675,54.4,160.61776587893));
#91712=CARTESIAN_POINT('Ctrl Pts',(-186.144761446821,54.8500380311087,156.650466794253));
#91713=CARTESIAN_POINT('Ctrl Pts',(-186.418046815866,54.7134552806674,156.720791693642));
#91714=CARTESIAN_POINT('Ctrl Pts',(-186.418046815765,54.4,156.720791693614));
#91715=CARTESIAN_POINT('Ctrl Pts',(-186.468386489537,54.850038031115,155.339660109173));
#91716=CARTESIAN_POINT('Ctrl Pts',(-186.74286676442,54.713455280679,155.405086705287));
#91717=CARTESIAN_POINT('Ctrl Pts',(-186.742866764511,54.4,155.405086705307));
#91718=CARTESIAN_POINT('Ctrl Pts',(-187.049982169092,54.850038031115,152.712642453476));
#91719=CARTESIAN_POINT('Ctrl Pts',(-187.326429131924,54.713455280679,152.769185688956));
#91720=CARTESIAN_POINT('Ctrl Pts',(-187.326429131834,54.4,152.769185688935));
#91721=CARTESIAN_POINT('Ctrl Pts',(-187.308038547416,54.8500380311205,151.397194165868));
#91722=CARTESIAN_POINT('Ctrl Pts',(-187.585258126222,54.7134552806912,151.449750314456));
#91723=CARTESIAN_POINT('Ctrl Pts',(-187.585258126313,54.4000000000092,151.449750314472));
#91724=CARTESIAN_POINT('Ctrl Pts',(-188.003945663939,54.8500380311037,147.446229609717));
#91725=CARTESIAN_POINT('Ctrl Pts',(-188.283075769649,54.7134552806547,147.48793887317));
#91726=CARTESIAN_POINT('Ctrl Pts',(-188.283075769467,54.3999999999814,147.487938873137));
#91727=CARTESIAN_POINT('Ctrl Pts',(-188.364534771007,54.8500380311496,144.806152648602));
#91728=CARTESIAN_POINT('Ctrl Pts',(-188.644410165692,54.7134552807506,144.842102846923));
#91729=CARTESIAN_POINT('Ctrl Pts',(-188.644410165763,54.4000000000368,144.842102846931));
#91730=CARTESIAN_POINT('Ctrl Pts',(-188.952047186871,54.8500380310803,139.518111180135));
#91731=CARTESIAN_POINT('Ctrl Pts',(-189.232988329538,54.7134552806075,139.544468866608));
#91732=CARTESIAN_POINT('Ctrl Pts',(-189.232988329467,54.3999999999631,139.5444688666));
#91733=CARTESIAN_POINT('Ctrl Pts',(-189.1784582655,54.8500380311149,136.870114362724));
#91734=CARTESIAN_POINT('Ctrl Pts',(-189.459709168722,54.713455280679,136.892642646065));
#91735=CARTESIAN_POINT('Ctrl Pts',(-189.45970916872,54.3999999999999,136.892642646065));
#91736=CARTESIAN_POINT('Ctrl Pts',(-189.542662973237,54.8500380311149,131.568886534478));
#91737=CARTESIAN_POINT('Ctrl Pts',(-189.824352296183,54.713455280679,131.585033344381));
#91738=CARTESIAN_POINT('Ctrl Pts',(-189.824352296185,54.3999999999999,131.585033344381));
#91739=CARTESIAN_POINT('Ctrl Pts',(-189.680191107803,54.8500380311248,128.915639981583));
#91740=CARTESIAN_POINT('Ctrl Pts',(-189.962004740436,54.7134552807043,128.92923846097));
#91741=CARTESIAN_POINT('Ctrl Pts',(-189.962004740445,54.4000000000368,128.929238460971));
#91742=CARTESIAN_POINT('Ctrl Pts',(-189.896513954462,54.8500380311051,123.605692278856));
#91743=CARTESIAN_POINT('Ctrl Pts',(-190.178499841913,54.7134552806537,123.615062522318));
#91744=CARTESIAN_POINT('Ctrl Pts',(-190.178499841904,54.3999999999631,123.615062522317));
#91745=CARTESIAN_POINT('Ctrl Pts',(-189.975161211412,54.8500380311372,120.948982719434));
#91746=CARTESIAN_POINT('Ctrl Pts',(-190.25719326379,54.7134552807275,120.956675467201));
#91747=CARTESIAN_POINT('Ctrl Pts',(-190.257193263797,54.4000000000369,120.956675467189));
#91748=CARTESIAN_POINT('Ctrl Pts',(-190.15455552149,54.8500380310701,112.939682823118));
#91749=CARTESIAN_POINT('Ctrl Pts',(-190.436680384205,54.7134552805815,112.943231928075));
#91750=CARTESIAN_POINT('Ctrl Pts',(-190.436680384191,54.3999999999257,112.943231928098));
#91751=CARTESIAN_POINT('Ctrl Pts',(-190.19870833527,54.850038030788,107.58375287472));
#91752=CARTESIAN_POINT('Ctrl Pts',(-190.480836465935,54.7134552799851,107.58575000634));
#91753=CARTESIAN_POINT('Ctrl Pts',(-190.480836465829,54.399999999552,107.585750006322));
#91754=CARTESIAN_POINT('Ctrl Pts',(-190.218057935276,54.8500380311216,102.226659873173));
#91755=CARTESIAN_POINT('Ctrl Pts',(-190.500189698379,54.7134552806931,102.227676769414));
#91756=CARTESIAN_POINT('Ctrl Pts',(-190.500189698381,54.4000000000091,102.227676769414));
#91757=CARTESIAN_POINT('Ctrl Pts',(1.21569421196455E-14,54.4,196.));
#91758=CARTESIAN_POINT('Ctrl Pts',(-10.7117531408873,54.4,196.));
#91759=CARTESIAN_POINT('Ctrl Pts',(-21.4235888453071,54.3999999999959,196.014918521175));
#91760=CARTESIAN_POINT('Ctrl Pts',(-32.1353671216415,54.4000000000734,196.019441470522));
#91761=CARTESIAN_POINT('Ctrl Pts',(-37.9435801512012,54.4000000001154,196.021893934778));
#91762=CARTESIAN_POINT('Ctrl Pts',(-43.7517791269623,54.4000000000876,196.021820074024));
#91763=CARTESIAN_POINT('Ctrl Pts',(-49.5599150077629,54.4000000000594,196.01034215732));
#91764=CARTESIAN_POINT('Ctrl Pts',(-54.4646195038332,54.4000000000355,196.000649582831));
#91765=CARTESIAN_POINT('Ctrl Pts',(-59.3692789259093,54.4000000000106,195.982824723479));
#91766=CARTESIAN_POINT('Ctrl Pts',(-64.2738634995991,54.400000000024,195.951525205213));
#91767=CARTESIAN_POINT('Ctrl Pts',(-69.6310359293998,54.4000000000387,195.917337413403));
#91768=CARTESIAN_POINT('Ctrl Pts',(-74.9881325496737,54.4,195.866500385808));
#91769=CARTESIAN_POINT('Ctrl Pts',(-80.3450312167437,54.4,195.785694345575));
#91770=CARTESIAN_POINT('Ctrl Pts',(-82.3276232645959,54.4,195.755787971991));
#91771=CARTESIAN_POINT('Ctrl Pts',(-84.3102773500987,54.4,195.721822553936));
#91772=CARTESIAN_POINT('Ctrl Pts',(-86.2928923209843,54.4,195.682687093389));
#91773=CARTESIAN_POINT('Ctrl Pts',(-89.6683134019806,54.4,195.616058594925));
#91774=CARTESIAN_POINT('Ctrl Pts',(-93.0436188031098,54.4,195.534443957971));
#91775=CARTESIAN_POINT('Ctrl Pts',(-96.4182977668297,54.4,195.432367934214));
#91776=CARTESIAN_POINT('Ctrl Pts',(-99.0028841103095,54.4,195.354190335743));
#91777=CARTESIAN_POINT('Ctrl Pts',(-101.586508773315,54.4,195.264201579288));
#91778=CARTESIAN_POINT('Ctrl Pts',(-104.168823808363,54.4000000000002,195.158121528418));
#91779=CARTESIAN_POINT('Ctrl Pts',(-106.940491118349,54.4000000000004,195.044262992474));
#91780=CARTESIAN_POINT('Ctrl Pts',(-109.71064886288,54.400000000001,194.911866455551));
#91781=CARTESIAN_POINT('Ctrl Pts',(-112.478864925773,54.400000000002,194.755651977743));
#91782=CARTESIAN_POINT('Ctrl Pts',(-114.594746353043,54.4000000000029,194.636249696723));
#91783=CARTESIAN_POINT('Ctrl Pts',(-116.709517996796,54.399999999997,194.503228627145));
#91784=CARTESIAN_POINT('Ctrl Pts',(-118.822814021222,54.3999999999952,194.352073476874));
#91785=CARTESIAN_POINT('Ctrl Pts',(-121.558134924859,54.3999999999929,194.156427510834));
#91786=CARTESIAN_POINT('Ctrl Pts',(-124.290982134953,54.3999999999953,193.93039917945));
#91787=CARTESIAN_POINT('Ctrl Pts',(-127.020559030863,54.400000000018,193.664236790067));
#91788=CARTESIAN_POINT('Ctrl Pts',(-127.515038935979,54.4000000000221,193.616019810635));
#91789=CARTESIAN_POINT('Ctrl Pts',(-128.009411525647,54.4000000000268,193.56648586568));
#91790=CARTESIAN_POINT('Ctrl Pts',(-128.503672075522,54.4000000000323,193.515577171767));
#91791=CARTESIAN_POINT('Ctrl Pts',(-130.44030260628,54.400000000054,193.316104786329));
#91792=CARTESIAN_POINT('Ctrl Pts',(-132.375187111056,54.4000000000251,193.095177265629));
#91793=CARTESIAN_POINT('Ctrl Pts',(-134.307827469057,54.4000000000103,192.846712461554));
#91794=CARTESIAN_POINT('Ctrl Pts',(-135.037156465656,54.4000000000048,192.752948205056));
#91795=CARTESIAN_POINT('Ctrl Pts',(-135.766166053061,54.4000000000007,192.655262645524));
#91796=CARTESIAN_POINT('Ctrl Pts',(-136.494829730514,54.4000000000009,192.553330224408));
#91797=CARTESIAN_POINT('Ctrl Pts',(-136.887919442628,54.400000000001,192.498341088389));
#91798=CARTESIAN_POINT('Ctrl Pts',(-137.28091003026,54.4000000000004,192.442107475666));
#91799=CARTESIAN_POINT('Ctrl Pts',(-137.6737996963,54.3999999999999,192.384558370491));
#91800=CARTESIAN_POINT('Ctrl Pts',(-138.610834530866,54.3999999999985,192.247304782757));
#91801=CARTESIAN_POINT('Ctrl Pts',(-139.547276781443,54.399999999997,192.102570241843));
#91802=CARTESIAN_POINT('Ctrl Pts',(-140.482938496475,54.4000000000026,191.949421722643));
#91803=CARTESIAN_POINT('Ctrl Pts',(-140.735750537609,54.4000000000041,191.908041607251));
#91804=CARTESIAN_POINT('Ctrl Pts',(-140.988534786983,54.4000000000047,191.866041232653));
#91805=CARTESIAN_POINT('Ctrl Pts',(-141.241276754107,54.400000000005,191.823400409481));
#91806=CARTESIAN_POINT('Ctrl Pts',(-142.316874391013,54.4000000000064,191.641933242939));
#91807=CARTESIAN_POINT('Ctrl Pts',(-143.391615355187,54.4000000000011,191.448879234487));
#91808=CARTESIAN_POINT('Ctrl Pts',(-144.462423620222,54.4000000000009,191.243014958559));
#91809=CARTESIAN_POINT('Ctrl Pts',(-144.849418259427,54.4000000000009,191.168614737913));
#91810=CARTESIAN_POINT('Ctrl Pts',(-145.235966560611,54.4000000000015,191.092555288149));
#91811=CARTESIAN_POINT('Ctrl Pts',(-145.622053844564,54.4000000000027,191.01472687048));
#91812=CARTESIAN_POINT('Ctrl Pts',(-147.026899899536,54.4000000000068,190.731534571558));
#91813=CARTESIAN_POINT('Ctrl Pts',(-148.425594625321,54.4000000000174,190.424926443793));
#91814=CARTESIAN_POINT('Ctrl Pts',(-149.816784865909,54.4000000000188,190.089768382214));
#91815=CARTESIAN_POINT('Ctrl Pts',(-150.659099159149,54.4000000000197,189.886842558322));
#91816=CARTESIAN_POINT('Ctrl Pts',(-151.498662621968,54.4000000000172,189.67345160904));
#91817=CARTESIAN_POINT('Ctrl Pts',(-152.33517708753,54.4000000000079,189.448465183433));
#91818=CARTESIAN_POINT('Ctrl Pts',(-152.632968467816,54.4000000000046,189.368372105566));
#91819=CARTESIAN_POINT('Ctrl Pts',(-152.930371223218,54.4000000000044,189.286797587327));
#91820=CARTESIAN_POINT('Ctrl Pts',(-153.227373996649,54.4000000000046,189.203666695846));
#91821=CARTESIAN_POINT('Ctrl Pts',(-154.162302082574,54.4000000000055,188.941980906329));
#91822=CARTESIAN_POINT('Ctrl Pts',(-155.093230768218,54.4000000000157,188.664878378805));
#91823=CARTESIAN_POINT('Ctrl Pts',(-156.019362358089,54.4000000000085,188.370172325145));
#91824=CARTESIAN_POINT('Ctrl Pts',(-156.084148131243,54.400000000008,188.34955672392));
#91825=CARTESIAN_POINT('Ctrl Pts',(-156.148910435088,54.4000000000074,188.328855001875));
#91826=CARTESIAN_POINT('Ctrl Pts',(-156.213648998875,54.4000000000067,188.308066420174));
#91827=CARTESIAN_POINT('Ctrl Pts',(-156.416564746016,54.4000000000046,188.24290694889));
#91828=CARTESIAN_POINT('Ctrl Pts',(-156.619277410847,54.4000000000042,188.176883120644));
#91829=CARTESIAN_POINT('Ctrl Pts',(-156.821789356633,54.4000000000037,188.109962015202));
#91830=CARTESIAN_POINT('Ctrl Pts',(-157.674439769922,54.4000000000014,187.828199336995));
#91831=CARTESIAN_POINT('Ctrl Pts',(-158.523442546846,54.4000000000024,187.530554236109));
#91832=CARTESIAN_POINT('Ctrl Pts',(-159.366711682169,54.4000000000019,187.215315777277));
#91833=CARTESIAN_POINT('Ctrl Pts',(-159.592281282814,54.4000000000018,187.130991318705));
#91834=CARTESIAN_POINT('Ctrl Pts',(-159.817440728344,54.4000000000015,187.045408262957));
#91835=CARTESIAN_POINT('Ctrl Pts',(-160.042150350673,54.4000000000011,186.958534466439));
#91836=CARTESIAN_POINT('Ctrl Pts',(-160.341043440676,54.4000000000005,186.842980992527));
#91837=CARTESIAN_POINT('Ctrl Pts',(-160.638745192439,54.4000000000012,186.725316022465));
#91838=CARTESIAN_POINT('Ctrl Pts',(-160.935217131209,54.400000000002,186.605440002852));
#91839=CARTESIAN_POINT('Ctrl Pts',(-162.043912972633,54.4000000000049,186.157147847507));
#91840=CARTESIAN_POINT('Ctrl Pts',(-163.135358589241,54.4000000000127,185.677949049057));
#91841=CARTESIAN_POINT('Ctrl Pts',(-164.206821641103,54.400000000017,185.162953209131));
#91842=CARTESIAN_POINT('Ctrl Pts',(-165.213812221236,54.400000000021,184.678945889688));
#91843=CARTESIAN_POINT('Ctrl Pts',(-166.203152821026,54.4000000000218,184.163320161186));
#91844=CARTESIAN_POINT('Ctrl Pts',(-167.172599949771,54.4000000000122,183.612061884605));
#91845=CARTESIAN_POINT('Ctrl Pts',(-167.234668705759,54.4000000000116,183.57676762828));
#91846=CARTESIAN_POINT('Ctrl Pts',(-167.296655923169,54.400000000011,183.541327323102));
#91847=CARTESIAN_POINT('Ctrl Pts',(-167.358561016714,54.4000000000103,183.505739922036));
#91848=CARTESIAN_POINT('Ctrl Pts',(-168.394803639309,54.3999999999987,182.910034791816));
#91849=CARTESIAN_POINT('Ctrl Pts',(-169.40790447556,54.4000000000016,182.27289323376));
#91850=CARTESIAN_POINT('Ctrl Pts',(-170.394537845123,54.4000000000013,181.588333408786));
#91851=CARTESIAN_POINT('Ctrl Pts',(-170.521200139063,54.4000000000013,181.500450796617));
#91852=CARTESIAN_POINT('Ctrl Pts',(-170.64742620343,54.4000000000013,181.411786725557));
#91853=CARTESIAN_POINT('Ctrl Pts',(-170.77320899952,54.4000000000012,181.322328563752));
#91854=CARTESIAN_POINT('Ctrl Pts',(-170.892813071244,54.4000000000011,181.237264781316));
#91855=CARTESIAN_POINT('Ctrl Pts',(-171.012017675547,54.4000000000009,181.151481008562));
#91856=CARTESIAN_POINT('Ctrl Pts',(-171.130802550739,54.4000000000005,181.064975846037));
#91857=CARTESIAN_POINT('Ctrl Pts',(-171.508826188153,54.3999999999992,180.789679886513));
#91858=CARTESIAN_POINT('Ctrl Pts',(-171.88264292564,54.3999999999966,180.50705177373));
#91859=CARTESIAN_POINT('Ctrl Pts',(-172.252308598498,54.4000000000004,180.216507814835));
#91860=CARTESIAN_POINT('Ctrl Pts',(-172.303960379812,54.4000000000009,180.175911367481));
#91861=CARTESIAN_POINT('Ctrl Pts',(-172.355531079046,54.4000000000015,180.135160303721));
#91862=CARTESIAN_POINT('Ctrl Pts',(-172.407020808966,54.4000000000023,180.094252958564));
#91863=CARTESIAN_POINT('Ctrl Pts',(-172.455054775837,54.400000000003,180.056091133574));
#91864=CARTESIAN_POINT('Ctrl Pts',(-172.50300769104,54.4000000000036,180.017800247102));
#91865=CARTESIAN_POINT('Ctrl Pts',(-172.550875974858,54.400000000004,179.979382823007));
#91866=CARTESIAN_POINT('Ctrl Pts',(-172.597530076281,54.4000000000044,179.941939859584));
#91867=CARTESIAN_POINT('Ctrl Pts',(-172.644097658006,54.4000000000046,179.904381602988));
#91868=CARTESIAN_POINT('Ctrl Pts',(-172.690571407175,54.4000000000048,179.866713791186));
#91869=CARTESIAN_POINT('Ctrl Pts',(-173.036090107705,54.4000000000061,179.586664653374));
#91870=CARTESIAN_POINT('Ctrl Pts',(-173.376498345685,54.4000000000024,179.300504241468));
#91871=CARTESIAN_POINT('Ctrl Pts',(-173.710509910594,54.4000000000008,179.009174034974));
#91872=CARTESIAN_POINT('Ctrl Pts',(-173.799924385604,54.4000000000004,178.931185305825));
#91873=CARTESIAN_POINT('Ctrl Pts',(-173.888880293489,54.4000000000001,178.852825858204));
#91874=CARTESIAN_POINT('Ctrl Pts',(-173.977352529316,54.4000000000001,178.77411328332));
#91875=CARTESIAN_POINT('Ctrl Pts',(-174.086885484671,54.4000000000001,178.676663265581));
#91876=CARTESIAN_POINT('Ctrl Pts',(-174.195746819395,54.4000000000001,178.578606690771));
#91877=CARTESIAN_POINT('Ctrl Pts',(-174.303919113315,54.4000000000002,178.479960989208));
#91878=CARTESIAN_POINT('Ctrl Pts',(-174.95858512167,54.4000000000008,177.882950559419));
#91879=CARTESIAN_POINT('Ctrl Pts',(-175.588161594654,54.400000000003,177.264237376583));
#91880=CARTESIAN_POINT('Ctrl Pts',(-176.192889081029,54.4000000000052,176.624027636066));
#91881=CARTESIAN_POINT('Ctrl Pts',(-176.801495076758,54.4000000000073,175.9797118155));
#91882=CARTESIAN_POINT('Ctrl Pts',(-177.384932334614,54.4000000000094,175.313622763741));
#91883=CARTESIAN_POINT('Ctrl Pts',(-177.943406073387,54.4000000000095,174.625935886316));
#91884=CARTESIAN_POINT('Ctrl Pts',(-178.443543971493,54.4000000000097,174.01008191584));
#91885=CARTESIAN_POINT('Ctrl Pts',(-178.923660601104,54.4000000000082,173.376906001319));
#91886=CARTESIAN_POINT('Ctrl Pts',(-179.383876297428,54.400000000004,172.726511192075));
#91887=CARTESIAN_POINT('Ctrl Pts',(-179.775881961457,54.4000000000004,172.172513466411));
#91888=CARTESIAN_POINT('Ctrl Pts',(-180.153586615473,54.3999999999974,171.606136536174));
#91889=CARTESIAN_POINT('Ctrl Pts',(-180.517306782578,54.4000000000037,171.027671453041));
#91890=CARTESIAN_POINT('Ctrl Pts',(-180.773257799144,54.4000000000081,170.620603768963));
#91891=CARTESIAN_POINT('Ctrl Pts',(-181.022282062403,54.4000000000033,170.207421858588));
#91892=CARTESIAN_POINT('Ctrl Pts',(-181.263216116216,54.4000000000031,169.790864332171));
#91893=CARTESIAN_POINT('Ctrl Pts',(-181.364433682584,54.400000000003,169.615866491854));
#91894=CARTESIAN_POINT('Ctrl Pts',(-181.464223290182,54.4000000000036,169.440273105744));
#91895=CARTESIAN_POINT('Ctrl Pts',(-181.562498312604,54.4000000000056,169.264287803901));
#91896=CARTESIAN_POINT('Ctrl Pts',(-181.963797855854,54.4000000000141,168.545663483017));
#91897=CARTESIAN_POINT('Ctrl Pts',(-182.341570248312,54.4000000000098,167.817937559455));
#91898=CARTESIAN_POINT('Ctrl Pts',(-182.698076436423,54.4000000000056,167.081983790314));
#91899=CARTESIAN_POINT('Ctrl Pts',(-182.931095611984,54.4000000000029,166.600950511637));
#91900=CARTESIAN_POINT('Ctrl Pts',(-183.155029566892,54.4,166.116402350166));
#91901=CARTESIAN_POINT('Ctrl Pts',(-183.370511496512,54.4,165.628584399065));
#91902=CARTESIAN_POINT('Ctrl Pts',(-183.755753296777,54.4,164.756456207084));
#91903=CARTESIAN_POINT('Ctrl Pts',(-184.114155896939,54.4,163.873944120111));
#91904=CARTESIAN_POINT('Ctrl Pts',(-184.448595887359,54.4,162.982161533304));
#91905=CARTESIAN_POINT('Ctrl Pts',(-184.791126771316,54.4,162.06880461874));
#91906=CARTESIAN_POINT('Ctrl Pts',(-185.10852159876,54.4,161.145723295192));
#91907=CARTESIAN_POINT('Ctrl Pts',(-185.403901993162,54.4,160.214125497789));
#91908=CARTESIAN_POINT('Ctrl Pts',(-185.613942467716,54.4,159.551680571965));
#91909=CARTESIAN_POINT('Ctrl Pts',(-185.812852196925,54.4,158.884929610429));
#91910=CARTESIAN_POINT('Ctrl Pts',(-186.001762645606,54.4,158.214310293893));
#91911=CARTESIAN_POINT('Ctrl Pts',(-186.020018321289,54.4,158.149503879878));
#91912=CARTESIAN_POINT('Ctrl Pts',(-186.038180629918,54.4,158.084661317201));
#91913=CARTESIAN_POINT('Ctrl Pts',(-186.056250572068,54.4,158.019783088719));
#91914=CARTESIAN_POINT('Ctrl Pts',(-186.248767714115,54.4,157.328570520082));
#91915=CARTESIAN_POINT('Ctrl Pts',(-186.430890122847,54.4,156.632354201029));
#91916=CARTESIAN_POINT('Ctrl Pts',(-186.603184662211,54.4,155.933322726759));
#91917=CARTESIAN_POINT('Ctrl Pts',(-186.726566778214,54.4,155.432738188409));
#91918=CARTESIAN_POINT('Ctrl Pts',(-186.844909102226,54.4,154.930710225721));
#91919=CARTESIAN_POINT('Ctrl Pts',(-186.958421160883,54.4,154.42804577865));
#91920=CARTESIAN_POINT('Ctrl Pts',(-186.98407601225,54.4,154.314438626865));
#91921=CARTESIAN_POINT('Ctrl Pts',(-187.009484169709,54.4,154.200798819904));
#91922=CARTESIAN_POINT('Ctrl Pts',(-187.034647948172,54.4,154.087136197121));
#91923=CARTESIAN_POINT('Ctrl Pts',(-187.249235148189,54.4,153.117864272993));
#91924=CARTESIAN_POINT('Ctrl Pts',(-187.446091441865,54.400000000005,152.147366918553));
#91925=CARTESIAN_POINT('Ctrl Pts',(-187.627848434952,54.4000000000063,151.175803321643));
#91926=CARTESIAN_POINT('Ctrl Pts',(-187.693091593958,54.4000000000068,150.827052623469));
#91927=CARTESIAN_POINT('Ctrl Pts',(-187.756389401055,54.4000000000069,150.478164329375));
#91928=CARTESIAN_POINT('Ctrl Pts',(-187.817864007364,54.4000000000059,150.129146500694));
#91929=CARTESIAN_POINT('Ctrl Pts',(-188.06963015802,54.4000000000017,148.699761580444));
#91930=CARTESIAN_POINT('Ctrl Pts',(-188.291104422212,54.4000000000111,147.268244123339));
#91931=CARTESIAN_POINT('Ctrl Pts',(-188.488029538762,54.4000000000176,145.834998333236));
#91932=CARTESIAN_POINT('Ctrl Pts',(-188.65465881123,54.400000000023,144.622249510451));
#91933=CARTESIAN_POINT('Ctrl Pts',(-188.803712723298,54.400000000027,143.408263309562));
#91934=CARTESIAN_POINT('Ctrl Pts',(-188.938699247615,54.4000000000176,142.193285856766));
#91935=CARTESIAN_POINT('Ctrl Pts',(-189.136760811129,54.4000000000038,140.410586915872));
#91936=CARTESIAN_POINT('Ctrl Pts',(-189.30429973454,54.4000000000006,138.625739732878));
#91937=CARTESIAN_POINT('Ctrl Pts',(-189.448306971578,54.4000000000001,136.839235864604));
#91938=CARTESIAN_POINT('Ctrl Pts',(-189.518148388495,54.3999999999998,135.972807454108));
#91939=CARTESIAN_POINT('Ctrl Pts',(-189.582455734489,54.4000000000004,135.105989435971));
#91940=CARTESIAN_POINT('Ctrl Pts',(-189.642030732453,54.4000000000003,134.238837995223));
#91941=CARTESIAN_POINT('Ctrl Pts',(-189.792507883552,54.4,132.048548732355));
#91942=CARTESIAN_POINT('Ctrl Pts',(-189.912606434434,54.4000000000252,129.856120468085));
#91943=CARTESIAN_POINT('Ctrl Pts',(-190.010855951794,54.4000000000233,127.662154066557));
#91944=CARTESIAN_POINT('Ctrl Pts',(-190.031601867449,54.4000000000229,127.198886224246));
#91945=CARTESIAN_POINT('Ctrl Pts',(-190.051373788504,54.4000000000214,126.735549820195));
#91946=CARTESIAN_POINT('Ctrl Pts',(-190.070252291175,54.4000000000179,126.272150491644));
#91947=CARTESIAN_POINT('Ctrl Pts',(-190.155978565131,54.4000000000021,124.167878850857));
#91948=CARTESIAN_POINT('Ctrl Pts',(-190.223187321394,54.4000000000231,122.062303121466));
#91949=CARTESIAN_POINT('Ctrl Pts',(-190.277034909484,54.4000000000263,119.95578683131));
#91950=CARTESIAN_POINT('Ctrl Pts',(-190.291163394482,54.4000000000271,119.403080853939));
#91951=CARTESIAN_POINT('Ctrl Pts',(-190.3043721644,54.4000000000267,118.850310089037));
#91952=CARTESIAN_POINT('Ctrl Pts',(-190.316754563799,54.4000000000241,118.297481238444));
#91953=CARTESIAN_POINT('Ctrl Pts',(-190.397155294802,54.4000000000074,114.707882625582));
#91954=CARTESIAN_POINT('Ctrl Pts',(-190.443516400857,54.4000000000024,111.11588653346));
#91955=CARTESIAN_POINT('Ctrl Pts',(-190.471166976935,54.4000000000008,107.522573212351));
#91956=CARTESIAN_POINT('Ctrl Pts',(-190.484470217798,54.4,105.793758866144));
#91957=CARTESIAN_POINT('Ctrl Pts',(-190.49344330146,54.4,104.064639655677));
#91958=CARTESIAN_POINT('Ctrl Pts',(-190.499797482064,54.4,102.335336081498));
#91959=CARTESIAN_POINT('Origin',(-189.5,59.,41.));
#91960=CARTESIAN_POINT('',(-190.5,51.8013867006572,41.));
#91961=CARTESIAN_POINT('',(-190.5,51.8013867006572,41.));
#91962=CARTESIAN_POINT('',(-189.5,51.8013867006572,40.));
#91963=CARTESIAN_POINT('',(-189.5,54.9,40.));
#91964=CARTESIAN_POINT('Origin',(-189.5,51.8013867006572,41.));
#91965=CARTESIAN_POINT('Ctrl Pts',(7.71069817591099E-15,-3.96262874552467,
41.));
#91966=CARTESIAN_POINT('Ctrl Pts',(7.71069817591099E-15,-3.96262874552467,
40.));
#91967=CARTESIAN_POINT('Ctrl Pts',(7.58040827681699E-15,-2.96262874552467,
40.));
#91968=CARTESIAN_POINT('Ctrl Pts',(-8.85050807869572,-3.96262874552467,
41.));
#91969=CARTESIAN_POINT('Ctrl Pts',(-8.85050807869562,-3.96262874563983,
40.));
#91970=CARTESIAN_POINT('Ctrl Pts',(-8.85149033058515,-2.96262874562831,
40.));
#91971=CARTESIAN_POINT('Ctrl Pts',(-17.7049033029141,-3.9725981542643,41.));
#91972=CARTESIAN_POINT('Ctrl Pts',(-17.7049033029142,-3.97259815428753,
40.));
#91973=CARTESIAN_POINT('Ctrl Pts',(-17.7032012684101,-2.97258723674239,
40.));
#91974=CARTESIAN_POINT('Ctrl Pts',(-35.4141298351867,-3.85438528439772,
41.));
#91975=CARTESIAN_POINT('Ctrl Pts',(-35.4141298351865,-3.85438528437448,
40.));
#91976=CARTESIAN_POINT('Ctrl Pts',(-35.4024817399098,-2.85444075890724,
40.));
#91977=CARTESIAN_POINT('Ctrl Pts',(-44.2690343362197,-3.7290091962045,41.));
#91978=CARTESIAN_POINT('Ctrl Pts',(-44.2690343362206,-3.72900919623712,
40.));
#91979=CARTESIAN_POINT('Ctrl Pts',(-44.2500950804588,-2.72914237565843,
40.));
#91980=CARTESIAN_POINT('Ctrl Pts',(-61.975684001311,-3.22335878785305,41.));
#91981=CARTESIAN_POINT('Ctrl Pts',(-61.9756840013101,-3.22335878782043,
40.));
#91982=CARTESIAN_POINT('Ctrl Pts',(-61.9375323490691,-2.22404061740319,
40.));
#91983=CARTESIAN_POINT('Ctrl Pts',(-70.8274773375622,-2.8447952216319,41.));
#91984=CARTESIAN_POINT('Ctrl Pts',(-70.8274773375648,-2.84479522167177,
40.));
#91985=CARTESIAN_POINT('Ctrl Pts',(-70.7774082065636,-1.84593393742596,
40.));
#91986=CARTESIAN_POINT('Ctrl Pts',(-84.1008785865341,-1.97714572979944,
41.));
#91987=CARTESIAN_POINT('Ctrl Pts',(-84.1008785865328,-1.97714572977952,
40.));
#91988=CARTESIAN_POINT('Ctrl Pts',(-84.0280706662548,-0.979770824085102,
40.));
#91989=CARTESIAN_POINT('Ctrl Pts',(-88.5246348023096,-1.63762966081861,
41.));
#91990=CARTESIAN_POINT('Ctrl Pts',(-88.5246348023124,-1.63762966084928,
40.0000000000001));
#91991=CARTESIAN_POINT('Ctrl Pts',(-88.4434228779164,-0.640887452776137,
40.0000000000001));
#91992=CARTESIAN_POINT('Ctrl Pts',(-97.3704217853518,-0.832166707467492,
41.));
#91993=CARTESIAN_POINT('Ctrl Pts',(-97.370421785349,-0.832166707436793,
40.0000000000001));
#91994=CARTESIAN_POINT('Ctrl Pts',(-97.2702717928855,0.162851073824349,
40.0000000000001));
#91995=CARTESIAN_POINT('Ctrl Pts',(-101.788182438523,-0.366638907835244,
41.));
#91996=CARTESIAN_POINT('Ctrl Pts',(-101.788182438527,-0.36663890786983,
40.));
#91997=CARTESIAN_POINT('Ctrl Pts',(-101.677510051103,0.627290636601703,
40.));
#91998=CARTESIAN_POINT('Ctrl Pts',(-110.595154903837,0.721257750102517,
41.));
#91999=CARTESIAN_POINT('Ctrl Pts',(-110.595154903833,0.721257750137102,
40.));
#92000=CARTESIAN_POINT('Ctrl Pts',(-110.460637374487,1.71224178179782,40.));
#92001=CARTESIAN_POINT('Ctrl Pts',(-114.986445334228,1.34357196524849,41.));
#92002=CARTESIAN_POINT('Ctrl Pts',(-114.986445334236,1.34357196519969,40.));
#92003=CARTESIAN_POINT('Ctrl Pts',(-114.838608995725,2.33270535868658,40.));
#92004=CARTESIAN_POINT('Ctrl Pts',(-123.73794201961,2.79063399912821,41.));
#92005=CARTESIAN_POINT('Ctrl Pts',(-123.737942019602,2.79063399917701,40.));
#92006=CARTESIAN_POINT('Ctrl Pts',(-123.559508040824,3.77470806565397,40.));
#92007=CARTESIAN_POINT('Ctrl Pts',(-128.098212002788,3.61490182217767,41.0000000001842));
#92008=CARTESIAN_POINT('Ctrl Pts',(-128.098212002812,3.61490182216112,40.0000000002763));
#92009=CARTESIAN_POINT('Ctrl Pts',(-127.902516032675,4.5957849159024,40.));
#92010=CARTESIAN_POINT('Ctrl Pts',(-134.607986242742,5.05437483435604,40.9999999999079));
#92011=CARTESIAN_POINT('Ctrl Pts',(-134.607986242731,5.05437483436432,39.9999999998619));
#92012=CARTESIAN_POINT('Ctrl Pts',(-134.381970283735,6.02855342450368,40.));
#92013=CARTESIAN_POINT('Ctrl Pts',(-136.772776373825,5.56826329016615,41.0000000000307));
#92014=CARTESIAN_POINT('Ctrl Pts',(-136.772776373836,5.56826329013963,40.0000000000461));
#92015=CARTESIAN_POINT('Ctrl Pts',(-136.535908314328,6.53988132256591,40.));
#92016=CARTESIAN_POINT('Ctrl Pts',(-141.090337531917,6.67665701106583,40.9999999999692));
#92017=CARTESIAN_POINT('Ctrl Pts',(-141.090337531907,6.67665701109232,39.9999999999538));
#92018=CARTESIAN_POINT('Ctrl Pts',(-140.829896351113,7.64222340961483,40.));
#92019=CARTESIAN_POINT('Ctrl Pts',(-143.245640919778,7.27188104593143,40.999999999815));
#92020=CARTESIAN_POINT('Ctrl Pts',(-143.245640919832,7.27188104576561,39.9999999997225));
#92021=CARTESIAN_POINT('Ctrl Pts',(-142.972463556223,8.23395393721191,40.));
#92022=CARTESIAN_POINT('Ctrl Pts',(-149.671568403027,9.19757481923777,41.00000000037));
#92023=CARTESIAN_POINT('Ctrl Pts',(-149.67156840292,9.19757481956941,40.000000000555));
#92024=CARTESIAN_POINT('Ctrl Pts',(-149.356734736723,10.1471643326025,40.));
#92025=CARTESIAN_POINT('Ctrl Pts',(-153.892282124603,10.6608124936544,41.));
#92026=CARTESIAN_POINT('Ctrl Pts',(-153.892282124687,10.660812493454,40.0000000000001));
#92027=CARTESIAN_POINT('Ctrl Pts',(-153.545256591485,11.5996387774958,40.0000000000001));
#92028=CARTESIAN_POINT('Ctrl Pts',(-160.084751714187,13.254997283011,41.));
#92029=CARTESIAN_POINT('Ctrl Pts',(-160.084751714145,13.2549972831112,40.0000000000001));
#92030=CARTESIAN_POINT('Ctrl Pts',(-159.678679400237,14.1690873519471,40.0000000000001));
#92031=CARTESIAN_POINT('Ctrl Pts',(-162.125908453503,14.187144173683,41.));
#92032=CARTESIAN_POINT('Ctrl Pts',(-162.125908453557,14.1871441735757,40.));
#92033=CARTESIAN_POINT('Ctrl Pts',(-161.69833306059,15.0915173718029,40.));
#92034=CARTESIAN_POINT('Ctrl Pts',(-166.147967957112,16.2216704183731,41.));
#92035=CARTESIAN_POINT('Ctrl Pts',(-166.147967957058,16.2216704184803,40.));
#92036=CARTESIAN_POINT('Ctrl Pts',(-165.672785207306,17.1019618206062,40.));
#92037=CARTESIAN_POINT('Ctrl Pts',(-168.107616958799,17.3133889676838,41.0000000000612));
#92038=CARTESIAN_POINT('Ctrl Pts',(-168.107616958864,17.3133889675427,40.0000000000764));
#92039=CARTESIAN_POINT('Ctrl Pts',(-167.606564886958,18.1794445808324,40.0000000000001));
#92040=CARTESIAN_POINT('Ctrl Pts',(-171.901224347846,19.6798162046833,40.9999999999389));
#92041=CARTESIAN_POINT('Ctrl Pts',(-171.901224347781,19.6798162048244,39.9999999999236));
#92042=CARTESIAN_POINT('Ctrl Pts',(-171.343751302672,20.5106767876529,40.0000000000001));
#92043=CARTESIAN_POINT('Ctrl Pts',(-173.735371451672,20.9542971278746,41.0000000000305));
#92044=CARTESIAN_POINT('Ctrl Pts',(-173.7353714518,20.9542971276705,40.0000000000305));
#92045=CARTESIAN_POINT('Ctrl Pts',(-173.147319647996,21.7642077357057,40.));
#92046=CARTESIAN_POINT('Ctrl Pts',(-177.244885717175,23.73437233231,40.9999999999695));
#92047=CARTESIAN_POINT('Ctrl Pts',(-177.244885717047,23.7343723325141,39.9999999999695));
#92048=CARTESIAN_POINT('Ctrl Pts',(-176.591062187867,24.4921816156992,40.));
#92049=CARTESIAN_POINT('Ctrl Pts',(-178.920625669167,25.2395538542272,40.9999999998762));
#92050=CARTESIAN_POINT('Ctrl Pts',(-178.920625669525,25.239553853915,39.9999999998375));
#92051=CARTESIAN_POINT('Ctrl Pts',(-178.231553296469,25.9661960735548,39.9999999999999));
#92052=CARTESIAN_POINT('Ctrl Pts',(-181.276582615106,27.724368039953,41.0000000000618));
#92053=CARTESIAN_POINT('Ctrl Pts',(-181.276582614927,27.724368040109,40.0000000000811));
#92054=CARTESIAN_POINT('Ctrl Pts',(-180.532610330637,28.3931076402081,39.9999999999999));
#92055=CARTESIAN_POINT('Ctrl Pts',(-182.038370134922,28.594995197168,41.000000000031));
#92056=CARTESIAN_POINT('Ctrl Pts',(-182.038370135018,28.5949951971027,40.0000000000465));
#92057=CARTESIAN_POINT('Ctrl Pts',(-181.275699297888,29.2424485691571,40.));
#92058=CARTESIAN_POINT('Ctrl Pts',(-183.470925423842,30.3865407544758,40.999999999969));
#92059=CARTESIAN_POINT('Ctrl Pts',(-183.470925423746,30.386540754541,39.9999999999534));
#92060=CARTESIAN_POINT('Ctrl Pts',(-182.671568980253,30.9881153143562,40.));
#92061=CARTESIAN_POINT('Ctrl Pts',(-184.144844526056,31.3102252938863,41.0000000000001));
#92062=CARTESIAN_POINT('Ctrl Pts',(-184.144844526143,31.3102252938285,40.0000000000001));
#92063=CARTESIAN_POINT('Ctrl Pts',(-183.327437398454,31.8871479480862,40.0000000000001));
#92064=CARTESIAN_POINT('Ctrl Pts',(-186.030824239729,34.1695586767068,41.0000000000001));
#92065=CARTESIAN_POINT('Ctrl Pts',(-186.030824239554,34.1695586768225,40.0000000000001));
#92066=CARTESIAN_POINT('Ctrl Pts',(-185.161335117964,34.6675198327877,40.0000000000001));
#92067=CARTESIAN_POINT('Ctrl Pts',(-187.108035248898,36.1953798490653,40.9999999997501));
#92068=CARTESIAN_POINT('Ctrl Pts',(-187.108035248771,36.1953798491075,39.999999999625));
#92069=CARTESIAN_POINT('Ctrl Pts',(-186.20661784616,36.6337883765426,40.));
#92070=CARTESIAN_POINT('Ctrl Pts',(-188.84587319312,40.4985477363864,41.00000000025));
#92071=CARTESIAN_POINT('Ctrl Pts',(-188.845873193246,40.4985477363443,40.0000000003749));
#92072=CARTESIAN_POINT('Ctrl Pts',(-187.89280993586,40.8090727718468,40.));
#92073=CARTESIAN_POINT('Ctrl Pts',(-189.476816493,42.70183971556,41.));
#92074=CARTESIAN_POINT('Ctrl Pts',(-189.476816492796,42.7018397155975,40.));
#92075=CARTESIAN_POINT('Ctrl Pts',(-188.505057255412,42.9465120076084,40.));
#92076=CARTESIAN_POINT('Ctrl Pts',(-190.097254322749,46.0714373593176,41.));
#92077=CARTESIAN_POINT('Ctrl Pts',(-190.09725432285,46.0714373592989,40.));
#92078=CARTESIAN_POINT('Ctrl Pts',(-189.107932516311,46.2207273442081,40.));
#92079=CARTESIAN_POINT('Ctrl Pts',(-190.249747513175,47.205433603925,41.));
#92080=CARTESIAN_POINT('Ctrl Pts',(-190.249747513114,47.2054336039303,40.));
#92081=CARTESIAN_POINT('Ctrl Pts',(-189.256273490598,47.3234827160453,40.));
#92082=CARTESIAN_POINT('Ctrl Pts',(-190.451241426909,49.4932627877844,41.));
#92083=CARTESIAN_POINT('Ctrl Pts',(-190.451241426969,49.4932627877791,40.));
#92084=CARTESIAN_POINT('Ctrl Pts',(-189.452427308737,49.5506786699904,40.));
#92085=CARTESIAN_POINT('Ctrl Pts',(-190.5,50.6495849457038,40.9999999998129));
#92086=CARTESIAN_POINT('Ctrl Pts',(-190.500000000406,50.6495849457076,39.9999999997193));
#92087=CARTESIAN_POINT('Ctrl Pts',(-189.500000000281,50.6775460919873,40.));
#92088=CARTESIAN_POINT('Ctrl Pts',(-190.5,51.8013867006572,41.));
#92089=CARTESIAN_POINT('Ctrl Pts',(-190.5,51.8013867006572,40.));
#92090=CARTESIAN_POINT('Ctrl Pts',(-189.5,51.8013867006572,40.));
#92091=CARTESIAN_POINT('',(7.58040827681699E-15,-2.96262874552467,40.));
#92092=CARTESIAN_POINT('',(7.71069817591099E-15,-3.96262874552467,41.));
#92093=CARTESIAN_POINT('Origin',(7.58040827681699E-15,-2.96262874552467,
41.));
#92094=CARTESIAN_POINT('Ctrl Pts',(-190.5,51.8013867006571,41.));
#92095=CARTESIAN_POINT('Ctrl Pts',(-190.5,51.1173208557555,40.9999999998888));
#92096=CARTESIAN_POINT('Ctrl Pts',(-190.482804508878,50.4323861127385,40.9999999999097));
#92097=CARTESIAN_POINT('Ctrl Pts',(-190.447827838384,49.749902987648,40.9999999999442));
#92098=CARTESIAN_POINT('Ctrl Pts',(-190.423824777408,49.2815426824526,40.9999999999678));
#92099=CARTESIAN_POINT('Ctrl Pts',(-190.391446880902,48.8143355445067,40.9999999999977));
#92100=CARTESIAN_POINT('Ctrl Pts',(-190.350494470042,48.3493481958547,40.9999999999965));
#92101=CARTESIAN_POINT('Ctrl Pts',(-190.291195016811,47.6760424012827,40.9999999999947));
#92102=CARTESIAN_POINT('Ctrl Pts',(-190.214000398395,47.0065391729747,40.9999999999964));
#92103=CARTESIAN_POINT('Ctrl Pts',(-190.11844385301,46.3409947367191,40.9999999999979));
#92104=CARTESIAN_POINT('Ctrl Pts',(-190.055206160698,45.9005487776227,40.999999999999));
#92105=CARTESIAN_POINT('Ctrl Pts',(-189.983926901072,45.4618373621409,41.0000000000006));
#92106=CARTESIAN_POINT('Ctrl Pts',(-189.904470540969,45.0249032275489,40.9999999999998));
#92107=CARTESIAN_POINT('Ctrl Pts',(-189.899822264666,44.9993421449489,40.9999999999998));
#92108=CARTESIAN_POINT('Ctrl Pts',(-189.89514599803,44.9737871160482,40.9999999999997));
#92109=CARTESIAN_POINT('Ctrl Pts',(-189.890441712832,44.9482381447317,40.9999999999996));
#92110=CARTESIAN_POINT('Ctrl Pts',(-189.738971319567,44.1256024900784,40.9999999999961));
#92111=CARTESIAN_POINT('Ctrl Pts',(-189.558451814601,43.309235270496,40.9999999999954));
#92112=CARTESIAN_POINT('Ctrl Pts',(-189.347911931431,42.4993478242337,40.9999999999948));
#92113=CARTESIAN_POINT('Ctrl Pts',(-189.165422479056,41.7973624600857,40.9999999999943));
#92114=CARTESIAN_POINT('Ctrl Pts',(-188.960378432237,41.1002453485348,40.9999999999939));
#92115=CARTESIAN_POINT('Ctrl Pts',(-188.732115344505,40.4081401060491,40.999999999992));
#92116=CARTESIAN_POINT('Ctrl Pts',(-188.617983800639,40.0620874848063,40.9999999999911));
#92117=CARTESIAN_POINT('Ctrl Pts',(-188.498047016744,39.7172879245513,40.9999999999898));
#92118=CARTESIAN_POINT('Ctrl Pts',(-188.3722189604,39.3737599806281,40.9999999999879));
#92119=CARTESIAN_POINT('Ctrl Pts',(-188.295438183618,39.1641378729073,40.9999999999868));
#92120=CARTESIAN_POINT('Ctrl Pts',(-188.216463758887,38.9549892582146,40.9999999999854));
#92121=CARTESIAN_POINT('Ctrl Pts',(-188.135275760166,38.7463184326317,40.9999999999838));
#92122=CARTESIAN_POINT('Ctrl Pts',(-188.101465942341,38.6594198428209,40.9999999999831));
#92123=CARTESIAN_POINT('Ctrl Pts',(-188.067273383454,38.5726068818537,40.9999999999828));
#92124=CARTESIAN_POINT('Ctrl Pts',(-188.032688393693,38.485859497833,40.99999999998));
#92125=CARTESIAN_POINT('Ctrl Pts',(-188.014221711024,38.4395406634451,40.9999999999785));
#92126=CARTESIAN_POINT('Ctrl Pts',(-187.99564365788,38.3932418618882,40.9999999999765));
#92127=CARTESIAN_POINT('Ctrl Pts',(-187.976954221009,38.3469637927259,40.9999999999739));
#92128=CARTESIAN_POINT('Ctrl Pts',(-187.868393712879,38.0781504123006,40.9999999999589));
#92129=CARTESIAN_POINT('Ctrl Pts',(-187.7565374796,37.8111930698997,40.9999999999416));
#92130=CARTESIAN_POINT('Ctrl Pts',(-187.641486166773,37.5461991512206,40.9999999999268));
#92131=CARTESIAN_POINT('Ctrl Pts',(-187.571160560859,37.3842204876452,40.9999999999178));
#92132=CARTESIAN_POINT('Ctrl Pts',(-187.499641397824,37.2229752862343,40.9999999999097));
#92133=CARTESIAN_POINT('Ctrl Pts',(-187.426953737642,37.0624868083052,40.9999999999037));
#92134=CARTESIAN_POINT('Ctrl Pts',(-187.379481793659,36.957672593416,40.9999999998998));
#92135=CARTESIAN_POINT('Ctrl Pts',(-187.331507172533,36.8531715415705,40.9999999998967));
#92136=CARTESIAN_POINT('Ctrl Pts',(-187.283032855265,36.7489815473987,40.9999999998944));
#92137=CARTESIAN_POINT('Ctrl Pts',(-187.00428820088,36.1498518318543,40.9999999998812));
#92138=CARTESIAN_POINT('Ctrl Pts',(-186.70902499862,35.5610077961926,40.9999999998937));
#92139=CARTESIAN_POINT('Ctrl Pts',(-186.397799748604,34.9821024060981,40.9999999999139));
#92140=CARTESIAN_POINT('Ctrl Pts',(-186.147394527304,34.5163274334359,40.9999999999302));
#92141=CARTESIAN_POINT('Ctrl Pts',(-185.886655271096,34.0569865721678,40.9999999999514));
#92142=CARTESIAN_POINT('Ctrl Pts',(-185.615851289347,33.6039114545961,40.9999999999676));
#92143=CARTESIAN_POINT('Ctrl Pts',(-185.43368915347,33.2991407101028,40.9999999999785));
#92144=CARTESIAN_POINT('Ctrl Pts',(-185.246972491802,32.9972053740416,40.9999999999872));
#92145=CARTESIAN_POINT('Ctrl Pts',(-185.055779072472,32.6980570974861,40.9999999999907));
#92146=CARTESIAN_POINT('Ctrl Pts',(-184.962742517282,32.5524886713373,40.9999999999924));
#92147=CARTESIAN_POINT('Ctrl Pts',(-184.868646723106,32.4075816278813,40.9999999999931));
#92148=CARTESIAN_POINT('Ctrl Pts',(-184.773504430614,32.2633364214931,40.9999999999929));
#92149=CARTESIAN_POINT('Ctrl Pts',(-184.458585155278,31.7858873851478,40.999999999992));
#92150=CARTESIAN_POINT('Ctrl Pts',(-184.132137181499,31.3155633445286,40.9999999999869));
#92151=CARTESIAN_POINT('Ctrl Pts',(-183.794494884448,30.8522043465452,40.9999999999853));
#92152=CARTESIAN_POINT('Ctrl Pts',(-183.591224917035,30.5732494607284,40.9999999999844));
#92153=CARTESIAN_POINT('Ctrl Pts',(-183.383897782516,30.2968189244016,40.9999999999847));
#92154=CARTESIAN_POINT('Ctrl Pts',(-183.172587081022,30.0228774709136,40.9999999999881));
#92155=CARTESIAN_POINT('Ctrl Pts',(-183.108845303359,29.9402431551997,40.9999999999891));
#92156=CARTESIAN_POINT('Ctrl Pts',(-183.044739012704,29.857832773681,40.9999999999905));
#92157=CARTESIAN_POINT('Ctrl Pts',(-182.980283594838,29.7756622281338,40.9999999999917));
#92158=CARTESIAN_POINT('Ctrl Pts',(-182.905546559319,29.6803842331343,40.999999999993));
#92159=CARTESIAN_POINT('Ctrl Pts',(-182.830335932828,29.5854231532485,40.9999999999942));
#92160=CARTESIAN_POINT('Ctrl Pts',(-182.754647779382,29.4907679758219,40.9999999999957));
#92161=CARTESIAN_POINT('Ctrl Pts',(-182.575856472569,29.2671725768292,40.9999999999991));
#92162=CARTESIAN_POINT('Ctrl Pts',(-182.394204884809,29.0451111870287,40.9999999999999));
#92163=CARTESIAN_POINT('Ctrl Pts',(-182.209929929983,28.8247353866391,41.0000000000001));
#92164=CARTESIAN_POINT('Ctrl Pts',(-182.12072133944,28.7180501642158,41.0000000000002));
#92165=CARTESIAN_POINT('Ctrl Pts',(-182.030898854479,28.6117613402199,41.0000000000002));
#92166=CARTESIAN_POINT('Ctrl Pts',(-181.940484260319,28.5058818454224,41.0000000000001));
#92167=CARTESIAN_POINT('Ctrl Pts',(-181.717534007252,28.2447972231964,41.0000000000001));
#92168=CARTESIAN_POINT('Ctrl Pts',(-181.491000481348,27.9862289912591,40.9999999999999));
#92169=CARTESIAN_POINT('Ctrl Pts',(-181.261802368934,27.7310307756614,40.9999999999976));
#92170=CARTESIAN_POINT('Ctrl Pts',(-181.198338976531,27.6603681322122,40.999999999997));
#92171=CARTESIAN_POINT('Ctrl Pts',(-181.134671516089,27.5899636589942,40.9999999999962));
#92172=CARTESIAN_POINT('Ctrl Pts',(-181.070819954649,27.5198349571244,40.9999999999952));
#92173=CARTESIAN_POINT('Ctrl Pts',(-181.018712159623,27.4626045317426,40.9999999999944));
#92174=CARTESIAN_POINT('Ctrl Pts',(-180.966481760453,27.4055577608882,40.9999999999934));
#92175=CARTESIAN_POINT('Ctrl Pts',(-180.914139683862,27.3487040801191,40.9999999999924));
#92176=CARTESIAN_POINT('Ctrl Pts',(-180.883283615482,27.315188385371,40.9999999999917));
#92177=CARTESIAN_POINT('Ctrl Pts',(-180.852387969248,27.2817389335116,40.999999999991));
#92178=CARTESIAN_POINT('Ctrl Pts',(-180.821445495686,27.2483474710294,40.9999999999902));
#92179=CARTESIAN_POINT('Ctrl Pts',(-180.711921869605,27.1301554317317,40.9999999999871));
#92180=CARTESIAN_POINT('Ctrl Pts',(-180.601840652286,27.0127215882594,40.9999999999823));
#92181=CARTESIAN_POINT('Ctrl Pts',(-180.491263633126,26.8960966447111,40.9999999999755));
#92182=CARTESIAN_POINT('Ctrl Pts',(-179.98837410592,26.3657019644473,40.9999999999445));
#92183=CARTESIAN_POINT('Ctrl Pts',(-179.474102428684,25.8501900736901,40.9999999999326));
#92184=CARTESIAN_POINT('Ctrl Pts',(-178.949364837618,25.3485900212007,40.9999999999311));
#92185=CARTESIAN_POINT('Ctrl Pts',(-178.394722254172,24.8184035933437,40.9999999999295));
#92186=CARTESIAN_POINT('Ctrl Pts',(-177.828386861868,24.3037598681548,40.9999999999397));
#92187=CARTESIAN_POINT('Ctrl Pts',(-177.251475858342,23.8034620495015,40.9999999999514));
#92188=CARTESIAN_POINT('Ctrl Pts',(-176.940781259065,23.5340273718199,40.9999999999577));
#92189=CARTESIAN_POINT('Ctrl Pts',(-176.62701995777,23.268752659544,40.9999999999644));
#92190=CARTESIAN_POINT('Ctrl Pts',(-176.310370263142,23.007445530886,40.99999999997));
#92191=CARTESIAN_POINT('Ctrl Pts',(-176.09830532097,22.8324443163949,40.9999999999737));
#92192=CARTESIAN_POINT('Ctrl Pts',(-175.884949396412,22.6592259929049,40.9999999999767));
#92193=CARTESIAN_POINT('Ctrl Pts',(-175.670328039924,22.4877094396632,40.9999999999798));
#92194=CARTESIAN_POINT('Ctrl Pts',(-175.610359698279,22.4397852096096,40.9999999999807));
#92195=CARTESIAN_POINT('Ctrl Pts',(-175.550292866756,22.3919940974155,40.9999999999815));
#92196=CARTESIAN_POINT('Ctrl Pts',(-175.490128584424,22.3443347300923,40.9999999999823));
#92197=CARTESIAN_POINT('Ctrl Pts',(-174.688956926142,21.7096835239187,40.9999999999932));
#92198=CARTESIAN_POINT('Ctrl Pts',(-173.870424468313,21.0984838183586,40.9999999999862));
#92199=CARTESIAN_POINT('Ctrl Pts',(-173.036110998015,20.5086051060234,40.9999999999796));
#92200=CARTESIAN_POINT('Ctrl Pts',(-172.184479498597,19.9064821508693,40.9999999999728));
#92201=CARTESIAN_POINT('Ctrl Pts',(-171.316405856158,19.326574818821,40.9999999999649));
#92202=CARTESIAN_POINT('Ctrl Pts',(-170.433598454822,18.7665715747235,40.9999999999801));
#92203=CARTESIAN_POINT('Ctrl Pts',(-170.290921642194,18.6760654486893,40.9999999999825));
#92204=CARTESIAN_POINT('Ctrl Pts',(-170.147859942551,18.5860790675574,40.9999999999858));
#92205=CARTESIAN_POINT('Ctrl Pts',(-170.004420653322,18.4966025861836,40.99999999999));
#92206=CARTESIAN_POINT('Ctrl Pts',(-169.057564734203,17.9059601166997,41.0000000000176));
#92207=CARTESIAN_POINT('Ctrl Pts',(-168.094206320727,17.3375962595065,41.0000000000171));
#92208=CARTESIAN_POINT('Ctrl Pts',(-167.115805421991,16.7895568522908,41.0000000000111));
#92209=CARTESIAN_POINT('Ctrl Pts',(-166.424537246453,16.4023513605147,41.0000000000068));
#92210=CARTESIAN_POINT('Ctrl Pts',(-165.725760727533,16.025290592085,40.9999999999997));
#92211=CARTESIAN_POINT('Ctrl Pts',(-165.019998607327,15.6576738469852,40.9999999999979));
#92212=CARTESIAN_POINT('Ctrl Pts',(-164.796837319539,15.541433793998,40.9999999999973));
#92213=CARTESIAN_POINT('Ctrl Pts',(-164.572975928768,15.4261369848494,40.9999999999972));
#92214=CARTESIAN_POINT('Ctrl Pts',(-164.348424175168,15.3117577010838,40.9999999999975));
#92215=CARTESIAN_POINT('Ctrl Pts',(-164.277996273564,15.2758840425021,40.9999999999976));
#92216=CARTESIAN_POINT('Ctrl Pts',(-164.207500742519,15.2401007843316,40.9999999999977));
#92217=CARTESIAN_POINT('Ctrl Pts',(-164.136938205308,15.204407296028,40.9999999999979));
#92218=CARTESIAN_POINT('Ctrl Pts',(-163.634767706658,14.9503884139369,40.9999999999993));
#92219=CARTESIAN_POINT('Ctrl Pts',(-163.130528643012,14.701581308456,40.9999999999997));
#92220=CARTESIAN_POINT('Ctrl Pts',(-162.624382406767,14.4577468036969,40.9999999999999));
#92221=CARTESIAN_POINT('Ctrl Pts',(-162.333101907192,14.3174232543474,40.9999999999999));
#92222=CARTESIAN_POINT('Ctrl Pts',(-162.041191333437,14.1787471618155,40.9999999999999));
#92223=CARTESIAN_POINT('Ctrl Pts',(-161.748676951111,14.0416699123734,40.9999999999999));
#92224=CARTESIAN_POINT('Ctrl Pts',(-161.024703460289,13.7024035351041,40.9999999999999));
#92225=CARTESIAN_POINT('Ctrl Pts',(-160.296989156764,13.3729114062466,41.));
#92226=CARTESIAN_POINT('Ctrl Pts',(-159.565837204964,13.0524114796293,41.));
#92227=CARTESIAN_POINT('Ctrl Pts',(-159.052413363196,12.8273525117845,41.));
#92228=CARTESIAN_POINT('Ctrl Pts',(-158.537289951449,12.6067257478939,41.0000000000012));
#92229=CARTESIAN_POINT('Ctrl Pts',(-158.020595184326,12.3902690198921,40.9999999999964));
#92230=CARTESIAN_POINT('Ctrl Pts',(-156.620459513298,11.803716174009,40.9999999999833));
#92231=CARTESIAN_POINT('Ctrl Pts',(-155.208729326418,11.2473855688854,40.9999999999796));
#92232=CARTESIAN_POINT('Ctrl Pts',(-153.786660840674,10.7180565395898,40.9999999999779));
#92233=CARTESIAN_POINT('Ctrl Pts',(-152.404789951638,10.2036900490597,40.9999999999763));
#92234=CARTESIAN_POINT('Ctrl Pts',(-151.01315718763,9.71481955399222,40.9999999999766));
#92235=CARTESIAN_POINT('Ctrl Pts',(-149.612929914259,9.24844692736709,40.9999999999717));
#92236=CARTESIAN_POINT('Ctrl Pts',(-148.892028742829,9.00833692576161,40.9999999999693));
#92237=CARTESIAN_POINT('Ctrl Pts',(-148.168849678895,8.77418970238386,40.9999999999654));
#92238=CARTESIAN_POINT('Ctrl Pts',(-147.443553337577,8.54559230069181,40.9999999999593));
#92239=CARTESIAN_POINT('Ctrl Pts',(-147.074239559723,8.42919274754762,40.9999999999562));
#92240=CARTESIAN_POINT('Ctrl Pts',(-146.704376838914,8.3142320835025,40.9999999999524));
#92241=CARTESIAN_POINT('Ctrl Pts',(-146.333986459289,8.20065555828211,40.999999999948));
#92242=CARTESIAN_POINT('Ctrl Pts',(-146.076894129919,8.12182075306847,40.9999999999449));
#92243=CARTESIAN_POINT('Ctrl Pts',(-145.819544077849,8.04365172394714,40.9999999999402));
#92244=CARTESIAN_POINT('Ctrl Pts',(-145.561936540897,7.96612814281965,40.9999999999303));
#92245=CARTESIAN_POINT('Ctrl Pts',(-145.503842861038,7.94864561821321,40.9999999999281));
#92246=CARTESIAN_POINT('Ctrl Pts',(-145.445736226424,7.93119596097413,40.9999999999257));
#92247=CARTESIAN_POINT('Ctrl Pts',(-145.387616747528,7.91377897036687,40.999999999923));
#92248=CARTESIAN_POINT('Ctrl Pts',(-144.317135170216,7.59298174487044,40.9999999998743));
#92249=CARTESIAN_POINT('Ctrl Pts',(-143.242915326353,7.28372140949535,40.9999999998847));
#92250=CARTESIAN_POINT('Ctrl Pts',(-142.16642871014,6.9853813390909,40.9999999999084));
#92251=CARTESIAN_POINT('Ctrl Pts',(-141.628185402034,6.83621130388867,40.9999999999202));
#92252=CARTESIAN_POINT('Ctrl Pts',(-141.089375548839,6.68977097174617,40.9999999999353));
#92253=CARTESIAN_POINT('Ctrl Pts',(-140.550183738394,6.54598122051974,40.9999999999481));
#92254=CARTESIAN_POINT('Ctrl Pts',(-140.301162777883,6.47957319786708,40.9999999999539));
#92255=CARTESIAN_POINT('Ctrl Pts',(-140.052060351194,6.41373051878849,40.9999999999593));
#92256=CARTESIAN_POINT('Ctrl Pts',(-139.802894658828,6.34844529911264,40.9999999999636));
#92257=CARTESIAN_POINT('Ctrl Pts',(-139.654849521108,6.30965521029164,40.9999999999661));
#92258=CARTESIAN_POINT('Ctrl Pts',(-139.506778229424,6.27106091261389,40.9999999999684));
#92259=CARTESIAN_POINT('Ctrl Pts',(-139.358676711506,6.23265874940007,40.9999999999706));
#92260=CARTESIAN_POINT('Ctrl Pts',(-139.216328160858,6.19574830883112,40.9999999999728));
#92261=CARTESIAN_POINT('Ctrl Pts',(-139.073953826219,6.15901592701736,40.9999999999747));
#92262=CARTESIAN_POINT('Ctrl Pts',(-138.931556952871,6.122460150616,40.9999999999763));
#92263=CARTESIAN_POINT('Ctrl Pts',(-137.852774493575,5.84551776107746,40.9999999999883));
#92264=CARTESIAN_POINT('Ctrl Pts',(-136.772065878145,5.57853332011435,40.9999999999726));
#92265=CARTESIAN_POINT('Ctrl Pts',(-135.68972235984,5.32079043385352,40.9999999999605));
#92266=CARTESIAN_POINT('Ctrl Pts',(-135.07155026317,5.17358258559918,40.9999999999537));
#92267=CARTESIAN_POINT('Ctrl Pts',(-134.45284490054,5.02938905934688,40.999999999948));
#92268=CARTESIAN_POINT('Ctrl Pts',(-133.833660863296,4.888074170245,40.9999999999494));
#92269=CARTESIAN_POINT('Ctrl Pts',(-133.368729598412,4.78196402175094,40.9999999999505));
#92270=CARTESIAN_POINT('Ctrl Pts',(-132.903533275812,4.67747788586212,40.9999999999548));
#92271=CARTESIAN_POINT('Ctrl Pts',(-132.438061496091,4.57455049696325,40.9999999999709));
#92272=CARTESIAN_POINT('Ctrl Pts',(-129.978499200868,4.03068009297673,41.0000000000562));
#92273=CARTESIAN_POINT('Ctrl Pts',(-127.511390385521,3.53007933571102,41.0000000000492));
#92274=CARTESIAN_POINT('Ctrl Pts',(-125.037816464169,3.06656201112882,41.0000000000282));
#92275=CARTESIAN_POINT('Ctrl Pts',(-123.149548259225,2.71272377775557,41.0000000000122));
#92276=CARTESIAN_POINT('Ctrl Pts',(-121.257513320784,2.38049453077747,40.999999999987));
#92277=CARTESIAN_POINT('Ctrl Pts',(-119.362193676919,2.06710298218835,40.9999999999911));
#92278=CARTESIAN_POINT('Ctrl Pts',(-117.175237669972,1.70548929241751,40.9999999999958));
#92279=CARTESIAN_POINT('Ctrl Pts',(-114.983887583549,1.36907516990482,40.999999999998));
#92280=CARTESIAN_POINT('Ctrl Pts',(-112.788634863691,1.05504893658129,40.9999999999991));
#92281=CARTESIAN_POINT('Ctrl Pts',(-111.65029988351,0.89221253836014,40.9999999999996));
#92282=CARTESIAN_POINT('Ctrl Pts',(-110.510915568272,0.735395733931361,
40.9999999999999));
#92283=CARTESIAN_POINT('Ctrl Pts',(-109.370550654786,0.584205063488431,
40.9999999999999));
#92284=CARTESIAN_POINT('Ctrl Pts',(-108.698866089248,0.495152481644728,
41.));
#92285=CARTESIAN_POINT('Ctrl Pts',(-108.02684132648,0.408051762178606,41.));
#92286=CARTESIAN_POINT('Ctrl Pts',(-107.354490434212,0.322822359446492,
41.));
#92287=CARTESIAN_POINT('Ctrl Pts',(-106.96698848389,0.273701342187092,41.));
#92288=CARTESIAN_POINT('Ctrl Pts',(-106.579377911394,0.225201882287813,
41.));
#92289=CARTESIAN_POINT('Ctrl Pts',(-106.19166867118,0.177309421133637,41.));
#92290=CARTESIAN_POINT('Ctrl Pts',(-103.990648852084,-0.0945753967966797,
41.));
#92291=CARTESIAN_POINT('Ctrl Pts',(-101.78586236742,-0.346893843387375,
41.));
#92292=CARTESIAN_POINT('Ctrl Pts',(-99.5782059295342,-0.581609328457616,
41.));
#92293=CARTESIAN_POINT('Ctrl Pts',(-98.4707994783828,-0.699347504512224,
41.));
#92294=CARTESIAN_POINT('Ctrl Pts',(-97.3626708656601,-0.812656151974744,
41.));
#92295=CARTESIAN_POINT('Ctrl Pts',(-96.2539332971608,-0.921782003691591,
41.));
#92296=CARTESIAN_POINT('Ctrl Pts',(-95.4162205862063,-1.00423263554009,
41.));
#92297=CARTESIAN_POINT('Ctrl Pts',(-94.5781602445548,-1.08429544478856,
41.));
#92298=CARTESIAN_POINT('Ctrl Pts',(-93.7398011429836,-1.16207664008724,
41.));
#92299=CARTESIAN_POINT('Ctrl Pts',(-93.4757377541879,-1.18657588626546,
41.));
#92300=CARTESIAN_POINT('Ctrl Pts',(-93.2116456158809,-1.21084868819005,
41.));
#92301=CARTESIAN_POINT('Ctrl Pts',(-92.9475282938307,-1.23489818414305,
41.));
#92302=CARTESIAN_POINT('Ctrl Pts',(-90.7372300593495,-1.43615934351134,
41.));
#92303=CARTESIAN_POINT('Ctrl Pts',(-88.5261974020728,-1.62168029502631,
41.));
#92304=CARTESIAN_POINT('Ctrl Pts',(-86.3143658196803,-1.79305840637293,
41.));
#92305=CARTESIAN_POINT('Ctrl Pts',(-84.9944564499124,-1.89532820699439,
41.));
#92306=CARTESIAN_POINT('Ctrl Pts',(-83.6742625748037,-1.99256160295836,
41.));
#92307=CARTESIAN_POINT('Ctrl Pts',(-82.3537704872285,-2.08509819210469,
41.));
#92308=CARTESIAN_POINT('Ctrl Pts',(-81.5348603298117,-2.14248524765592,
41.));
#92309=CARTESIAN_POINT('Ctrl Pts',(-80.7158331792441,-2.19806609943898,
41.));
#92310=CARTESIAN_POINT('Ctrl Pts',(-79.8966933309586,-2.25192128951806,
41.));
#92311=CARTESIAN_POINT('Ctrl Pts',(-79.8232669179519,-2.25674878440502,
41.));
#92312=CARTESIAN_POINT('Ctrl Pts',(-79.7498396409215,-2.26156241089664,
41.));
#92313=CARTESIAN_POINT('Ctrl Pts',(-79.6764115035435,-2.26636222707692,
41.));
#92314=CARTESIAN_POINT('Ctrl Pts',(-75.9717789993547,-2.50852491389651,
41.));
#92315=CARTESIAN_POINT('Ctrl Pts',(-72.264953695338,-2.7157624742687,41.));
#92316=CARTESIAN_POINT('Ctrl Pts',(-68.5564163959988,-2.89342107889025,
41.));
#92317=CARTESIAN_POINT('Ctrl Pts',(-65.9855045365144,-3.0165813916212,41.));
#92318=CARTESIAN_POINT('Ctrl Pts',(-63.4137699397649,-3.1255277688436,41.));
#92319=CARTESIAN_POINT('Ctrl Pts',(-60.8413730070096,-3.22205506124308,
41.));
#92320=CARTESIAN_POINT('Ctrl Pts',(-59.5551745406319,-3.27031870744282,
41.));
#92321=CARTESIAN_POINT('Ctrl Pts',(-58.2688104927504,-3.31547774299482,
41.));
#92322=CARTESIAN_POINT('Ctrl Pts',(-56.9823009271456,-3.35775741157833,
41.));
#92323=CARTESIAN_POINT('Ctrl Pts',(-56.240043581815,-3.38215085209619,41.));
#92324=CARTESIAN_POINT('Ctrl Pts',(-55.4977377972299,-3.40558582972323,
41.));
#92325=CARTESIAN_POINT('Ctrl Pts',(-54.7553874279252,-3.42810568308979,
41.));
#92326=CARTESIAN_POINT('Ctrl Pts',(-54.3016290330985,-3.44187084430996,
41.));
#92327=CARTESIAN_POINT('Ctrl Pts',(-53.8478518097628,-3.45529415926112,
41.));
#92328=CARTESIAN_POINT('Ctrl Pts',(-53.3940635403805,-3.4683853368097,41.));
#92329=CARTESIAN_POINT('Ctrl Pts',(-53.3034955436783,-3.47099810096656,
41.));
#92330=CARTESIAN_POINT('Ctrl Pts',(-53.2129274197839,-3.47359762622963,
41.));
#92331=CARTESIAN_POINT('Ctrl Pts',(-53.1223591687654,-3.47618399202878,
41.));
#92332=CARTESIAN_POINT('Ctrl Pts',(-47.2953401631429,-3.64258670487363,
41.));
#92333=CARTESIAN_POINT('Ctrl Pts',(-41.4677740863017,-3.7537775757723,41.));
#92334=CARTESIAN_POINT('Ctrl Pts',(-35.639833792225,-3.8272049942722,41.));
#92335=CARTESIAN_POINT('Ctrl Pts',(-32.6131542432301,-3.86533875246033,
41.));
#92336=CARTESIAN_POINT('Ctrl Pts',(-29.5863734940691,-3.89328680280741,
41.));
#92337=CARTESIAN_POINT('Ctrl Pts',(-26.5595165690504,-3.91349171933101,
41.));
#92338=CARTESIAN_POINT('Ctrl Pts',(-20.0200301960568,-3.95714418773194,
41.));
#92339=CARTESIAN_POINT('Ctrl Pts',(-13.4801699608071,-3.96312141411588,
41.));
#92340=CARTESIAN_POINT('Ctrl Pts',(-6.94025147230322,-3.96326053282878,
41.));
#92341=CARTESIAN_POINT('Ctrl Pts',(-4.62683685123245,-3.96330974433885,
41.));
#92342=CARTESIAN_POINT('Ctrl Pts',(-2.31341497974243,-3.96262874552467,
41.));
#92343=CARTESIAN_POINT('Ctrl Pts',(7.71069805227384E-15,-3.96262874552467,
41.));
#92344=CARTESIAN_POINT('Ctrl Pts',(7.58040827681699E-15,-2.96262874552467,
40.));
#92345=CARTESIAN_POINT('Ctrl Pts',(-8.85144823879692,-2.96262874562831,
40.));
#92346=CARTESIAN_POINT('Ctrl Pts',(-17.7032012684452,-2.97258723674216,
40.));
#92347=CARTESIAN_POINT('Ctrl Pts',(-26.5528415041601,-2.91351399783701,
40.));
#92348=CARTESIAN_POINT('Ctrl Pts',(-35.402481739875,-2.85444075893186,40.));
#92349=CARTESIAN_POINT('Ctrl Pts',(-44.2500950803765,-2.72914237566079,
40.));
#92350=CARTESIAN_POINT('Ctrl Pts',(-53.0938137147646,-2.4765914965461,40.));
#92351=CARTESIAN_POINT('Ctrl Pts',(-61.9375323491527,-2.22404061743142,
40.));
#92352=CARTESIAN_POINT('Ctrl Pts',(-70.7774082066898,-1.84593393741772,
40.));
#92353=CARTESIAN_POINT('Ctrl Pts',(-79.6111831796923,-1.26849186187931,
40.));
#92354=CARTESIAN_POINT('Ctrl Pts',(-84.0280706661936,-0.979770824110103,
40.));
#92355=CARTESIAN_POINT('Ctrl Pts',(-88.4434228779194,-0.640887452775866,
40.0000000000001));
#92356=CARTESIAN_POINT('Ctrl Pts',(-92.8568473354026,-0.239018189490933,
40.0000000000001));
#92357=CARTESIAN_POINT('Ctrl Pts',(-97.2702717928858,0.162851073794002,
40.0000000000001));
#92358=CARTESIAN_POINT('Ctrl Pts',(-101.677510051147,0.627290636607177,
40.));
#92359=CARTESIAN_POINT('Ctrl Pts',(-106.069073712797,1.16976620918298,40.));
#92360=CARTESIAN_POINT('Ctrl Pts',(-110.460637374447,1.71224178175879,40.));
#92361=CARTESIAN_POINT('Ctrl Pts',(-114.838608995747,2.33270535869012,40.));
#92362=CARTESIAN_POINT('Ctrl Pts',(-119.199058518279,3.05370671214597,40.));
#92363=CARTESIAN_POINT('Ctrl Pts',(-123.559508040812,3.77470806560183,40.));
#92364=CARTESIAN_POINT('Ctrl Pts',(-127.902516032416,4.59578491584501,40.));
#92365=CARTESIAN_POINT('Ctrl Pts',(-132.222152200056,5.55096392160199,40.));
#92366=CARTESIAN_POINT('Ctrl Pts',(-134.381970283877,6.02855342448048,40.));
#92367=CARTESIAN_POINT('Ctrl Pts',(-136.535908314317,6.53988132256321,40.));
#92368=CARTESIAN_POINT('Ctrl Pts',(-138.682902332726,7.09105236606981,40.));
#92369=CARTESIAN_POINT('Ctrl Pts',(-140.829896351135,7.6422234095764,40.));
#92370=CARTESIAN_POINT('Ctrl Pts',(-142.97246355619,8.23395393720208,40.));
#92371=CARTESIAN_POINT('Ctrl Pts',(-145.100553949739,8.87169073562511,40.));
#92372=CARTESIAN_POINT('Ctrl Pts',(-149.356734736836,10.1471643324712,40.));
#92373=CARTESIAN_POINT('Ctrl Pts',(-153.545256591528,11.5996387775139,40.0000000000001));
#92374=CARTESIAN_POINT('Ctrl Pts',(-157.634205130681,13.3126044937319,40.0000000000001));
#92375=CARTESIAN_POINT('Ctrl Pts',(-159.678679400257,14.1690873518408,40.0000000000001));
#92376=CARTESIAN_POINT('Ctrl Pts',(-161.698333060539,15.0915173717773,40.));
#92377=CARTESIAN_POINT('Ctrl Pts',(-163.685559133974,16.0967395961537,40.));
#92378=CARTESIAN_POINT('Ctrl Pts',(-165.672785207409,17.1019618205302,40.));
#92379=CARTESIAN_POINT('Ctrl Pts',(-167.606564886913,18.179444580804,40.0000000000001));
#92380=CARTESIAN_POINT('Ctrl Pts',(-169.475158094859,19.3450606841723,40.0000000000001));
#92381=CARTESIAN_POINT('Ctrl Pts',(-171.343751302806,20.5106767875407,40.0000000000001));
#92382=CARTESIAN_POINT('Ctrl Pts',(-173.147319648035,21.7642077357359,40.));
#92383=CARTESIAN_POINT('Ctrl Pts',(-174.869190918009,23.1281946756062,40.));
#92384=CARTESIAN_POINT('Ctrl Pts',(-176.591062187983,24.4921816154764,40.));
#92385=CARTESIAN_POINT('Ctrl Pts',(-178.23155329653,25.966196073619,39.9999999999999));
#92386=CARTESIAN_POINT('Ctrl Pts',(-179.765591319341,27.5841371179025,39.9999999999999));
#92387=CARTESIAN_POINT('Ctrl Pts',(-180.532610330747,28.3931076400442,39.9999999999999));
#92388=CARTESIAN_POINT('Ctrl Pts',(-181.275699297867,29.2424485691303,40.));
#92389=CARTESIAN_POINT('Ctrl Pts',(-181.973634139114,30.1152819417224,40.));
#92390=CARTESIAN_POINT('Ctrl Pts',(-182.671568980361,30.9881153143144,40.));
#92391=CARTESIAN_POINT('Ctrl Pts',(-183.327437398447,31.8871479480752,40.0000000000001));
#92392=CARTESIAN_POINT('Ctrl Pts',(-183.938736638342,32.8139385762865,40.0000000000001));
#92393=CARTESIAN_POINT('Ctrl Pts',(-185.161335118131,34.6675198327091,40.0000000000001));
#92394=CARTESIAN_POINT('Ctrl Pts',(-186.206617846403,36.6337883765178,40.));
#92395=CARTESIAN_POINT('Ctrl Pts',(-187.049713891119,38.7214305741511,40.));
#92396=CARTESIAN_POINT('Ctrl Pts',(-187.892809935835,40.8090727717843,40.));
#92397=CARTESIAN_POINT('Ctrl Pts',(-188.505057255607,42.9465120075526,40.));
#92398=CARTESIAN_POINT('Ctrl Pts',(-188.906974096078,45.129322231996,40.));
#92399=CARTESIAN_POINT('Ctrl Pts',(-189.107932516313,46.2207273442177,40.));
#92400=CARTESIAN_POINT('Ctrl Pts',(-189.256273490652,47.3234827160355,40.));
#92401=CARTESIAN_POINT('Ctrl Pts',(-189.354350399695,48.4370806930155,40.));
#92402=CARTESIAN_POINT('Ctrl Pts',(-189.405887616132,49.0222514587305,40.));
#92403=CARTESIAN_POINT('Ctrl Pts',(-189.443467838815,49.6109038488981,40.));
#92404=CARTESIAN_POINT('Ctrl Pts',(-189.467540106621,50.2009603371434,40.));
#92405=CARTESIAN_POINT('Ctrl Pts',(-189.489278105322,50.7337995062214,40.));
#92406=CARTESIAN_POINT('Ctrl Pts',(-189.500000000133,51.2677847576647,40.));
#92407=CARTESIAN_POINT('Ctrl Pts',(-189.5,51.8013867006571,40.));
#92408=CARTESIAN_POINT('Ctrl Pts',(7.59225281309826E-15,-2.96262874552467,
40.));
#92409=CARTESIAN_POINT('Ctrl Pts',(7.71069817591099E-15,-3.96262874552467,
40.));
#92410=CARTESIAN_POINT('Ctrl Pts',(7.71069817591099E-15,-3.96262874552467,
41.));
#92411=CARTESIAN_POINT('Ctrl Pts',(9.22286794822226,-2.96262874561266,40.));
#92412=CARTESIAN_POINT('Ctrl Pts',(9.22185412936952,-3.96262874542067,40.000000000576));
#92413=CARTESIAN_POINT('Ctrl Pts',(9.22185412936967,-3.96262874552467,41.000000000384));
#92414=CARTESIAN_POINT('Ctrl Pts',(18.4459311592863,-2.97316630718802,40.0000000000001));
#92415=CARTESIAN_POINT('Ctrl Pts',(18.4478537919059,-3.97317899216111,39.9999999998081));
#92416=CARTESIAN_POINT('Ctrl Pts',(18.4478537919057,-3.97317899207265,40.9999999998721));
#92417=CARTESIAN_POINT('Ctrl Pts',(36.888025186236,-2.83828047197706,40.0000000000001));
#92418=CARTESIAN_POINT('Ctrl Pts',(36.9007302013505,-3.83821429426901,40.000000000192));
#92419=CARTESIAN_POINT('Ctrl Pts',(36.9007302013507,-3.8382142943575,41.000000000128));
#92420=CARTESIAN_POINT('Ctrl Pts',(46.1071023205165,-2.69618114038663,40.));
#92421=CARTESIAN_POINT('Ctrl Pts',(46.127686373253,-3.69602375409421,40.0000000001919));
#92422=CARTESIAN_POINT('Ctrl Pts',(46.127686373252,-3.69602375412447,41.0000000001279));
#92423=CARTESIAN_POINT('Ctrl Pts',(64.5376642708818,-2.12424138803454,40.));
#92424=CARTESIAN_POINT('Ctrl Pts',(64.5791146330909,-3.12343647566289,39.999999999808));
#92425=CARTESIAN_POINT('Ctrl Pts',(64.579114633092,-3.12343647563261,40.999999999872));
#92426=CARTESIAN_POINT('Ctrl Pts',(73.7492053716307,-1.69653408055239,40.));
#92427=CARTESIAN_POINT('Ctrl Pts',(73.8036313518568,-2.69519228857308,40.0000000003842));
#92428=CARTESIAN_POINT('Ctrl Pts',(73.8036313518527,-2.69519228864398,41.0000000002562));
#92429=CARTESIAN_POINT('Ctrl Pts',(87.5574640501196,-0.711874711538739,
40.));
#92430=CARTESIAN_POINT('Ctrl Pts',(87.6369443133912,-1.70874631254166,39.9999999998079));
#92431=CARTESIAN_POINT('Ctrl Pts',(87.6369443133933,-1.70874631250621,40.9999999998719));
#92432=CARTESIAN_POINT('Ctrl Pts',(92.1597820946751,-0.325827219991832,
40.));
#92433=CARTESIAN_POINT('Ctrl Pts',(92.2485669610653,-1.32193429002331,40.));
#92434=CARTESIAN_POINT('Ctrl Pts',(92.2485669610628,-1.32193428999809,41.));
#92435=CARTESIAN_POINT('Ctrl Pts',(101.336839995159,0.590146567660638,40.));
#92436=CARTESIAN_POINT('Ctrl Pts',(101.446690684835,-0.403857895832186,
40.));
#92437=CARTESIAN_POINT('Ctrl Pts',(101.446690684837,-0.403857895857384,
41.));
#92438=CARTESIAN_POINT('Ctrl Pts',(105.914098473304,1.12003310600361,40.));
#92439=CARTESIAN_POINT('Ctrl Pts',(106.035715901227,0.127363203503316,40.000000000671));
#92440=CARTESIAN_POINT('Ctrl Pts',(106.035715901271,0.127363203184816,41.0000000004473));
#92441=CARTESIAN_POINT('Ctrl Pts',(110.476932254378,1.74203503103179,40.));
#92442=CARTESIAN_POINT('Ctrl Pts',(110.612002249462,0.751198971722283,40.));
#92443=CARTESIAN_POINT('Ctrl Pts',(110.612002249462,0.751198971722297,41.));
#92444=CARTESIAN_POINT('',(110.476932254378,1.74203503103179,40.));
#92445=CARTESIAN_POINT('',(110.612002249462,0.751198971722297,41.));
#92446=CARTESIAN_POINT('Origin',(110.476932254378,1.74203503103178,41.));
#92447=CARTESIAN_POINT('Ctrl Pts',(7.71069817591099E-15,-3.96262874552467,
41.));
#92448=CARTESIAN_POINT('Ctrl Pts',(5.82930178377565,-3.96262874552467,41.));
#92449=CARTESIAN_POINT('Ctrl Pts',(11.6587149026642,-3.96683913664252,40.9999999999486));
#92450=CARTESIAN_POINT('Ctrl Pts',(17.4876489527825,-3.95291174806464,40.9999999999272));
#92451=CARTESIAN_POINT('Ctrl Pts',(20.8833979233155,-3.94479810069465,40.9999999999147));
#92452=CARTESIAN_POINT('Ctrl Pts',(24.2789843696462,-3.93052998937519,40.9999999999123));
#92453=CARTESIAN_POINT('Ctrl Pts',(27.6742919966282,-3.90569664321507,40.9999999999361));
#92454=CARTESIAN_POINT('Ctrl Pts',(33.9894118154414,-3.8595077337752,40.9999999999802));
#92455=CARTESIAN_POINT('Ctrl Pts',(40.3036077491836,-3.77832350323118,40.9999999999941));
#92456=CARTESIAN_POINT('Ctrl Pts',(46.61629413806,-3.63995619654589,40.9999999999781));
#92457=CARTESIAN_POINT('Ctrl Pts',(49.5290034318352,-3.57611273667641,40.9999999999707));
#92458=CARTESIAN_POINT('Ctrl Pts',(52.4413913669821,-3.50009598589696,40.9999999999568));
#92459=CARTESIAN_POINT('Ctrl Pts',(55.353400503172,-3.40973011487854,40.9999999999364));
#92460=CARTESIAN_POINT('Ctrl Pts',(60.455282861202,-3.25140779459896,40.9999999999007));
#92461=CARTESIAN_POINT('Ctrl Pts',(65.5560203048567,-3.04969502865525,40.9999999999245));
#92462=CARTESIAN_POINT('Ctrl Pts',(70.6552234068538,-2.78987297547265,40.999999999938));
#92463=CARTESIAN_POINT('Ctrl Pts',(74.779834762682,-2.57970974611788,40.999999999949));
#92464=CARTESIAN_POINT('Ctrl Pts',(78.9034422335561,-2.33152756586165,40.9999999999533));
#92465=CARTESIAN_POINT('Ctrl Pts',(83.0258399928798,-2.03756163788547,40.9999999999148));
#92466=CARTESIAN_POINT('Ctrl Pts',(83.702952471426,-1.98927711763268,40.9999999999085));
#92467=CARTESIAN_POINT('Ctrl Pts',(84.3800458281722,-1.9397441896904,40.9999999999059));
#92468=CARTESIAN_POINT('Ctrl Pts',(85.0570974588133,-1.8889166619343,40.999999999906));
#92469=CARTESIAN_POINT('Ctrl Pts',(87.0236209542901,-1.74128607805296,40.9999999999064));
#92470=CARTESIAN_POINT('Ctrl Pts',(88.9897932279612,-1.58273540574224,40.9999999999299));
#92471=CARTESIAN_POINT('Ctrl Pts',(90.9550653787228,-1.4121181790945,40.9999999999533));
#92472=CARTESIAN_POINT('Ctrl Pts',(91.9377014541036,-1.32680956577063,40.999999999965));
#92473=CARTESIAN_POINT('Ctrl Pts',(92.9201124704526,-1.23848396737367,40.9999999999766));
#92474=CARTESIAN_POINT('Ctrl Pts',(93.9022294421414,-1.14699577506546,40.9999999999854));
#92475=CARTESIAN_POINT('Ctrl Pts',(94.3953787582656,-1.10105690956286,40.9999999999898));
#92476=CARTESIAN_POINT('Ctrl Pts',(94.8884539303434,-1.05432062249788,40.9999999999934));
#92477=CARTESIAN_POINT('Ctrl Pts',(95.381446184432,-1.00676831544679,40.999999999996));
#92478=CARTESIAN_POINT('Ctrl Pts',(95.7294863070638,-0.973197583573767,
40.9999999999978));
#92479=CARTESIAN_POINT('Ctrl Pts',(96.0774851027509,-0.939220144658271,
40.9999999999991));
#92480=CARTESIAN_POINT('Ctrl Pts',(96.4254394745113,-0.904829419904913,
40.9999999999996));
#92481=CARTESIAN_POINT('Ctrl Pts',(96.5661765935577,-0.890919402050511,
40.9999999999999));
#92482=CARTESIAN_POINT('Ctrl Pts',(96.7069064798408,-0.876941768460753,
41.));
#92483=CARTESIAN_POINT('Ctrl Pts',(96.84762882295,-0.862896092927736,41.));
#92484=CARTESIAN_POINT('Ctrl Pts',(100.443648508519,-0.503972807556701,
40.9999999999998));
#92485=CARTESIAN_POINT('Ctrl Pts',(104.034503830642,-0.100826113757949,
40.9999999999999));
#92486=CARTESIAN_POINT('Ctrl Pts',(107.619039731541,0.356421973888414,41.));
#92487=CARTESIAN_POINT('Ctrl Pts',(108.61719230131,0.483747621147737,41.));
#92488=CARTESIAN_POINT('Ctrl Pts',(109.61485481989,0.615268615590165,41.));
#92489=CARTESIAN_POINT('Ctrl Pts',(110.612002249462,0.751198971722297,41.));
#92490=CARTESIAN_POINT('Ctrl Pts',(110.476932254378,1.74203503103179,40.));
#92491=CARTESIAN_POINT('Ctrl Pts',(107.65673548948,1.35758801823668,40.));
#92492=CARTESIAN_POINT('Ctrl Pts',(104.832744534644,1.0085602200593,40.));
#92493=CARTESIAN_POINT('Ctrl Pts',(102.005490363231,0.690046765893749,40.0000000000001));
#92494=CARTESIAN_POINT('Ctrl Pts',(100.25430781925,0.492761637942585,40.0000000000001));
#92495=CARTESIAN_POINT('Ctrl Pts',(98.5018731756585,0.307184392575044,40.0000000000001));
#92496=CARTESIAN_POINT('Ctrl Pts',(96.74831108378,0.132159284469113,40.));
#92497=CARTESIAN_POINT('Ctrl Pts',(96.7415197154669,0.13148142995875,40.));
#92498=CARTESIAN_POINT('Ctrl Pts',(96.7347283247242,0.130803733819283,40.));
#92499=CARTESIAN_POINT('Ctrl Pts',(96.7279369115921,0.13012619600356,40.));
#92500=CARTESIAN_POINT('Ctrl Pts',(94.2757194146321,-0.114516568948024,
40.));
#92501=CARTESIAN_POINT('Ctrl Pts',(91.8208450764136,-0.338497674584954,
40.0000000000002));
#92502=CARTESIAN_POINT('Ctrl Pts',(89.364611533855,-0.544078641455991,40.0000000000008));
#92503=CARTESIAN_POINT('Ctrl Pts',(87.2287242584436,-0.722847379688103,
40.0000000000013));
#92504=CARTESIAN_POINT('Ctrl Pts',(85.0918085318741,-0.88770123381528,40.0000000000019));
#92505=CARTESIAN_POINT('Ctrl Pts',(82.9547112714115,-1.04009610158038,40.0000000000013));
#92506=CARTESIAN_POINT('Ctrl Pts',(82.9478289630004,-1.04058687404059,40.0000000000013));
#92507=CARTESIAN_POINT('Ctrl Pts',(82.9409466503039,-1.04107751870878,40.0000000000013));
#92508=CARTESIAN_POINT('Ctrl Pts',(82.9340643333063,-1.04156803562236,40.0000000000013));
#92509=CARTESIAN_POINT('Ctrl Pts',(73.7354319150329,-1.69717352205083,39.9999999999987));
#92510=CARTESIAN_POINT('Ctrl Pts',(64.5307746673837,-2.12445562062589,40.));
#92511=CARTESIAN_POINT('Ctrl Pts',(55.322383302435,-2.41021148127205,40.));
#92512=CARTESIAN_POINT('Ctrl Pts',(55.3177902240801,-2.41035401420819,40.));
#92513=CARTESIAN_POINT('Ctrl Pts',(55.3131971447822,-2.41049651140351,40.));
#92514=CARTESIAN_POINT('Ctrl Pts',(55.3086040645415,-2.41063897286659,40.));
#92515=CARTESIAN_POINT('Ctrl Pts',(46.0979123788003,-2.69632277214192,39.9999999999999));
#92516=CARTESIAN_POINT('Ctrl Pts',(36.8834292267035,-2.83831408691453,39.9999999999997));
#92517=CARTESIAN_POINT('Ctrl Pts',(27.6669781789878,-2.90572424091316,40.0000000000004));
#92518=CARTESIAN_POINT('Ctrl Pts',(27.6646802028605,-2.90574104856763,40.0000000000004));
#92519=CARTESIAN_POINT('Ctrl Pts',(27.6623822266079,-2.90575785137913,40.0000000000004));
#92520=CARTESIAN_POINT('Ctrl Pts',(27.6600842502302,-2.90577464934903,40.0000000000004));
#92521=CARTESIAN_POINT('Ctrl Pts',(18.4413342218722,-2.97316275959541,40.0000000000011));
#92522=CARTESIAN_POINT('Ctrl Pts',(9.22052813832371,-2.96262874561264,40.));
#92523=CARTESIAN_POINT('Ctrl Pts',(7.59225281309826E-15,-2.96262874552467,
40.));
#92524=CARTESIAN_POINT('Origin',(110.747072244546,-0.239637087587196,41.));
#92525=CARTESIAN_POINT('',(111.732514372547,1.50073753081004,40.));
#92526=CARTESIAN_POINT('Origin',(111.732514372547,1.50073753081004,41.));
#92527=CARTESIAN_POINT('Origin',(110.747072244546,-0.239637087587196,41.));
#92528=CARTESIAN_POINT('Origin',(110.747072244546,-0.239637087587196,40.));
#92529=CARTESIAN_POINT('Origin',(125.29348064571,25.4505574462982,41.));
#92530=CARTESIAN_POINT('',(147.519501177935,9.21794547079491,40.));
#92531=CARTESIAN_POINT('Origin',(147.519501177935,9.21794547079491,41.));
#92532=CARTESIAN_POINT('Origin',(125.29348064571,25.4505574462982,40.));
#92533=CARTESIAN_POINT('Origin',(110.747072244546,-0.239637087587196,150.608250755187));
#92534=CARTESIAN_POINT('',(110.612002249461,0.751198971722164,150.608250755189));
#92535=CARTESIAN_POINT('Origin',(110.747072244546,-0.239637087587191,150.608250755187));
#92536=CARTESIAN_POINT('',(110.612002249462,0.751198971722297,41.));
#92537=CARTESIAN_POINT('Origin',(149.134611526938,8.03836140827812,41.));
#92538=CARTESIAN_POINT('',(148.513697082188,9.93953611153414,40.));
#92539=CARTESIAN_POINT('',(148.824154304563,8.98894875990614,41.));
#92540=CARTESIAN_POINT('Origin',(148.513697082188,9.93953611153414,41.));
#92541=CARTESIAN_POINT('Origin',(149.134611526938,8.03836140827812,41.));
#92542=CARTESIAN_POINT('Origin',(149.134611526938,8.03836140827812,40.));
#92543=CARTESIAN_POINT('Ctrl Pts',(110.612002249462,0.751198971722294,150.608250755187));
#92544=CARTESIAN_POINT('Ctrl Pts',(110.946247390914,0.796763007456252,150.608250755187));
#92545=CARTESIAN_POINT('Ctrl Pts',(111.239793308547,0.630550221611425,150.608250755187));
#92546=CARTESIAN_POINT('Ctrl Pts',(110.612002230967,0.751198969201009,150.693639752826));
#92547=CARTESIAN_POINT('Ctrl Pts',(110.946247372074,0.796763018434683,150.731492884106));
#92548=CARTESIAN_POINT('Ctrl Pts',(111.23979328877,0.630550232809205,150.779028752436));
#92549=CARTESIAN_POINT('Ctrl Pts',(110.582396971373,0.758074598003006,150.775891503277));
#92550=CARTESIAN_POINT('Ctrl Pts',(110.917292843193,0.81358059931356,150.85066217237));
#92551=CARTESIAN_POINT('Ctrl Pts',(111.209697548339,0.647533917538457,150.943532248718));
#92552=CARTESIAN_POINT('Ctrl Pts',(110.473864498357,0.783673855713148,150.933269838702));
#92553=CARTESIAN_POINT('Ctrl Pts',(110.812459489596,0.875126003979084,151.073781688751));
#92554=CARTESIAN_POINT('Ctrl Pts',(111.099346993048,0.710519201534495,151.258288924866));
#92555=CARTESIAN_POINT('Ctrl Pts',(110.398057036428,0.801688169240552,151.004328255835));
#92556=CARTESIAN_POINT('Ctrl Pts',(110.738903039506,0.918545320463253,151.172655401108));
#92557=CARTESIAN_POINT('Ctrl Pts',(111.022262845842,0.754759056919205,151.400405752383));
#92558=CARTESIAN_POINT('Ctrl Pts',(110.218030599701,0.845370947931939,151.134168853203));
#92559=CARTESIAN_POINT('Ctrl Pts',(110.566311747443,1.02190104841371,151.346871626469));
#92560=CARTESIAN_POINT('Ctrl Pts',(110.839158587949,0.861480818033809,151.660086955321));
#92561=CARTESIAN_POINT('Ctrl Pts',(110.116756966979,0.870327544773072,151.190904988883));
#92562=CARTESIAN_POINT('Ctrl Pts',(110.469279013687,1.0806646106112,151.419609649809));
#92563=CARTESIAN_POINT('Ctrl Pts',(110.736134030468,0.922221916391551,151.773559220278));
#92564=CARTESIAN_POINT('Ctrl Pts',(109.898938544125,0.925233080786458,151.292822817772));
#92565=CARTESIAN_POINT('Ctrl Pts',(110.262975165541,1.20755085870014,151.542883455069));
#92566=CARTESIAN_POINT('Ctrl Pts',(110.514486881992,1.05512902874504,151.977394882657));
#92567=CARTESIAN_POINT('Ctrl Pts',(109.78151096426,0.955417648896434,151.338065123121));
#92568=CARTESIAN_POINT('Ctrl Pts',(110.152251323704,1.27662677766495,151.593100193495));
#92569=CARTESIAN_POINT('Ctrl Pts',(110.394965311842,1.12785792027832,152.067879488634));
#92570=CARTESIAN_POINT('Ctrl Pts',(109.422128673717,1.0500087684249,151.455574585986));
#92571=CARTESIAN_POINT('Ctrl Pts',(109.813360261285,1.49144507563439,151.711420401226));
#92572=CARTESIAN_POINT('Ctrl Pts',(110.029060664743,1.35452646652739,152.302898421626));
#92573=CARTESIAN_POINT('Ctrl Pts',(109.169114092848,1.1194514186453,151.51211819045));
#92574=CARTESIAN_POINT('Ctrl Pts',(109.580757706994,1.6437216273512,151.744418133447));
#92575=CARTESIAN_POINT('Ctrl Pts',(109.771307831859,1.51936475733935,152.415985623633));
#92576=CARTESIAN_POINT('Ctrl Pts',(108.649983750045,1.26921788090281,151.588936256037));
#92577=CARTESIAN_POINT('Ctrl Pts',(109.124609723565,1.95156485229409,151.736067979281));
#92578=CARTESIAN_POINT('Ctrl Pts',(109.242075229445,1.87107024784917,152.569621758969));
#92579=CARTESIAN_POINT('Ctrl Pts',(108.389788066051,1.34778888692035,151.608250755187));
#92580=CARTESIAN_POINT('Ctrl Pts',(108.904821123451,2.10515872248547,151.689264229384));
#92581=CARTESIAN_POINT('Ctrl Pts',(108.976632768029,2.05384440757191,152.608250750215));
#92582=CARTESIAN_POINT('Ctrl Pts',(108.12932364768,1.43023673425741,151.608250755187));
#92583=CARTESIAN_POINT('Ctrl Pts',(108.710714013295,2.24386148976203,151.608250755187));
#92584=CARTESIAN_POINT('Ctrl Pts',(108.710714013295,2.24386148976203,152.608250755187));
#92585=CARTESIAN_POINT('',(108.129344917475,1.43023000148885,151.608250755144));
#92586=CARTESIAN_POINT('Origin',(108.12932364768,1.43023673425741,152.608250755187));
#92587=CARTESIAN_POINT('Ctrl Pts',(110.612002249462,0.751198971722294,150.608250755189));
#92588=CARTESIAN_POINT('Ctrl Pts',(110.612002249452,0.751198971720885,150.629522166779));
#92589=CARTESIAN_POINT('Ctrl Pts',(110.610161909816,0.75162639831703,150.650481814028));
#92590=CARTESIAN_POINT('Ctrl Pts',(110.606637178143,0.752447951651463,150.671066183928));
#92591=CARTESIAN_POINT('Ctrl Pts',(110.603124557815,0.753266682043145,150.691579823791));
#92592=CARTESIAN_POINT('Ctrl Pts',(110.597938087509,0.754477085709687,150.711719134966));
#92593=CARTESIAN_POINT('Ctrl Pts',(110.591282043221,0.756034195684844,150.73139543502));
#92594=CARTESIAN_POINT('Ctrl Pts',(110.586707521022,0.757104355954006,150.744918432687));
#92595=CARTESIAN_POINT('Ctrl Pts',(110.581439972465,0.758338012708028,150.758222724358));
#92596=CARTESIAN_POINT('Ctrl Pts',(110.575559656037,0.759717155612428,150.771279454307));
#92597=CARTESIAN_POINT('Ctrl Pts',(110.570108513205,0.760995642076692,150.783383241706));
#92598=CARTESIAN_POINT('Ctrl Pts',(110.564129055894,0.762399560426148,150.795277264634));
#92599=CARTESIAN_POINT('Ctrl Pts',(110.557702779899,0.763910315589563,150.80692281406));
#92600=CARTESIAN_POINT('Ctrl Pts',(110.548682698323,0.766030849290375,150.823268798254));
#92601=CARTESIAN_POINT('Ctrl Pts',(110.538777594462,0.768362981190624,150.839142111502));
#92602=CARTESIAN_POINT('Ctrl Pts',(110.528130734865,0.770874226858077,150.854580670989));
#92603=CARTESIAN_POINT('Ctrl Pts',(110.522606361851,0.77217724561878,150.862591329967));
#92604=CARTESIAN_POINT('Ctrl Pts',(110.516916289504,0.773520734835112,150.87044028587));
#92605=CARTESIAN_POINT('Ctrl Pts',(110.511065300135,0.774903837338248,150.8781534036));
#92606=CARTESIAN_POINT('Ctrl Pts',(110.49675000416,0.778287798655982,150.897024667283));
#92607=CARTESIAN_POINT('Ctrl Pts',(110.481490408537,0.781904580009331,150.91504702297));
#92608=CARTESIAN_POINT('Ctrl Pts',(110.465697924213,0.785659761757801,150.932146675738));
#92609=CARTESIAN_POINT('Ctrl Pts',(110.462737064113,0.786363803476632,150.935352610825));
#92610=CARTESIAN_POINT('Ctrl Pts',(110.459756910977,0.787072836516795,150.938527001465));
#92611=CARTESIAN_POINT('Ctrl Pts',(110.456750103519,0.787788631045777,150.94167972859));
#92612=CARTESIAN_POINT('Ctrl Pts',(110.439536415148,0.791886487037215,150.959728793256));
#92613=CARTESIAN_POINT('Ctrl Pts',(110.42152783605,0.796187304544596,150.976987704495));
#92614=CARTESIAN_POINT('Ctrl Pts',(110.40290188466,0.800652170714823,150.993568951696));
#92615=CARTESIAN_POINT('Ctrl Pts',(110.383199066548,0.805375174882903,151.011108850242));
#92616=CARTESIAN_POINT('Ctrl Pts',(110.362805198615,0.810281780069283,151.027890437271));
#92617=CARTESIAN_POINT('Ctrl Pts',(110.341874993262,0.815338382011048,151.044029963927));
#92618=CARTESIAN_POINT('Ctrl Pts',(110.330744571933,0.81802741965561,151.052612762266));
#92619=CARTESIAN_POINT('Ctrl Pts',(110.319461583996,0.820759078031207,151.061013710925));
#92620=CARTESIAN_POINT('Ctrl Pts',(110.308043818064,0.823529558586245,151.069248554519));
#92621=CARTESIAN_POINT('Ctrl Pts',(110.282997151361,0.829607043751403,151.087312980089));
#92622=CARTESIAN_POINT('Ctrl Pts',(110.25753240075,0.835815613704716,151.104421923017));
#92623=CARTESIAN_POINT('Ctrl Pts',(110.231691500055,0.842147539981722,151.120755955339));
#92624=CARTESIAN_POINT('Ctrl Pts',(110.213993989033,0.846484050399732,151.131942551365));
#92625=CARTESIAN_POINT('Ctrl Pts',(110.196119026854,0.850878666513219,151.142764962505));
#92626=CARTESIAN_POINT('Ctrl Pts',(110.178068985415,0.855331688375319,151.15327329781));
#92627=CARTESIAN_POINT('Ctrl Pts',(110.144029566785,0.863729357479973,151.173090295226));
#92628=CARTESIAN_POINT('Ctrl Pts',(110.109390729821,0.872329659079962,151.191779430376));
#92629=CARTESIAN_POINT('Ctrl Pts',(110.074302136121,0.881101259647679,151.209539849258));
#92630=CARTESIAN_POINT('Ctrl Pts',(110.052320079445,0.886596430598848,151.220666272213));
#92631=CARTESIAN_POINT('Ctrl Pts',(110.030160566118,0.892159045199865,151.231427543411));
#92632=CARTESIAN_POINT('Ctrl Pts',(110.007852155919,0.89778332038,151.241866826161));
#92633=CARTESIAN_POINT('Ctrl Pts',(109.970500956097,0.907200101953821,151.259345424256));
#92634=CARTESIAN_POINT('Ctrl Pts',(109.932631685714,0.916816594981333,151.275928634357));
#92635=CARTESIAN_POINT('Ctrl Pts',(109.894447290657,0.926582979000112,151.291691334144));
#92636=CARTESIAN_POINT('Ctrl Pts',(109.852384741436,0.937341274578199,151.309054954405));
#92637=CARTESIAN_POINT('Ctrl Pts',(109.809939438207,0.948281505647227,151.325423210272));
#92638=CARTESIAN_POINT('Ctrl Pts',(109.767319628914,0.959353905644784,151.3408783142));
#92639=CARTESIAN_POINT('Ctrl Pts',(109.732213376733,0.968474323427329,151.35360879763));
#92640=CARTESIAN_POINT('Ctrl Pts',(109.696987178204,0.977684816576761,151.365719377932));
#92641=CARTESIAN_POINT('Ctrl Pts',(109.661733986723,0.986964195335185,151.377246386361));
#92642=CARTESIAN_POINT('Ctrl Pts',(109.614572865747,0.99937799067772,151.392667022513));
#92643=CARTESIAN_POINT('Ctrl Pts',(109.567209175688,1.01195382312556,151.407140915232));
#92644=CARTESIAN_POINT('Ctrl Pts',(109.519520623797,1.02472635764171,151.420776182521));
#92645=CARTESIAN_POINT('Ctrl Pts',(109.446484320137,1.0442878388033,151.441658962196));
#92646=CARTESIAN_POINT('Ctrl Pts',(109.37301201643,1.0642323371024,151.460485446871));
#92647=CARTESIAN_POINT('Ctrl Pts',(109.299170657915,1.08455251676184,151.477473436277));
#92648=CARTESIAN_POINT('Ctrl Pts',(109.220851198854,1.10610501133885,151.495491660314));
#92649=CARTESIAN_POINT('Ctrl Pts',(109.142116222202,1.12808011914536,151.511441624991));
#92650=CARTESIAN_POINT('Ctrl Pts',(109.063009522562,1.1504815767125,151.525536766875));
#92651=CARTESIAN_POINT('Ctrl Pts',(109.012011299796,1.16492326785228,151.534623572278));
#92652=CARTESIAN_POINT('Ctrl Pts',(108.960857865818,1.17954240781536,151.542938554077));
#92653=CARTESIAN_POINT('Ctrl Pts',(108.909554859704,1.1943425298468,151.550529724418));
#92654=CARTESIAN_POINT('Ctrl Pts',(108.882458423677,1.20215943162696,151.554539112505));
#92655=CARTESIAN_POINT('Ctrl Pts',(108.855384688227,1.21000775512804,151.558336010665));
#92656=CARTESIAN_POINT('Ctrl Pts',(108.828326358283,1.21788960972175,151.561922431859));
#92657=CARTESIAN_POINT('Ctrl Pts',(108.625188701118,1.2770618306088,151.588847123828));
#92658=CARTESIAN_POINT('Ctrl Pts',(108.421787066927,1.33847795579103,151.604069000832));
#92659=CARTESIAN_POINT('Ctrl Pts',(108.21817335316,1.40225878138333,151.607501729799));
#92660=CARTESIAN_POINT('Ctrl Pts',(108.188568310647,1.41153239079901,151.608000841991));
#92661=CARTESIAN_POINT('Ctrl Pts',(108.158958780341,1.4208560027417,151.608250635593));
#92662=CARTESIAN_POINT('Ctrl Pts',(108.129344917475,1.43023000148885,151.608250755144));
#92663=CARTESIAN_POINT('Ctrl Pts',(190.5,51.8013867006572,41.));
#92664=CARTESIAN_POINT('Ctrl Pts',(190.5,51.8013867006572,40.));
#92665=CARTESIAN_POINT('Ctrl Pts',(189.5,51.8013867006572,40.));
#92666=CARTESIAN_POINT('Ctrl Pts',(190.5,49.0776276471086,41.));
#92667=CARTESIAN_POINT('Ctrl Pts',(190.500000000443,49.077627647157,40.));
#92668=CARTESIAN_POINT('Ctrl Pts',(189.500000000443,49.1436388962432,40.));
#92669=CARTESIAN_POINT('Ctrl Pts',(190.230148217333,46.3947031958517,41.));
#92670=CARTESIAN_POINT('Ctrl Pts',(190.230148217548,46.3947031957874,40.));
#92671=CARTESIAN_POINT('Ctrl Pts',(189.236843327146,46.5338535505999,40.));
#92672=CARTESIAN_POINT('Ctrl Pts',(189.361745789355,42.4483454229149,41.));
#92673=CARTESIAN_POINT('Ctrl Pts',(189.361745789248,42.4483454229471,40.));
#92674=CARTESIAN_POINT('Ctrl Pts',(188.393447405239,42.7011350513066,40.));
#92675=CARTESIAN_POINT('Ctrl Pts',(188.994929796133,41.145948626321,41.));
#92676=CARTESIAN_POINT('Ctrl Pts',(188.994929796263,41.1459486262754,40.));
#92677=CARTESIAN_POINT('Ctrl Pts',(188.03743539513,41.4372314385205,40.));
#92678=CARTESIAN_POINT('Ctrl Pts',(188.320848581514,39.2146325226266,41.));
#92679=CARTESIAN_POINT('Ctrl Pts',(188.320848581448,39.2146325226495,40.));
#92680=CARTESIAN_POINT('Ctrl Pts',(187.383379063071,39.5632888051564,40.));
#92681=CARTESIAN_POINT('Ctrl Pts',(188.07440016264,38.5721075764589,41.0000000000092));
#92682=CARTESIAN_POINT('Ctrl Pts',(188.07440016258,38.5721075764866,40.0000000000138));
#92683=CARTESIAN_POINT('Ctrl Pts',(187.144269963878,38.939897855964,40.));
#92684=CARTESIAN_POINT('Ctrl Pts',(187.545929721486,37.3110698530063,40.9999999999908));
#92685=CARTESIAN_POINT('Ctrl Pts',(187.545929721547,37.3110698529785,39.9999999999862));
#92686=CARTESIAN_POINT('Ctrl Pts',(186.631487670084,37.7162952356469,40.));
#92687=CARTESIAN_POINT('Ctrl Pts',(187.263906551726,36.6919462209565,41.));
#92688=CARTESIAN_POINT('Ctrl Pts',(187.263906551658,36.6919462209899,40.));
#92689=CARTESIAN_POINT('Ctrl Pts',(186.357812851989,37.1154901542486,40.));
#92690=CARTESIAN_POINT('Ctrl Pts',(185.76842343351,33.6516773356634,41.));
#92691=CARTESIAN_POINT('Ctrl Pts',(185.768423433782,33.6516773355295,40.));
#92692=CARTESIAN_POINT('Ctrl Pts',(184.906205569059,34.1644194244269,40.));
#92693=CARTESIAN_POINT('Ctrl Pts',(184.299478625402,31.3966159998617,41.0000000000366));
#92694=CARTESIAN_POINT('Ctrl Pts',(184.299478625217,31.3966160000255,40.0000000000549));
#92695=CARTESIAN_POINT('Ctrl Pts',(183.479162611529,31.9726430192458,40.0000000000001));
#92696=CARTESIAN_POINT('Ctrl Pts',(182.174203530724,28.7729657639328,40.9999999999909));
#92697=CARTESIAN_POINT('Ctrl Pts',(182.174203530771,28.7729657638918,39.9999999999864));
#92698=CARTESIAN_POINT('Ctrl Pts',(181.407974125944,29.4157626542651,40.0000000000001));
#92699=CARTESIAN_POINT('Ctrl Pts',(181.734653162829,28.2579931028748,41.));
#92700=CARTESIAN_POINT('Ctrl Pts',(181.734653162795,28.2579931029011,39.9999999999931));
#92701=CARTESIAN_POINT('Ctrl Pts',(180.979331279132,28.9135514351784,40.0000000000001));
#92702=CARTESIAN_POINT('Ctrl Pts',(180.827681669059,27.246908681366,41.));
#92703=CARTESIAN_POINT('Ctrl Pts',(180.827681669093,27.2469086813396,40.0000000000069));
#92704=CARTESIAN_POINT('Ctrl Pts',(180.094217491189,27.9268338056749,40.0000000000001));
#92705=CARTESIAN_POINT('Ctrl Pts',(180.360725912636,26.7514671965533,40.9999999999908));
#92706=CARTESIAN_POINT('Ctrl Pts',(180.36072591255,26.7514671966354,39.9999999999862));
#92707=CARTESIAN_POINT('Ctrl Pts',(179.63819831998,27.4429796616177,40.));
#92708=CARTESIAN_POINT('Ctrl Pts',(178.935911835944,25.3077730343987,41.0000000000183));
#92709=CARTESIAN_POINT('Ctrl Pts',(178.935911836115,25.3077730342345,40.0000000000275));
#92710=CARTESIAN_POINT('Ctrl Pts',(178.245730718942,26.0320605949285,40.));
#92711=CARTESIAN_POINT('Ctrl Pts',(177.949212299624,24.3963507756892,41.0000000000183));
#92712=CARTESIAN_POINT('Ctrl Pts',(177.949212299508,24.3963507758324,40.0000000000274));
#92713=CARTESIAN_POINT('Ctrl Pts',(177.280088553843,25.1399810127014,40.0000000000001));
#92714=CARTESIAN_POINT('Ctrl Pts',(174.895556188476,21.7926966511935,40.9999999999637));
#92715=CARTESIAN_POINT('Ctrl Pts',(174.895556188708,21.7926966509072,39.9999999999455));
#92716=CARTESIAN_POINT('Ctrl Pts',(174.287368474715,22.5882830821278,40.0000000000001));
#92717=CARTESIAN_POINT('Ctrl Pts',(172.735872865175,20.2300058704473,41.));
#92718=CARTESIAN_POINT('Ctrl Pts',(172.735872865024,20.2300058706094,39.9999999999818));
#92719=CARTESIAN_POINT('Ctrl Pts',(172.165255517355,21.0522193748322,40.0000000000001));
#92720=CARTESIAN_POINT('Ctrl Pts',(169.356441294098,18.0818577291379,41.));
#92721=CARTESIAN_POINT('Ctrl Pts',(169.356441294173,18.0818577290568,40.0000000000092));
#92722=CARTESIAN_POINT('Ctrl Pts',(168.837076511978,18.9366501155665,40.0000000000001));
#92723=CARTESIAN_POINT('Ctrl Pts',(168.204655946576,17.3977933717527,41.));
#92724=CARTESIAN_POINT('Ctrl Pts',(168.204655946514,17.3977933718631,40.));
#92725=CARTESIAN_POINT('Ctrl Pts',(167.701570963275,18.2622113948054,40.));
#92726=CARTESIAN_POINT('Ctrl Pts',(165.867055390467,16.0921286981499,41.));
#92727=CARTESIAN_POINT('Ctrl Pts',(165.867055390528,16.0921286980395,40.));
#92728=CARTESIAN_POINT('Ctrl Pts',(165.394862835991,16.973801659069,40.));
#92729=CARTESIAN_POINT('Ctrl Pts',(164.686884180974,15.473505799436,40.9999999999817));
#92730=CARTESIAN_POINT('Ctrl Pts',(164.686884180934,15.4735057995083,39.9999999999726));
#92731=CARTESIAN_POINT('Ctrl Pts',(164.229235699794,16.3627715090405,39.9999999999999));
#92732=CARTESIAN_POINT('Ctrl Pts',(161.117211964886,13.7051879643896,41.0000000000364));
#92733=CARTESIAN_POINT('Ctrl Pts',(161.117211964965,13.705187964245,40.0000000000546));
#92734=CARTESIAN_POINT('Ctrl Pts',(160.700828996284,14.6148954782875,39.9999999999999));
#92735=CARTESIAN_POINT('Ctrl Pts',(158.698784431002,12.6423350514952,40.9999999998913));
#92736=CARTESIAN_POINT('Ctrl Pts',(158.698784430949,12.6423350515778,39.999999999837));
#92737=CARTESIAN_POINT('Ctrl Pts',(158.306770084267,13.5625992022113,40.0000000000001));
#92738=CARTESIAN_POINT('Ctrl Pts',(153.802915982434,10.6924687335121,41.0000000001088));
#92739=CARTESIAN_POINT('Ctrl Pts',(153.802915982487,10.6924687334295,40.0000000001631));
#92740=CARTESIAN_POINT('Ctrl Pts',(153.454924546975,11.6302657880098,40.0000000000001));
#92741=CARTESIAN_POINT('Ctrl Pts',(151.325348981608,9.80582682032301,40.9999999999275));
#92742=CARTESIAN_POINT('Ctrl Pts',(151.32534898167,9.80582682007378,39.9999999998913));
#92743=CARTESIAN_POINT('Ctrl Pts',(150.997001969331,10.7505714530412,40.0000000000001));
#92744=CARTESIAN_POINT('Ctrl Pts',(148.824154304563,8.98894875990613,41.));
#92745=CARTESIAN_POINT('Ctrl Pts',(148.824154304563,8.98894875990614,40.0000000000001));
#92746=CARTESIAN_POINT('Ctrl Pts',(148.513697082188,9.93953611153414,40.0000000000001));
#92747=CARTESIAN_POINT('',(189.5,51.8013867006572,40.));
#92748=CARTESIAN_POINT('',(190.5,51.8013867006572,41.));
#92749=CARTESIAN_POINT('Origin',(189.5,51.8013867006572,41.));
#92750=CARTESIAN_POINT('Ctrl Pts',(148.824154304563,8.98894875990614,41.));
#92751=CARTESIAN_POINT('Ctrl Pts',(151.374396929587,9.82184564245748,41.));
#92752=CARTESIAN_POINT('Ctrl Pts',(153.894322991189,10.7254588349369,41.));
#92753=CARTESIAN_POINT('Ctrl Pts',(158.858378723721,12.7094876159781,41.));
#92754=CARTESIAN_POINT('Ctrl Pts',(161.302641161874,13.7895935121803,41.));
#92755=CARTESIAN_POINT('Ctrl Pts',(164.895576805134,15.5811002632408,41.));
#92756=CARTESIAN_POINT('Ctrl Pts',(166.080912343717,16.2069826871151,41.));
#92757=CARTESIAN_POINT('Ctrl Pts',(168.423049908267,17.5253047067075,41.));
#92758=CARTESIAN_POINT('Ctrl Pts',(169.573365929323,18.214181934056,41.));
#92759=CARTESIAN_POINT('Ctrl Pts',(172.947104141466,20.3771647370291,41.));
#92760=CARTESIAN_POINT('Ctrl Pts',(175.097030815196,21.948091086913,41.));
#92761=CARTESIAN_POINT('Ctrl Pts',(178.127203245858,24.5574879603648,41.));
#92762=CARTESIAN_POINT('Ctrl Pts',(179.104620116965,25.4696986671831,41.));
#92763=CARTESIAN_POINT('Ctrl Pts',(180.513665800821,26.9121814463635,41.));
#92764=CARTESIAN_POINT('Ctrl Pts',(180.975042758687,27.4068420809117,41.));
#92765=CARTESIAN_POINT('Ctrl Pts',(181.868856334096,28.4135619078113,41.));
#92766=CARTESIAN_POINT('Ctrl Pts',(182.301682749673,28.9258761071667,41.));
#92767=CARTESIAN_POINT('Ctrl Pts',(184.393047680122,31.533722716317,41.));
#92768=CARTESIAN_POINT('Ctrl Pts',(185.833875349279,33.7677063786469,41.));
#92769=CARTESIAN_POINT('Ctrl Pts',(187.301196170355,36.77240822161,41.));
#92770=CARTESIAN_POINT('Ctrl Pts',(187.577936119931,37.3839842039535,41.));
#92771=CARTESIAN_POINT('Ctrl Pts',(188.096717650489,38.629202283799,41.));
#92772=CARTESIAN_POINT('Ctrl Pts',(188.338665411654,39.2629767077245,41.));
#92773=CARTESIAN_POINT('Ctrl Pts',(189.004582545503,41.1792956133264,41.));
#92774=CARTESIAN_POINT('Ctrl Pts',(189.371588131973,42.4864580865601,41.));
#92775=CARTESIAN_POINT('Ctrl Pts',(190.234410487385,46.4275807179081,41.));
#92776=CARTESIAN_POINT('Ctrl Pts',(190.5,49.0966280990945,41.));
#92777=CARTESIAN_POINT('Ctrl Pts',(190.5,51.8013867006572,41.));
#92778=CARTESIAN_POINT('Ctrl Pts',(189.5,51.8013867006572,40.));
#92779=CARTESIAN_POINT('Ctrl Pts',(189.500000000381,49.5150063958733,40.));
#92780=CARTESIAN_POINT('Ctrl Pts',(189.305251220874,47.2641771162462,39.9999999999999));
#92781=CARTESIAN_POINT('Ctrl Pts',(188.892871196549,45.0530760686969,40.0000000000001));
#92782=CARTESIAN_POINT('Ctrl Pts',(188.826741633494,44.6985022835477,40.0000000000001));
#92783=CARTESIAN_POINT('Ctrl Pts',(188.755015452642,44.3449501511665,40.0000000000002));
#92784=CARTESIAN_POINT('Ctrl Pts',(188.677598163273,43.9924369200007,40.0000000000002));
#92785=CARTESIAN_POINT('Ctrl Pts',(188.676593078966,43.9878603516488,40.0000000000002));
#92786=CARTESIAN_POINT('Ctrl Pts',(188.675587035428,43.9832839585214,40.0000000000002));
#92787=CARTESIAN_POINT('Ctrl Pts',(188.674580032453,43.9787077406567,40.0000000000002));
#92788=CARTESIAN_POINT('Ctrl Pts',(188.394958895188,42.7079992378199,40.0000000000004));
#92789=CARTESIAN_POINT('Ctrl Pts',(188.041258879596,41.4508135433267,40.));
#92790=CARTESIAN_POINT('Ctrl Pts',(187.60841945111,40.2080747459915,40.));
#92791=CARTESIAN_POINT('Ctrl Pts',(187.60608126682,40.2013615120737,40.));
#92792=CARTESIAN_POINT('Ctrl Pts',(187.603740773219,40.1946486981984,40.));
#92793=CARTESIAN_POINT('Ctrl Pts',(187.601397969504,40.1879363045588,40.));
#92794=CARTESIAN_POINT('Ctrl Pts',(187.386112555457,39.5711196097217,40.));
#92795=CARTESIAN_POINT('Ctrl Pts',(187.150262439701,38.9555155944513,40.0000000000113));
#92796=CARTESIAN_POINT('Ctrl Pts',(186.897516139808,38.3511109250051,40.0000000000038));
#92797=CARTESIAN_POINT('Ctrl Pts',(186.894307237426,38.3434373187688,40.0000000000037));
#92798=CARTESIAN_POINT('Ctrl Pts',(186.891095610294,38.3357655101271,40.0000000000036));
#92799=CARTESIAN_POINT('Ctrl Pts',(186.887881265928,38.328095519511,40.0000000000035));
#92800=CARTESIAN_POINT('Ctrl Pts',(186.635165548002,37.7250713987454,39.9999999999965));
#92801=CARTESIAN_POINT('Ctrl Pts',(186.365651623061,37.1327088502353,40.));
#92802=CARTESIAN_POINT('Ctrl Pts',(186.079960250839,36.5506519989377,40.));
#92803=CARTESIAN_POINT('Ctrl Pts',(186.07580740624,36.5421911496209,40.));
#92804=CARTESIAN_POINT('Ctrl Pts',(186.071651142412,36.5337324756742,40.));
#92805=CARTESIAN_POINT('Ctrl Pts',(186.067491461228,36.5252759759054,40.));
#92806=CARTESIAN_POINT('Ctrl Pts',(184.912445383137,34.1771039736579,40.));
#92807=CARTESIAN_POINT('Ctrl Pts',(183.494489308755,31.9961998873436,39.999999999999));
#92808=CARTESIAN_POINT('Ctrl Pts',(181.848901150115,29.9601216086773,40.0000000000012));
#92809=CARTESIAN_POINT('Ctrl Pts',(181.840011734412,29.9491227775739,40.0000000000012));
#92810=CARTESIAN_POINT('Ctrl Pts',(181.831115675126,29.9381281731419,40.0000000000012));
#92811=CARTESIAN_POINT('Ctrl Pts',(181.822212977855,29.9271377918265,40.0000000000012));
#92812=CARTESIAN_POINT('Ctrl Pts',(181.417620189473,29.4276679248657,40.0000000000016));
#92813=CARTESIAN_POINT('Ctrl Pts',(180.999283430905,28.9369421095781,40.0000000000001));
#92814=CARTESIAN_POINT('Ctrl Pts',(180.567663620525,28.4546672424251,40.0000000000001));
#92815=CARTESIAN_POINT('Ctrl Pts',(180.557374801756,28.4431709241716,40.0000000000001));
#92816=CARTESIAN_POINT('Ctrl Pts',(180.547078402794,28.4316793699371,40.0000000000001));
#92817=CARTESIAN_POINT('Ctrl Pts',(180.536774431889,28.4201925785101,40.0000000000001));
#92818=CARTESIAN_POINT('Ctrl Pts',(180.105311565568,27.9392009298139,40.0000000000001));
#92819=CARTESIAN_POINT('Ctrl Pts',(179.660998793274,27.4671830454874,40.0000000000089));
#92820=CARTESIAN_POINT('Ctrl Pts',(179.208941172121,27.0080712980567,40.0000000000045));
#92821=CARTESIAN_POINT('Ctrl Pts',(179.19731416185,26.9962628542807,40.0000000000044));
#92822=CARTESIAN_POINT('Ctrl Pts',(179.185681914772,26.9844628235726,40.0000000000043));
#92823=CARTESIAN_POINT('Ctrl Pts',(179.174044515442,26.9726712705521,40.0000000000042));
#92824=CARTESIAN_POINT('Ctrl Pts',(178.499085028626,26.2887709978425,39.999999999998));
#92825=CARTESIAN_POINT('Ctrl Pts',(177.804262150814,25.6304014524943,39.9999999999994));
#92826=CARTESIAN_POINT('Ctrl Pts',(177.091787308052,24.9950133496928,40.0000000000011));
#92827=CARTESIAN_POINT('Ctrl Pts',(176.838514100436,24.7691432231717,40.0000000000016));
#92828=CARTESIAN_POINT('Ctrl Pts',(176.583010542457,24.5461768349467,40.0000000000027));
#92829=CARTESIAN_POINT('Ctrl Pts',(176.325376910205,24.325998452793,40.0000000000056));
#92830=CARTESIAN_POINT('Ctrl Pts',(176.311096984169,24.3137945686019,40.0000000000057));
#92831=CARTESIAN_POINT('Ctrl Pts',(176.296810486525,24.3015992278323,40.0000000000059));
#92832=CARTESIAN_POINT('Ctrl Pts',(176.282517433164,24.2894124098309,40.0000000000061));
#92833=CARTESIAN_POINT('Ctrl Pts',(174.305240624492,22.6035086356279,40.0000000000279));
#92834=CARTESIAN_POINT('Ctrl Pts',(172.203250088958,21.0797419335985,39.9999999999525));
#92835=CARTESIAN_POINT('Ctrl Pts',(170.006058541585,19.6797512754289,40.0000000000483));
#92836=CARTESIAN_POINT('Ctrl Pts',(169.98620495979,19.6671011134178,40.0000000000492));
#92837=CARTESIAN_POINT('Ctrl Pts',(169.96634374653,19.6544611562793,40.00000000005));
#92838=CARTESIAN_POINT('Ctrl Pts',(169.946474915949,19.6418313700356,40.0000000000508));
#92839=CARTESIAN_POINT('Ctrl Pts',(169.265312398142,19.2088447902787,40.0000000000772));
#92840=CARTESIAN_POINT('Ctrl Pts',(168.57446714291,18.7875560756054,40.0000000000313));
#92841=CARTESIAN_POINT('Ctrl Pts',(167.875526707261,18.3776388152218,40.0000000000131));
#92842=CARTESIAN_POINT('Ctrl Pts',(167.458565391396,18.1330977476744,40.0000000000022));
#92843=CARTESIAN_POINT('Ctrl Pts',(167.038722359307,17.8926044574574,40.0000000000005));
#92844=CARTESIAN_POINT('Ctrl Pts',(166.616329946493,17.6560969384847,40.0000000000003));
#92845=CARTESIAN_POINT('Ctrl Pts',(166.593633120015,17.6433884476215,40.0000000000002));
#92846=CARTESIAN_POINT('Ctrl Pts',(166.570928868342,17.6306914358825,40.0000000000002));
#92847=CARTESIAN_POINT('Ctrl Pts',(166.54821725046,17.6180058988327,40.0000000000002));
#92848=CARTESIAN_POINT('Ctrl Pts',(165.41908891768,16.9873331139122,39.9999999999997));
#92849=CARTESIAN_POINT('Ctrl Pts',(164.277098272627,16.3878383790561,39.9999999999967));
#92850=CARTESIAN_POINT('Ctrl Pts',(163.123421206771,15.8150185333796,40.0000000000032));
#92851=CARTESIAN_POINT('Ctrl Pts',(163.099985980906,15.8033825540742,40.0000000000034));
#92852=CARTESIAN_POINT('Ctrl Pts',(163.076546021088,15.7917576290974,40.0000000000035));
#92853=CARTESIAN_POINT('Ctrl Pts',(163.053101341965,15.7801437228353,40.0000000000036));
#92854=CARTESIAN_POINT('Ctrl Pts',(161.986099857154,15.2515779377907,40.0000000000097));
#92855=CARTESIAN_POINT('Ctrl Pts',(160.909372419548,14.7457024936771,40.0000000000103));
#92856=CARTESIAN_POINT('Ctrl Pts',(159.823918020749,14.2601912942237,40.0000000000086));
#92857=CARTESIAN_POINT('Ctrl Pts',(158.70516141636,13.7597844033452,40.0000000000068));
#92858=CARTESIAN_POINT('Ctrl Pts',(157.577134187948,13.2810103531194,40.0000000000028));
#92859=CARTESIAN_POINT('Ctrl Pts',(156.440948827796,12.8212705536111,40.0000000000148));
#92860=CARTESIAN_POINT('Ctrl Pts',(156.270965230959,12.7524893252391,40.0000000000166));
#92861=CARTESIAN_POINT('Ctrl Pts',(156.100799064079,12.6841340486979,40.0000000000189));
#92862=CARTESIAN_POINT('Ctrl Pts',(155.930454085978,12.6161959298486,40.000000000022));
#92863=CARTESIAN_POINT('Ctrl Pts',(155.913921012608,12.6096020993987,40.0000000000223));
#92864=CARTESIAN_POINT('Ctrl Pts',(155.897386254016,12.6030121998952,40.0000000000226));
#92865=CARTESIAN_POINT('Ctrl Pts',(155.880849813508,12.5964262232311,40.0000000000228));
#92866=CARTESIAN_POINT('Ctrl Pts',(154.560886364425,12.0707237016309,40.0000000000461));
#92867=CARTESIAN_POINT('Ctrl Pts',(153.23016485382,11.5701212714179,40.0000000000271));
#92868=CARTESIAN_POINT('Ctrl Pts',(151.889842870709,11.0919212256656,40.0000000000128));
#92869=CARTESIAN_POINT('Ctrl Pts',(150.770923688729,10.6927132661168,40.0000000000009));
#92870=CARTESIAN_POINT('Ctrl Pts',(149.645314177788,10.3091167708951,40.0000000000001));
#92871=CARTESIAN_POINT('Ctrl Pts',(148.513697082188,9.9395361115339,40.0000000000001));
#92872=CARTESIAN_POINT('Origin',(149.134611526938,8.03836140827812,150.608250755187));
#92873=CARTESIAN_POINT('',(148.824154304613,8.98894875992246,150.608250755187));
#92874=CARTESIAN_POINT('Origin',(149.134611526927,8.03836140827455,150.608250755186));
#92875=CARTESIAN_POINT('',(148.824154304563,8.98894875990614,150.608250755187));
#92876=CARTESIAN_POINT('Origin',(125.29348064571,25.4505574462982,152.608250755187));
#92877=CARTESIAN_POINT('',(95.8129088738133,23.8757620423259,151.608250755187));
#92878=CARTESIAN_POINT('Origin',(95.8129088738133,23.8757620423259,152.608250755187));
#92879=CARTESIAN_POINT('Origin',(125.29348064571,25.4505574462982,151.608250755187));
#92880=CARTESIAN_POINT('Origin',(189.5,59.,41.));
#92881=CARTESIAN_POINT('',(189.5,51.8013867006572,40.));
#92882=CARTESIAN_POINT('',(190.5,54.9,41.));
#92883=CARTESIAN_POINT('Ctrl Pts',(150.890053008323,10.740031424167,151.608250755187));
#92884=CARTESIAN_POINT('Ctrl Pts',(150.023036902254,11.238311537975,151.608250755187));
#92885=CARTESIAN_POINT('Ctrl Pts',(150.023036902254,11.238311537975,152.608250755187));
#92886=CARTESIAN_POINT('Ctrl Pts',(150.679848671071,10.5466203837958,151.608250755187));
#92887=CARTESIAN_POINT('Ctrl Pts',(149.898373926292,11.0213957787624,151.690671913218));
#92888=CARTESIAN_POINT('Ctrl Pts',(149.856007771352,10.9476779311712,152.608250750006));
#92889=CARTESIAN_POINT('Ctrl Pts',(150.469500865012,10.3582448836075,151.58941017031));
#92890=CARTESIAN_POINT('Ctrl Pts',(149.756882065769,10.7815385921042,151.738129573559));
#92891=CARTESIAN_POINT('Ctrl Pts',(149.686939041021,10.6653465091927,152.570569586968));
#92892=CARTESIAN_POINT('Ctrl Pts',(150.049234791875,9.99119406960843,151.515506211375));
#92893=CARTESIAN_POINT('Ctrl Pts',(149.461299151908,10.2989599789586,151.749878235574));
#92894=CARTESIAN_POINT('Ctrl Pts',(149.345761369004,10.1165733930159,152.422761666028));
#92895=CARTESIAN_POINT('Ctrl Pts',(149.836710770193,9.81044310313042,151.459547614775));
#92896=CARTESIAN_POINT('Ctrl Pts',(149.304412653593,10.0509204841014,151.718712252751));
#92897=CARTESIAN_POINT('Ctrl Pts',(149.17146532147,9.8470577724018,152.310844478137));
#92898=CARTESIAN_POINT('Ctrl Pts',(149.43689869125,9.477996755743,151.305510205471));
#92899=CARTESIAN_POINT('Ctrl Pts',(149.002736057782,9.5899170411257,151.566756275077));
#92900=CARTESIAN_POINT('Ctrl Pts',(148.840879579051,9.35250297616965,152.002769651981));
#92901=CARTESIAN_POINT('Ctrl Pts',(149.244022866828,9.32177597503067,151.206172324202));
#92902=CARTESIAN_POINT('Ctrl Pts',(148.851344778941,9.36640628955775,151.448241697994));
#92903=CARTESIAN_POINT('Ctrl Pts',(148.679929727225,9.12075031956211,151.80409390049));
#92904=CARTESIAN_POINT('Ctrl Pts',(149.013179253012,9.13764052726729,151.012654819751));
#92905=CARTESIAN_POINT('Ctrl Pts',(148.668260894911,9.10226279678571,151.186102695064));
#92906=CARTESIAN_POINT('Ctrl Pts',(148.486316262615,8.84803681808999,151.41705888068));
#92907=CARTESIAN_POINT('Ctrl Pts',(148.946252751058,9.08480391731076,150.940166521214));
#92908=CARTESIAN_POINT('Ctrl Pts',(148.614853057507,9.02629227892066,151.085099511553));
#92909=CARTESIAN_POINT('Ctrl Pts',(148.429993799101,8.76987161641128,151.272082289649));
#92910=CARTESIAN_POINT('Ctrl Pts',(148.851443947787,9.01024718564305,150.781805962456));
#92911=CARTESIAN_POINT('Ctrl Pts',(148.539419389592,8.91959726288131,150.860017320521));
#92912=CARTESIAN_POINT('Ctrl Pts',(148.350106592124,8.65962177792194,150.955361167317));
#92913=CARTESIAN_POINT('Ctrl Pts',(148.824154321238,8.98894876535212,150.695048022002));
#92914=CARTESIAN_POINT('Ctrl Pts',(148.517388962888,8.88876069858572,150.733964227236));
#92915=CARTESIAN_POINT('Ctrl Pts',(148.327056364841,8.62815345652074,150.78184529078));
#92916=CARTESIAN_POINT('Ctrl Pts',(148.824154304563,8.98894875990614,150.608250755186));
#92917=CARTESIAN_POINT('Ctrl Pts',(148.517388951131,8.88876068209877,150.608250755186));
#92918=CARTESIAN_POINT('Ctrl Pts',(148.327056352437,8.62815343953653,150.608250755186));
#92919=CARTESIAN_POINT('',(150.890034276198,10.7400141885713,151.608250755137));
#92920=CARTESIAN_POINT('Origin',(150.890053008323,10.740031424167,152.608250755187));
#92921=CARTESIAN_POINT('Ctrl Pts',(150.890034276198,10.7400141885713,151.608250755137));
#92922=CARTESIAN_POINT('Ctrl Pts',(150.702220874324,10.5672055383393,151.60824975506));
#92923=CARTESIAN_POINT('Ctrl Pts',(150.513515802512,10.3977022423503,151.593212219756));
#92924=CARTESIAN_POINT('Ctrl Pts',(150.32404987297,10.2313684559334,151.563261500175));
#92925=CARTESIAN_POINT('Ctrl Pts',(150.302482255713,10.2124340572738,151.55985209745));
#92926=CARTESIAN_POINT('Ctrl Pts',(150.28092156319,10.1935549579782,151.556251950677));
#92927=CARTESIAN_POINT('Ctrl Pts',(150.259359907948,10.1747237977009,151.552460508724));
#92928=CARTESIAN_POINT('Ctrl Pts',(150.196877948972,10.1201543423087,151.541473563708));
#92929=CARTESIAN_POINT('Ctrl Pts',(150.134156936491,10.0658027349855,151.528804384371));
#92930=CARTESIAN_POINT('Ctrl Pts',(150.07139188021,10.0118119412705,151.51433719755));
#92931=CARTESIAN_POINT('Ctrl Pts',(150.015325641343,9.96358350149239,151.501414071211));
#92932=CARTESIAN_POINT('Ctrl Pts',(149.959223383041,9.9156424153212,151.487055826325));
#92933=CARTESIAN_POINT('Ctrl Pts',(149.903238759799,9.86810887537708,151.471148343347));
#92934=CARTESIAN_POINT('Ctrl Pts',(149.85352379096,9.82589856261102,151.457022321329));
#92935=CARTESIAN_POINT('Ctrl Pts',(149.803901299349,9.7840094868303,151.441674307829));
#92936=CARTESIAN_POINT('Ctrl Pts',(149.754498021731,9.74254510422443,151.425002834105));
#92937=CARTESIAN_POINT('Ctrl Pts',(149.715112765934,9.70948889026117,151.411712010322));
#92938=CARTESIAN_POINT('Ctrl Pts',(149.675856770622,9.67669314558932,151.397575569593));
#92939=CARTESIAN_POINT('Ctrl Pts',(149.636803961062,9.6442201983715,151.382529318118));
#92940=CARTESIAN_POINT('Ctrl Pts',(149.594993458305,9.60945419140713,151.366420583668));
#92941=CARTESIAN_POINT('Ctrl Pts',(149.553169819802,9.57485906888988,151.349214625101));
#92942=CARTESIAN_POINT('Ctrl Pts',(149.51159298729,9.54063089633836,151.330765820964));
#92943=CARTESIAN_POINT('Ctrl Pts',(149.498919450395,9.53019739331577,151.325142217968));
#92944=CARTESIAN_POINT('Ctrl Pts',(149.48626910023,9.51979819119965,151.319402992941));
#92945=CARTESIAN_POINT('Ctrl Pts',(149.473650016671,9.50943941894691,151.313543636607));
#92946=CARTESIAN_POINT('Ctrl Pts',(149.440007168315,9.48182262709181,151.297922420085));
#92947=CARTESIAN_POINT('Ctrl Pts',(149.406484061281,9.45440888248824,151.281402363808));
#92948=CARTESIAN_POINT('Ctrl Pts',(149.373220289311,9.42730489399397,151.263853428368));
#92949=CARTESIAN_POINT('Ctrl Pts',(149.342132586372,9.401974010187,151.247452519526));
#92950=CARTESIAN_POINT('Ctrl Pts',(149.311271225832,9.3769135727762,151.23015290458));
#92951=CARTESIAN_POINT('Ctrl Pts',(149.280781733949,9.352236209495,151.211831178815));
#92952=CARTESIAN_POINT('Ctrl Pts',(149.254017698261,9.33057412886442,151.19574815178));
#92953=CARTESIAN_POINT('Ctrl Pts',(149.227540417594,9.30920741102851,151.178877360186));
#92954=CARTESIAN_POINT('Ctrl Pts',(149.201472558853,9.28823154460514,151.161123285777));
#92955=CARTESIAN_POINT('Ctrl Pts',(149.178745519636,9.26994391524619,151.145644548172));
#92956=CARTESIAN_POINT('Ctrl Pts',(149.156284165708,9.25191801548321,151.129467025821));
#92957=CARTESIAN_POINT('Ctrl Pts',(149.134140819759,9.23419340628573,151.112465523864));
#92958=CARTESIAN_POINT('Ctrl Pts',(149.119315419052,9.2223264357599,151.101082687697));
#92959=CARTESIAN_POINT('Ctrl Pts',(149.10463318418,9.21059503744752,151.089330111665));
#92960=CARTESIAN_POINT('Ctrl Pts',(149.090119188631,9.19901878583329,151.077164926928));
#92961=CARTESIAN_POINT('Ctrl Pts',(149.072065293653,9.18461913756459,151.062032707349));
#92962=CARTESIAN_POINT('Ctrl Pts',(149.054284809231,9.1704676159025,151.04623098932));
#92963=CARTESIAN_POINT('Ctrl Pts',(149.036925482486,9.15667686664026,151.029695222165));
#92964=CARTESIAN_POINT('Ctrl Pts',(149.020628290217,9.14372990760409,151.014171199799));
#92965=CARTESIAN_POINT('Ctrl Pts',(149.004702141776,9.1311008202778,150.998000123864));
#92966=CARTESIAN_POINT('Ctrl Pts',(148.989304616076,9.11891023333167,150.981123519122));
#92967=CARTESIAN_POINT('Ctrl Pts',(148.978126890576,9.11006056246756,150.968872066593));
#92968=CARTESIAN_POINT('Ctrl Pts',(148.967228418988,9.10144250223408,150.956248701183));
#92969=CARTESIAN_POINT('Ctrl Pts',(148.956683203421,9.09311277673819,150.943229559169));
#92970=CARTESIAN_POINT('Ctrl Pts',(148.94495349998,9.08384741756284,150.928748046306));
#92971=CARTESIAN_POINT('Ctrl Pts',(148.933584378101,9.07489430584278,150.913728163051));
#92972=CARTESIAN_POINT('Ctrl Pts',(148.922730874631,9.06635281780613,150.898085641888));
#92973=CARTESIAN_POINT('Ctrl Pts',(148.917030133927,9.06186645000287,150.889869496995));
#92974=CARTESIAN_POINT('Ctrl Pts',(148.911472216629,9.05749419673198,150.881481585143));
#92975=CARTESIAN_POINT('Ctrl Pts',(148.906083889309,9.05325444445017,150.872909874024));
#92976=CARTESIAN_POINT('Ctrl Pts',(148.903614104637,9.05131111870578,150.868980958893));
#92977=CARTESIAN_POINT('Ctrl Pts',(148.901179323965,9.04939580803512,150.865014674827));
#92978=CARTESIAN_POINT('Ctrl Pts',(148.898781146499,9.04750992291207,150.86100941786));
#92979=CARTESIAN_POINT('Ctrl Pts',(148.890200772378,9.04076246567011,150.846679117571));
#92980=CARTESIAN_POINT('Ctrl Pts',(148.882105340252,9.03440329935373,150.831820967099));
#92981=CARTESIAN_POINT('Ctrl Pts',(148.874581296409,9.02850640119304,150.816392770031));
#92982=CARTESIAN_POINT('Ctrl Pts',(148.870885359862,9.02560974589988,150.808814180834));
#92983=CARTESIAN_POINT('Ctrl Pts',(148.867327896282,9.02282506859138,150.801098019324));
#92984=CARTESIAN_POINT('Ctrl Pts',(148.863922930779,9.02016392556131,150.793239294057));
#92985=CARTESIAN_POINT('Ctrl Pts',(148.8577859103,9.015367551189,150.779074933838));
#92986=CARTESIAN_POINT('Ctrl Pts',(148.852233457605,9.01101353123725,150.764504006908));
#92987=CARTESIAN_POINT('Ctrl Pts',(148.847355686723,9.00718402694656,150.749595709683));
#92988=CARTESIAN_POINT('Ctrl Pts',(148.839939029894,9.00136126080139,150.726927624791));
#92989=CARTESIAN_POINT('Ctrl Pts',(148.834072242688,8.99674936577631,150.703484221276));
#92990=CARTESIAN_POINT('Ctrl Pts',(148.830097384467,8.99362376040685,150.679507686099));
#92991=CARTESIAN_POINT('Ctrl Pts',(148.82622971412,8.99058244156457,150.656177713313));
#92992=CARTESIAN_POINT('Ctrl Pts',(148.824154304567,8.98894875990739,150.63234387459));
#92993=CARTESIAN_POINT('Ctrl Pts',(148.824154304563,8.98894875990613,150.608250755187));
#92994=CARTESIAN_POINT('Origin',(95.8129088738133,23.8757620423259,152.608250755187));
#92995=CARTESIAN_POINT('',(95.8129088738133,24.8757620423259,152.608250755187));
#92996=CARTESIAN_POINT('Origin',(95.8129088738133,23.8757620423259,152.608250755187));
#92997=CARTESIAN_POINT('Origin',(95.8129088738133,23.8757620423259,152.608250755187));
#92998=CARTESIAN_POINT('Origin',(125.29348064571,25.4505574462982,152.608250755187));
#92999=CARTESIAN_POINT('',(154.774052417606,23.8757620423259,151.608250755187));
#93000=CARTESIAN_POINT('Origin',(154.774052417606,23.8757620423259,152.608250755187));
#93001=CARTESIAN_POINT('Origin',(125.29348064571,25.4505574462982,151.608250755187));
#93002=CARTESIAN_POINT('Origin',(95.8129088738133,23.8757620423259,200.));
#93003=CARTESIAN_POINT('',(95.8129088734846,24.8757620423263,194.272015611497));
#93004=CARTESIAN_POINT('Origin',(95.8129088738133,23.8757620423259,194.272013743528));
#93005=CARTESIAN_POINT('',(95.8129088738133,24.8757620423259,209.282162333937));
#93006=CARTESIAN_POINT('Origin',(154.774052417606,23.8757620423259,152.608250755187));
#93007=CARTESIAN_POINT('',(154.774052417606,24.8757620423259,152.608250755187));
#93008=CARTESIAN_POINT('Origin',(154.774052417606,23.8757620423259,152.608250755187));
#93009=CARTESIAN_POINT('Origin',(154.774052417606,23.8757620423259,152.608250755187));
#93010=CARTESIAN_POINT('Ctrl Pts',(95.8129088738133,24.8757620423259,194.272013743528));
#93011=CARTESIAN_POINT('Ctrl Pts',(96.7609165275083,24.8757620423259,194.272013743528));
#93012=CARTESIAN_POINT('Ctrl Pts',(96.8114851745877,23.9291040663932,194.272013743528));
#93013=CARTESIAN_POINT('Ctrl Pts',(95.8079727953211,24.8757620423259,194.394449674887));
#93014=CARTESIAN_POINT('Ctrl Pts',(96.7606658729216,24.8804543649553,194.400983611462));
#93015=CARTESIAN_POINT('Ctrl Pts',(96.8114851740455,23.9291040765447,194.51649042457));
#93016=CARTESIAN_POINT('Ctrl Pts',(95.8006244305256,24.8980341121937,194.515591412477));
#93017=CARTESIAN_POINT('Ctrl Pts',(96.760522851172,24.910116493455,194.526658900505));
#93018=CARTESIAN_POINT('Ctrl Pts',(96.8090937438902,23.9721393953228,194.758275720961));
#93019=CARTESIAN_POINT('Ctrl Pts',(95.7873179138766,24.9635088171672,194.687547735987));
#93020=CARTESIAN_POINT('Ctrl Pts',(96.7608130482612,24.986259065464,194.698633486749));
#93021=CARTESIAN_POINT('Ctrl Pts',(96.8029028333402,24.098653234827,195.101372403818));
#93022=CARTESIAN_POINT('Ctrl Pts',(95.7826072263359,24.9902403040083,194.74214852889));
#93023=CARTESIAN_POINT('Ctrl Pts',(96.7609969780626,25.0165323795395,194.752374177845));
#93024=CARTESIAN_POINT('Ctrl Pts',(96.8004649444392,24.1503052933488,195.210295541072));
#93025=CARTESIAN_POINT('Ctrl Pts',(95.7729687455057,25.0532515622315,194.846058360888));
#93026=CARTESIAN_POINT('Ctrl Pts',(96.7615918607211,25.0855066901878,194.852621305907));
#93027=CARTESIAN_POINT('Ctrl Pts',(96.7951694477337,24.2720591317408,195.417558574747));
#93028=CARTESIAN_POINT('Ctrl Pts',(95.7679900091412,25.0899771867542,194.895826418653));
#93029=CARTESIAN_POINT('Ctrl Pts',(96.7620107784742,25.1247157442461,194.899520222782));
#93030=CARTESIAN_POINT('Ctrl Pts',(96.7922803023377,24.3430224150016,195.516813717754));
#93031=CARTESIAN_POINT('Ctrl Pts',(95.7584833321546,25.1712173600468,194.987060242779));
#93032=CARTESIAN_POINT('Ctrl Pts',(96.7630842785473,25.2087962452066,194.983645143531));
#93033=CARTESIAN_POINT('Ctrl Pts',(96.7866131605335,24.4999991676107,195.698751372675));
#93034=CARTESIAN_POINT('Ctrl Pts',(95.7539645643008,25.2155346348072,195.028519785351));
#93035=CARTESIAN_POINT('Ctrl Pts',(96.7637357976572,25.2535048092381,195.020845409791));
#93036=CARTESIAN_POINT('Ctrl Pts',(96.7838438654193,24.5856314571151,195.781421806259));
#93037=CARTESIAN_POINT('Ctrl Pts',(95.7457923218438,25.3114864345674,195.10320966763));
#93038=CARTESIAN_POINT('Ctrl Pts',(96.7652338888118,25.3476725061538,195.086601753473));
#93039=CARTESIAN_POINT('Ctrl Pts',(96.7788223919801,24.7710348316154,195.930352581545));
#93040=CARTESIAN_POINT('Ctrl Pts',(95.7421172576637,25.3636687358292,195.136650236237));
#93041=CARTESIAN_POINT('Ctrl Pts',(96.7660895466707,25.3976087993447,195.115261771168));
#93042=CARTESIAN_POINT('Ctrl Pts',(96.7765574337878,24.8718643595615,195.997032176725));
#93043=CARTESIAN_POINT('Ctrl Pts',(95.7333832975172,25.5258065749971,195.22061596659));
#93044=CARTESIAN_POINT('Ctrl Pts',(96.7687559909472,25.5496067281877,195.186532790236));
#93045=CARTESIAN_POINT('Ctrl Pts',(96.7713474235503,25.1851560562777,196.164477575663));
#93046=CARTESIAN_POINT('Ctrl Pts',(95.7304688922887,25.6430766735032,195.256533916462));
#93047=CARTESIAN_POINT('Ctrl Pts',(96.7706567312437,25.6544438350804,195.215613536792));
#93048=CARTESIAN_POINT('Ctrl Pts',(96.7699131986613,25.4117499178439,196.23613851731));
#93049=CARTESIAN_POINT('Ctrl Pts',(95.7316383541684,25.7661094150365,195.270070553806));
#93050=CARTESIAN_POINT('Ctrl Pts',(96.7723664237184,25.763493773239,195.227911042172));
#93051=CARTESIAN_POINT('Ctrl Pts',(96.7715712560824,25.6494824928011,196.263237066376));
#93052=CARTESIAN_POINT('',(95.731638354191,25.7661094150387,195.270070553806));
#93053=CARTESIAN_POINT('Origin',(95.7715955767732,25.6564567877472,196.263237066376));
#93054=CARTESIAN_POINT('Ctrl Pts',(95.8129087986265,24.8757620423276,194.272015608479));
#93055=CARTESIAN_POINT('Ctrl Pts',(95.8111599846757,24.8757621224561,194.315393480133));
#93056=CARTESIAN_POINT('Ctrl Pts',(95.8091170484719,24.8785534558019,194.358408096338));
#93057=CARTESIAN_POINT('Ctrl Pts',(95.8068203772479,24.8840451859619,194.400933950253));
#93058=CARTESIAN_POINT('Ctrl Pts',(95.8045026574643,24.8895872467953,194.443849545618));
#93059=CARTESIAN_POINT('Ctrl Pts',(95.8019264129473,24.8978795127077,194.486268093549));
#93060=CARTESIAN_POINT('Ctrl Pts',(95.7991270967733,24.9088812271481,194.528059904604));
#93061=CARTESIAN_POINT('Ctrl Pts',(95.79682015952,24.9179478217431,194.562500846539));
#93062=CARTESIAN_POINT('Ctrl Pts',(95.7943615808282,24.9288555341911,194.596516310934));
#93063=CARTESIAN_POINT('Ctrl Pts',(95.7917690076823,24.9416074763769,194.630028143149));
#93064=CARTESIAN_POINT('Ctrl Pts',(95.7917638288634,24.941632949139,194.630095085025));
#93065=CARTESIAN_POINT('Ctrl Pts',(95.7917586495273,24.9416584291797,194.630162024657));
#93066=CARTESIAN_POINT('Ctrl Pts',(95.7917534696742,24.9416839164987,194.630228962045));
#93067=CARTESIAN_POINT('Ctrl Pts',(95.787316972302,24.9635135747863,194.687560229433));
#93068=CARTESIAN_POINT('Ctrl Pts',(95.7826068075667,24.9902431242573,194.74215317923));
#93069=CARTESIAN_POINT('Ctrl Pts',(95.7777879962155,25.0217459334254,194.794103444976));
#93070=CARTESIAN_POINT('Ctrl Pts',(95.7729914787601,25.0531029970358,194.845813366426));
#93071=CARTESIAN_POINT('Ctrl Pts',(95.7680367191655,25.0896312250587,194.895360130286));
#93072=CARTESIAN_POINT('Ctrl Pts',(95.7633016033217,25.1300430217835,194.940820367825));
#93073=CARTESIAN_POINT('Ctrl Pts',(95.7632799654491,25.1302276899813,194.941028105684));
#93074=CARTESIAN_POINT('Ctrl Pts',(95.7632583319708,25.1304124409499,194.941235760046));
#93075=CARTESIAN_POINT('Ctrl Pts',(95.7632367029239,25.1305972745647,194.941443330717));
#93076=CARTESIAN_POINT('Ctrl Pts',(95.7584926044537,25.1711385372072,194.986971721539));
#93077=CARTESIAN_POINT('Ctrl Pts',(95.7539707476346,25.2154626761908,195.028463770006));
#93078=CARTESIAN_POINT('Ctrl Pts',(95.7498784975762,25.263510536673,195.065864725834));
#93079=CARTESIAN_POINT('Ctrl Pts',(95.7457948977628,25.3114568330366,195.103186623092));
#93080=CARTESIAN_POINT('Ctrl Pts',(95.7421178281146,25.3636590503685,195.136645218593));
#93081=CARTESIAN_POINT('Ctrl Pts',(95.7392059782138,25.4177146834181,195.164638812005));
#93082=CARTESIAN_POINT('Ctrl Pts',(95.7362880075347,25.4718839427025,195.192691248621));
#93083=CARTESIAN_POINT('Ctrl Pts',(95.7341019804868,25.5283457376407,195.215693951352));
#93084=CARTESIAN_POINT('Ctrl Pts',(95.7327939124058,25.5865853949566,195.233353660436));
#93085=CARTESIAN_POINT('Ctrl Pts',(95.7315641209546,25.6413399094394,195.249956587743));
#93086=CARTESIAN_POINT('Ctrl Pts',(95.7311104577768,25.6976651602042,195.261836989884));
#93087=CARTESIAN_POINT('Ctrl Pts',(95.7315446396439,25.7551239438692,195.268800596824));
#93088=CARTESIAN_POINT('Ctrl Pts',(95.7315722754624,25.7587812143241,195.269243832693));
#93089=CARTESIAN_POINT('Ctrl Pts',(95.7316035045552,25.7624430757672,195.269667166021));
#93090=CARTESIAN_POINT('Ctrl Pts',(95.731638354173,25.7661094150365,195.270070553806));
#93091=CARTESIAN_POINT('Origin',(154.774052417606,23.8757620423259,200.));
#93092=CARTESIAN_POINT('',(154.774052417606,24.8757620428585,184.081718857687));
#93093=CARTESIAN_POINT('Origin',(154.774052417606,23.8757620423259,184.081718857688));
#93094=CARTESIAN_POINT('',(154.774052417606,24.8757620423259,209.282162333937));
#93095=CARTESIAN_POINT('Ctrl Pts',(95.7316383541684,25.7661094150367,195.270070553806));
#93096=CARTESIAN_POINT('Ctrl Pts',(96.7723664237184,25.7634937732391,195.227911042172));
#93097=CARTESIAN_POINT('Ctrl Pts',(96.7715712560824,25.6494824928014,196.263237066376));
#93098=CARTESIAN_POINT('Ctrl Pts',(95.7431185671264,26.8818810097605,195.392797778142));
#93099=CARTESIAN_POINT('Ctrl Pts',(96.7843087616111,26.8373701392618,195.349876958745));
#93100=CARTESIAN_POINT('Ctrl Pts',(96.779337565007,26.7630172805684,196.390166135436));
#93101=CARTESIAN_POINT('Ctrl Pts',(95.8218441751224,27.9971373813779,195.450206233717));
#93102=CARTESIAN_POINT('Ctrl Pts',(96.8559141943711,27.9051069966177,195.411323729247));
#93103=CARTESIAN_POINT('Ctrl Pts',(96.8521036068265,27.8758205758653,196.449663888928));
#93104=CARTESIAN_POINT('Ctrl Pts',(95.9690444983148,29.1114187506901,195.445834017246));
#93105=CARTESIAN_POINT('Ctrl Pts',(96.9905454909872,28.9836527494144,195.415492891841));
#93106=CARTESIAN_POINT('Ctrl Pts',(96.9910158671794,28.9874167683923,196.445393189885));
#93107=CARTESIAN_POINT('',(95.9690447990561,29.111418071869,195.445834751564));
#93108=CARTESIAN_POINT('Origin',(95.9987338969782,29.1114187506901,196.445393189885));
#93109=CARTESIAN_POINT('Ctrl Pts',(95.7316383541731,25.7661094150388,195.270070553806));
#93110=CARTESIAN_POINT('Ctrl Pts',(95.7406061566686,26.6376977150264,195.365939290139));
#93111=CARTESIAN_POINT('Ctrl Pts',(95.790599427845,27.508471439827,195.421899098602));
#93112=CARTESIAN_POINT('Ctrl Pts',(95.882078879369,28.3783025745837,195.439761788028));
#93113=CARTESIAN_POINT('Ctrl Pts',(95.9077872007393,28.6227498026515,195.444781710564));
#93114=CARTESIAN_POINT('Ctrl Pts',(95.9367721585806,28.8671225938835,195.446792581224));
#93115=CARTESIAN_POINT('Ctrl Pts',(95.9690444149639,29.1114181197373,195.445834019721));
#93116=CARTESIAN_POINT('Ctrl Pts',(154.442742286491,25.4284918940124,185.219477651476));
#93117=CARTESIAN_POINT('Ctrl Pts',(153.817575691237,25.3176612644957,185.442322230393));
#93118=CARTESIAN_POINT('Ctrl Pts',(153.812479229217,24.9971192497071,186.033932954978));
#93119=CARTESIAN_POINT('Ctrl Pts',(154.472026398247,25.2558401938721,185.111373906101));
#93120=CARTESIAN_POINT('Ctrl Pts',(153.818074697533,25.110693010453,185.299575711385));
#93121=CARTESIAN_POINT('Ctrl Pts',(153.807172637763,24.6633611425982,185.846711293107));
#93122=CARTESIAN_POINT('Ctrl Pts',(154.516058475459,25.1137033968244,184.943001574196));
#93123=CARTESIAN_POINT('Ctrl Pts',(153.817447383613,24.9564514213952,185.077611618409));
#93124=CARTESIAN_POINT('Ctrl Pts',(153.796905931419,24.388867509514,185.554961769222));
#93125=CARTESIAN_POINT('Ctrl Pts',(154.600746940777,24.9716430335893,184.644296030959));
#93126=CARTESIAN_POINT('Ctrl Pts',(153.818898801799,24.8420834669797,184.714743312115));
#93127=CARTESIAN_POINT('Ctrl Pts',(153.784915835979,24.1143706192211,185.041138096643));
#93128=CARTESIAN_POINT('Ctrl Pts',(154.632378374674,24.9354624397147,184.535985737446));
#93129=CARTESIAN_POINT('Ctrl Pts',(153.819796875227,24.8226658090599,184.584352025953));
#93130=CARTESIAN_POINT('Ctrl Pts',(153.781441235691,24.0444604764696,184.855381098777));
#93131=CARTESIAN_POINT('Ctrl Pts',(154.699685066687,24.8878568443247,184.31420127492));
#93132=CARTESIAN_POINT('Ctrl Pts',(153.822398663114,24.8213877551996,184.328869994504));
#93133=CARTESIAN_POINT('Ctrl Pts',(153.776752125358,23.9524743105778,184.476529617814));
#93134=CARTESIAN_POINT('Ctrl Pts',(154.735994047269,24.8757620423259,184.1985843258));
#93135=CARTESIAN_POINT('Ctrl Pts',(153.824151134487,24.8403128253378,184.200581623196));
#93136=CARTESIAN_POINT('Ctrl Pts',(153.775476116835,23.9291040664471,184.279754424779));
#93137=CARTESIAN_POINT('Ctrl Pts',(154.774052417606,24.8757620423259,184.081718857687));
#93138=CARTESIAN_POINT('Ctrl Pts',(153.826044763911,24.8757620423257,184.081718857687));
#93139=CARTESIAN_POINT('Ctrl Pts',(153.775476116832,23.9291040663932,184.081718857688));
#93140=CARTESIAN_POINT('',(154.442742286966,25.4284918937499,185.219477651102));
#93141=CARTESIAN_POINT('Origin',(154.812352855916,24.9812217457127,186.033932954964));
#93142=CARTESIAN_POINT('Ctrl Pts',(154.44274228656,25.4284918936062,185.219477651221));
#93143=CARTESIAN_POINT('Ctrl Pts',(154.448284212903,25.3958180921978,185.19901935167));
#93144=CARTESIAN_POINT('Ctrl Pts',(154.454281299807,25.364663906821,185.176674057838));
#93145=CARTESIAN_POINT('Ctrl Pts',(154.460687448475,25.3350161332536,185.152758299799));
#93146=CARTESIAN_POINT('Ctrl Pts',(154.467312158215,25.3043568550406,185.128026598523));
#93147=CARTESIAN_POINT('Ctrl Pts',(154.474374329022,25.2753083237004,185.101615189071));
#93148=CARTESIAN_POINT('Ctrl Pts',(154.481831864672,25.2478538641296,185.073818892769));
#93149=CARTESIAN_POINT('Ctrl Pts',(154.489693131172,25.2189130942252,185.044517780015));
#93150=CARTESIAN_POINT('Ctrl Pts',(154.497993712757,25.1917434060434,185.013677634679));
#93151=CARTESIAN_POINT('Ctrl Pts',(154.506694089653,25.1663266839483,184.981586326707));
#93152=CARTESIAN_POINT('Ctrl Pts',(154.5156826416,25.1400681057713,184.948432086124));
#93153=CARTESIAN_POINT('Ctrl Pts',(154.525097929767,25.1156802398802,184.913942042753));
#93154=CARTESIAN_POINT('Ctrl Pts',(154.534906494078,25.0931489773896,184.878378268025));
#93155=CARTESIAN_POINT('Ctrl Pts',(154.545184815804,25.0695386346909,184.841111252502));
#93156=CARTESIAN_POINT('Ctrl Pts',(154.555894981686,25.047966594657,184.802664857134));
#93157=CARTESIAN_POINT('Ctrl Pts',(154.567009342758,25.0284284402446,184.763286335916));
#93158=CARTESIAN_POINT('Ctrl Pts',(154.56882939591,25.0252289329324,184.756837831931));
#93159=CARTESIAN_POINT('Ctrl Pts',(154.570660310709,25.0220839992451,184.750364225634));
#93160=CARTESIAN_POINT('Ctrl Pts',(154.572501991839,25.0189936596592,184.743866482733));
#93161=CARTESIAN_POINT('Ctrl Pts',(154.575023733311,25.0147621793188,184.73496937917));
#93162=CARTESIAN_POINT('Ctrl Pts',(154.577568015069,25.0106275870193,184.726018641299));
#93163=CARTESIAN_POINT('Ctrl Pts',(154.580133819563,25.0065893890237,184.717018488867));
#93164=CARTESIAN_POINT('Ctrl Pts',(154.591777703693,24.9882636320624,184.676174873404));
#93165=CARTESIAN_POINT('Ctrl Pts',(154.603854224587,24.9719426858168,184.634361233353));
#93166=CARTESIAN_POINT('Ctrl Pts',(154.616261722143,24.9575932362401,184.591988610101));
#93167=CARTESIAN_POINT('Ctrl Pts',(154.62935435389,24.9424514191077,184.547276197316));
#93168=CARTESIAN_POINT('Ctrl Pts',(154.642815578117,24.9295046365609,184.501941061476));
#93169=CARTESIAN_POINT('Ctrl Pts',(154.656540518755,24.9187250131128,184.456411390074));
#93170=CARTESIAN_POINT('Ctrl Pts',(154.659684720487,24.9162555444567,184.445981146663));
#93171=CARTESIAN_POINT('Ctrl Pts',(154.662842817589,24.9138998617083,184.435540489566));
#93172=CARTESIAN_POINT('Ctrl Pts',(154.666013643873,24.9116577244602,184.425094219679));
#93173=CARTESIAN_POINT('Ctrl Pts',(154.681690213016,24.9005725950782,184.373447848185));
#93174=CARTESIAN_POINT('Ctrl Pts',(154.697814213832,24.8921152784088,184.321202826052));
#93175=CARTESIAN_POINT('Ctrl Pts',(154.714295347124,24.8861977637108,184.268661979121));
#93176=CARTESIAN_POINT('Ctrl Pts',(154.731628586706,24.8799743021214,184.213404669348));
#93177=CARTESIAN_POINT('Ctrl Pts',(154.749356958483,24.8765597521334,184.157819589899));
#93178=CARTESIAN_POINT('Ctrl Pts',(154.767390788052,24.8758861536974,184.102216495425));
#93179=CARTESIAN_POINT('Ctrl Pts',(154.769606753279,24.8758033831076,184.095384085071));
#93180=CARTESIAN_POINT('Ctrl Pts',(154.771827347406,24.8757620423259,184.088551359106));
#93181=CARTESIAN_POINT('Ctrl Pts',(154.774052417606,24.8757620423259,184.081718857687));
#93182=CARTESIAN_POINT('Ctrl Pts',(95.9690444983151,29.1114187506925,195.445834017246));
#93183=CARTESIAN_POINT('Ctrl Pts',(96.9905454909875,28.9836527494168,195.415492891841));
#93184=CARTESIAN_POINT('Ctrl Pts',(96.9910158671796,28.9874167683946,196.445393189885));
#93185=CARTESIAN_POINT('Ctrl Pts',(96.1808469360716,30.8083310983659,195.439542956962));
#93186=CARTESIAN_POINT('Ctrl Pts',(97.1949838327504,30.6213702247017,195.409160016061));
#93187=CARTESIAN_POINT('Ctrl Pts',(97.1958901734581,30.6268508847717,196.43909456317));
#93188=CARTESIAN_POINT('Ctrl Pts',(96.5357039062144,32.4621522990289,195.428958375868));
#93189=CARTESIAN_POINT('Ctrl Pts',(97.5375062160773,32.2174773037551,195.398506678642));
#93190=CARTESIAN_POINT('Ctrl Pts',(97.5391410311521,32.2246530909199,196.428497216997));
#93191=CARTESIAN_POINT('Ctrl Pts',(97.2734769439721,34.8806495075041,195.406087214197));
#93192=CARTESIAN_POINT('Ctrl Pts',(98.2495553841758,34.5514785375348,195.375526283764));
#93193=CARTESIAN_POINT('Ctrl Pts',(98.2528123253432,34.5612301109138,196.405597550267));
#93194=CARTESIAN_POINT('Ctrl Pts',(97.5538509175081,35.6764000718443,195.397285235172));
#93195=CARTESIAN_POINT('Ctrl Pts',(98.5201541771945,35.3194365450969,195.366686752647));
#93196=CARTESIAN_POINT('Ctrl Pts',(98.5240305654619,35.3300267321143,196.396784487269));
#93197=CARTESIAN_POINT('Ctrl Pts',(98.18431282738,37.2468200580182,195.377069023014));
#93198=CARTESIAN_POINT('Ctrl Pts',(99.12861500334,36.8350067634597,195.346402562534));
#93199=CARTESIAN_POINT('Ctrl Pts',(99.1339182696851,36.8472528999435,196.376542353047));
#93200=CARTESIAN_POINT('Ctrl Pts',(98.5352221250904,38.0231116098076,195.365628086643));
#93201=CARTESIAN_POINT('Ctrl Pts',(99.467269260868,37.584178042332,195.334931117862));
#93202=CARTESIAN_POINT('Ctrl Pts',(99.4733823025719,37.5972496311567,196.365086544997));
#93203=CARTESIAN_POINT('Ctrl Pts',(99.6908456903027,40.308852455946,195.326983759774));
#93204=CARTESIAN_POINT('Ctrl Pts',(100.58251136751,39.7901098462954,195.296224400173));
#93205=CARTESIAN_POINT('Ctrl Pts',(100.591345561039,39.8055670589042,196.326390874288));
#93206=CARTESIAN_POINT('Ctrl Pts',(100.581425535931,41.7447648678172,195.296060783275));
#93207=CARTESIAN_POINT('Ctrl Pts',(101.441852730532,41.1757850798975,195.265300953242));
#93208=CARTESIAN_POINT('Ctrl Pts',(101.452939744803,41.1928417403813,196.295425589375));
#93209=CARTESIAN_POINT('Ctrl Pts',(102.090446775052,43.7718345514203,195.239992129605));
#93210=CARTESIAN_POINT('Ctrl Pts',(102.897968356158,43.1322235416134,195.209383242826));
#93211=CARTESIAN_POINT('Ctrl Pts',(102.912967222459,43.1512498063651,196.239275391062));
#93212=CARTESIAN_POINT('Ctrl Pts',(102.622478624349,44.4262693750096,195.219675251719));
#93213=CARTESIAN_POINT('Ctrl Pts',(103.411299657064,43.7638416825715,195.189144427864));
#93214=CARTESIAN_POINT('Ctrl Pts',(103.427743450085,43.7835173833033,196.218928280365));
#93215=CARTESIAN_POINT('Ctrl Pts',(103.464637936624,45.3755996946146,195.186370350926));
#93216=CARTESIAN_POINT('Ctrl Pts',(104.223880926985,44.680177009279,195.15601221913));
#93217=CARTESIAN_POINT('Ctrl Pts',(104.242626300959,44.7006916523046,196.185572234913));
#93218=CARTESIAN_POINT('Ctrl Pts',(103.752719651255,45.6866487784825,195.174795965706));
#93219=CARTESIAN_POINT('Ctrl Pts',(104.501829185358,44.9804130395041,195.144505518144));
#93220=CARTESIAN_POINT('Ctrl Pts',(104.521383391689,45.0012047721157,196.173979831597));
#93221=CARTESIAN_POINT('Ctrl Pts',(104.343828694018,46.2977922800091,195.150621120664));
#93222=CARTESIAN_POINT('Ctrl Pts',(105.072143291029,45.5703390039032,195.120488733774));
#93223=CARTESIAN_POINT('Ctrl Pts',(105.093373457231,45.5916474059541,196.149766749665));
#93224=CARTESIAN_POINT('Ctrl Pts',(104.647630621959,46.5986011658697,195.137987528073));
#93225=CARTESIAN_POINT('Ctrl Pts',(105.365249074382,45.8607130300027,195.107946133969));
#93226=CARTESIAN_POINT('Ctrl Pts',(105.387356025942,45.8822671873913,196.13711288398));
#93227=CARTESIAN_POINT('Ctrl Pts',(106.193340539684,48.0640285060236,195.072510066659));
#93228=CARTESIAN_POINT('Ctrl Pts',(106.856313491502,47.2751774604217,195.042996477193));
#93229=CARTESIAN_POINT('Ctrl Pts',(106.88314578035,47.2980570568634,196.071528584548));
#93230=CARTESIAN_POINT('Ctrl Pts',(107.513689725659,49.1139724683082,195.012882323802));
#93231=CARTESIAN_POINT('Ctrl Pts',(108.129721803209,48.2887968792928,194.984003591972));
#93232=CARTESIAN_POINT('Ctrl Pts',(108.160975010984,48.3124369479142,196.011798414246));
#93233=CARTESIAN_POINT('Ctrl Pts',(109.615125126087,50.511791610423,194.909278340031));
#93234=CARTESIAN_POINT('Ctrl Pts',(110.157489415393,49.6394299207645,194.881793166221));
#93235=CARTESIAN_POINT('Ctrl Pts',(110.195027611433,49.6629086681952,195.908000630588));
#93236=CARTESIAN_POINT('Ctrl Pts',(110.335870143622,50.9480470823175,194.872368331763));
#93237=CARTESIAN_POINT('Ctrl Pts',(110.85272962471,50.0609555896405,194.845443682159));
#93238=CARTESIAN_POINT('Ctrl Pts',(110.89270788553,50.0843871411745,195.871019251302));
#93239=CARTESIAN_POINT('Ctrl Pts',(111.447804523715,51.5572270341353,194.812857830125));
#93240=CARTESIAN_POINT('Ctrl Pts',(111.925622387835,50.6499225755847,194.786916511041));
#93241=CARTESIAN_POINT('Ctrl Pts',(111.969145579328,50.6729327353859,195.811388698003));
#93242=CARTESIAN_POINT('Ctrl Pts',(111.823592422802,51.7527428674394,194.792328697466));
#93243=CARTESIAN_POINT('Ctrl Pts',(112.288148478452,50.8389588738988,194.766745695778));
#93244=CARTESIAN_POINT('Ctrl Pts',(112.332951136671,50.861825987525,195.790817373735));
#93245=CARTESIAN_POINT('Ctrl Pts',(112.585611671513,52.1284437551186,194.749769711206));
#93246=CARTESIAN_POINT('Ctrl Pts',(113.023310517829,51.2023071262054,194.724961663351));
#93247=CARTESIAN_POINT('Ctrl Pts',(113.070704237323,51.2248010026007,195.748169059864));
#93248=CARTESIAN_POINT('Ctrl Pts',(112.972600874585,52.3089265662353,194.727693914219));
#93249=CARTESIAN_POINT('Ctrl Pts',(113.396653199089,51.3769027979713,194.703305191536));
#93250=CARTESIAN_POINT('Ctrl Pts',(113.445385623426,51.3991704364259,195.726046023214));
#93251=CARTESIAN_POINT('Ctrl Pts',(114.916147013965,53.1645838313077,194.614306433195));
#93252=CARTESIAN_POINT('Ctrl Pts',(115.270541301213,52.2043876372251,194.592229587412));
#93253=CARTESIAN_POINT('Ctrl Pts',(115.327204948124,52.2258445773799,195.612410617938));
#93254=CARTESIAN_POINT('Ctrl Pts',(116.508960581184,53.7063929000131,194.51347209248));
#93255=CARTESIAN_POINT('Ctrl Pts',(116.806433549694,52.7296177887198,194.493744543161));
#93256=CARTESIAN_POINT('Ctrl Pts',(116.869699925243,52.7493012987645,195.511340071764));
#93257=CARTESIAN_POINT('Ctrl Pts',(118.952752804013,54.3121536802558,194.342894831349));
#93258=CARTESIAN_POINT('Ctrl Pts',(119.166670826541,53.3192109895653,194.327446358241));
#93259=CARTESIAN_POINT('Ctrl Pts',(119.236843055431,53.3345435367134,195.340320085676));
#93260=CARTESIAN_POINT('Ctrl Pts',(119.776496894014,54.479388232144,194.282800692507));
#93261=CARTESIAN_POINT('Ctrl Pts',(119.961612355366,53.4823273585296,194.269002235245));
#93262=CARTESIAN_POINT('Ctrl Pts',(120.034841083494,53.4961134609636,195.280063484756));
#93263=CARTESIAN_POINT('Ctrl Pts',(121.442484198752,54.7433756911386,194.155240928781));
#93264=CARTESIAN_POINT('Ctrl Pts',(121.569977744677,53.7408888473484,194.145104510391));
#93265=CARTESIAN_POINT('Ctrl Pts',(121.648970880559,53.7511590439454,195.152141272117));
#93266=CARTESIAN_POINT('Ctrl Pts',(122.287131939476,54.8401884933555,194.087563676381));
#93267=CARTESIAN_POINT('Ctrl Pts',(122.385374501015,53.8364730184404,194.079483650773));
#93268=CARTESIAN_POINT('Ctrl Pts',(122.467432995904,53.8446925471786,195.084263387053));
#93269=CARTESIAN_POINT('Ctrl Pts',(123.132502129594,54.900000000005,194.016421260282));
#93270=CARTESIAN_POINT('Ctrl Pts',(123.202778920349,53.8965577541562,194.010507093035));
#93271=CARTESIAN_POINT('Ctrl Pts',(123.286717970418,53.9024781190629,195.01289889797));
#93272=CARTESIAN_POINT('Origin',(123.216361044378,54.900000000005,195.01289889797));
#93273=CARTESIAN_POINT('Ctrl Pts',(95.9690444983151,29.1114187506925,195.445834017246));
#93274=CARTESIAN_POINT('Ctrl Pts',(96.0972458594227,30.1385385277655,195.4420261173));
#93275=CARTESIAN_POINT('Ctrl Pts',(96.2779248487746,31.1498429318702,195.436643202798));
#93276=CARTESIAN_POINT('Ctrl Pts',(96.5096309404584,32.1457528185718,195.429606506193));
#93277=CARTESIAN_POINT('Ctrl Pts',(96.6251548158192,32.6422929344827,195.426098154489));
#93278=CARTESIAN_POINT('Ctrl Pts',(96.7533634969236,33.1350069337616,195.422178692833));
#93279=CARTESIAN_POINT('Ctrl Pts',(96.8940801655196,33.6239508552454,195.417838302303));
#93280=CARTESIAN_POINT('Ctrl Pts',(96.9374041579526,33.7744874119013,195.41650197841));
#93281=CARTESIAN_POINT('Ctrl Pts',(96.9819149598591,33.9246585378549,195.415125718949));
#93282=CARTESIAN_POINT('Ctrl Pts',(97.0276077670339,34.0744669046563,195.413709226167));
#93283=CARTESIAN_POINT('Ctrl Pts',(97.2531653090372,34.813979512362,195.406716864573));
#93284=CARTESIAN_POINT('Ctrl Pts',(97.5076915903295,35.5446174058597,195.398733680154));
#93285=CARTESIAN_POINT('Ctrl Pts',(97.7915382531106,36.2664435551117,195.389659814951));
#93286=CARTESIAN_POINT('Ctrl Pts',(97.817148339291,36.3315703729101,195.38884112479));
#93287=CARTESIAN_POINT('Ctrl Pts',(97.8429971441018,36.3966254500846,195.388013554678));
#93288=CARTESIAN_POINT('Ctrl Pts',(97.869084946264,36.4616088280606,195.387177030534));
#93289=CARTESIAN_POINT('Ctrl Pts',(98.0671074803695,36.9548728102672,195.380827295525));
#93290=CARTESIAN_POINT('Ctrl Pts',(98.2792236607968,37.4446461484459,195.373951152163));
#93291=CARTESIAN_POINT('Ctrl Pts',(98.5051187984374,37.9296227062782,195.366520946132));
#93292=CARTESIAN_POINT('Ctrl Pts',(98.6387261442667,38.2164656696027,195.362126295954));
#93293=CARTESIAN_POINT('Ctrl Pts',(98.7772051355907,38.5017229381189,195.357536120521));
#93294=CARTESIAN_POINT('Ctrl Pts',(98.920447684268,38.7850162524432,195.352746052521));
#93295=CARTESIAN_POINT('Ctrl Pts',(99.1268822676556,39.193285568083,195.345842826482));
#93296=CARTESIAN_POINT('Ctrl Pts',(99.3419895912592,39.595291259492,195.338567559063));
#93297=CARTESIAN_POINT('Ctrl Pts',(99.5655235788531,39.9908276271668,195.330900660422));
#93298=CARTESIAN_POINT('Ctrl Pts',(99.9441651921826,40.6608220651446,195.317913790274));
#93299=CARTESIAN_POINT('Ctrl Pts',(100.347228042345,41.3130031012681,195.303795012562));
#93300=CARTESIAN_POINT('Ctrl Pts',(100.774291075539,41.9476732328044,195.288422771642));
#93301=CARTESIAN_POINT('Ctrl Pts',(101.036318534828,42.3370794541982,195.27899102757));
#93302=CARTESIAN_POINT('Ctrl Pts',(101.307415862361,42.71986864212,195.269086164844));
#93303=CARTESIAN_POINT('Ctrl Pts',(101.587479545813,43.0961149066845,195.258680201397));
#93304=CARTESIAN_POINT('Ctrl Pts',(102.0904180901,43.7717781924818,195.239993165493));
#93305=CARTESIAN_POINT('Ctrl Pts',(102.6224379013,44.4262190589009,195.219676863045));
#93306=CARTESIAN_POINT('Ctrl Pts',(103.183919146169,45.0591553824135,195.197471945756));
#93307=CARTESIAN_POINT('Ctrl Pts',(103.328957744289,45.2226518444957,195.191736099538));
#93308=CARTESIAN_POINT('Ctrl Pts',(103.475964910566,45.3847114464566,195.185873922911));
#93309=CARTESIAN_POINT('Ctrl Pts',(103.624955980477,45.5453229777685,195.17987985077));
#93310=CARTESIAN_POINT('Ctrl Pts',(103.76432206781,45.6955588322588,195.174273002105));
#93311=CARTESIAN_POINT('Ctrl Pts',(103.905424036428,45.8445277145151,195.168550747912));
#93312=CARTESIAN_POINT('Ctrl Pts',(104.048275195727,45.9922195364714,195.162708501344));
#93313=CARTESIAN_POINT('Ctrl Pts',(104.34381814322,46.2977772694011,195.150621551688));
#93314=CARTESIAN_POINT('Ctrl Pts',(104.647622860237,46.5985833927272,195.137987864661));
#93315=CARTESIAN_POINT('Ctrl Pts',(104.9567881871,46.8916701423301,195.124891376));
#93316=CARTESIAN_POINT('Ctrl Pts',(105.059488272285,46.9890291652721,195.120540918868));
#93317=CARTESIAN_POINT('Ctrl Pts',(105.162768415866,47.0855444753236,195.116140391019));
#93318=CARTESIAN_POINT('Ctrl Pts',(105.266626989144,47.1812182581203,195.111688523098));
#93319=CARTESIAN_POINT('Ctrl Pts',(105.7772405543,47.651591861224,195.089801219247));
#93320=CARTESIAN_POINT('Ctrl Pts',(106.301870403894,48.1015964351509,195.066671393992));
#93321=CARTESIAN_POINT('Ctrl Pts',(106.840200252243,48.5316682118175,195.042153591274));
#93322=CARTESIAN_POINT('Ctrl Pts',(106.900314316541,48.5796933445769,195.039415744258));
#93323=CARTESIAN_POINT('Ctrl Pts',(106.960599259229,48.6274699524295,195.036660588573));
#93324=CARTESIAN_POINT('Ctrl Pts',(107.021054673501,48.6749986650904,195.033887920901));
#93325=CARTESIAN_POINT('Ctrl Pts',(107.634725807791,49.1574533692965,195.005743111454));
#93326=CARTESIAN_POINT('Ctrl Pts',(108.266032185147,49.6142467316366,194.975790759413));
#93327=CARTESIAN_POINT('Ctrl Pts',(108.914698173805,50.0457741179989,194.943810465903));
#93328=CARTESIAN_POINT('Ctrl Pts',(109.538356981193,50.46066538691,194.913063067305));
#93329=CARTESIAN_POINT('Ctrl Pts',(110.178153551123,50.8520678887675,194.880429223269));
#93330=CARTESIAN_POINT('Ctrl Pts',(110.834313273343,51.2196253302198,194.845632352756));
#93331=CARTESIAN_POINT('Ctrl Pts',(110.91501763279,51.2648330546013,194.841352511964));
#93332=CARTESIAN_POINT('Ctrl Pts',(110.995966727058,51.3096789160716,194.837040097392));
#93333=CARTESIAN_POINT('Ctrl Pts',(111.077161966758,51.3541629481376,194.832694544323));
#93334=CARTESIAN_POINT('Ctrl Pts',(111.447779236129,51.5572111878583,194.812859181829));
#93335=CARTESIAN_POINT('Ctrl Pts',(111.823530943453,51.7527118271191,194.792332131191));
#93336=CARTESIAN_POINT('Ctrl Pts',(112.204602154873,51.9405930916626,194.77104919832));
#93337=CARTESIAN_POINT('Ctrl Pts',(112.432425524418,52.0529178789464,194.75832519993));
#93338=CARTESIAN_POINT('Ctrl Pts',(112.662421583518,52.1626255365207,194.745314563013));
#93339=CARTESIAN_POINT('Ctrl Pts',(112.893703680816,52.2692992869394,194.732057324778));
#93340=CARTESIAN_POINT('Ctrl Pts',(113.049130625069,52.3409865262605,194.723148152592));
#93341=CARTESIAN_POINT('Ctrl Pts',(113.20509063946,52.4112759157413,194.714130343679));
#93342=CARTESIAN_POINT('Ctrl Pts',(113.361315636869,52.4800453780003,194.705016095229));
#93343=CARTESIAN_POINT('Ctrl Pts',(113.815260557361,52.6798696608935,194.678532710005));
#93344=CARTESIAN_POINT('Ctrl Pts',(114.272332766094,52.867453125254,194.65119297123));
#93345=CARTESIAN_POINT('Ctrl Pts',(114.732715972104,53.0430471260378,194.622914824101));
#93346=CARTESIAN_POINT('Ctrl Pts',(114.830412899452,53.0803095502821,194.61691397948));
#93347=CARTESIAN_POINT('Ctrl Pts',(114.928259001973,53.11703189196,194.610870861698));
#93348=CARTESIAN_POINT('Ctrl Pts',(115.026256154282,53.1532162768944,194.604784662144));
#93349=CARTESIAN_POINT('Ctrl Pts',(115.870603102918,53.4649822240463,194.552345750391));
#93350=CARTESIAN_POINT('Ctrl Pts',(116.72569566523,53.736734200438,194.496737807013));
#93351=CARTESIAN_POINT('Ctrl Pts',(117.591372418923,53.9690295322985,194.437533206228));
#93352=CARTESIAN_POINT('Ctrl Pts',(117.773172849744,54.0178137825741,194.425099671558));
#93353=CARTESIAN_POINT('Ctrl Pts',(117.955439915971,54.0648577672854,194.412507512248));
#93354=CARTESIAN_POINT('Ctrl Pts',(118.138171848527,54.1101665523461,194.399752772408));
#93355=CARTESIAN_POINT('Ctrl Pts',(118.566636924481,54.2164054114275,194.369845790647));
#93356=CARTESIAN_POINT('Ctrl Pts',(118.997672232339,54.3130506966135,194.339041040927));
#93357=CARTESIAN_POINT('Ctrl Pts',(119.431296878576,54.4000000000098,194.307272194192));
#93358=CARTESIAN_POINT('Ctrl Pts',(151.26536469753,39.0180386085744,189.729482705023));
#93359=CARTESIAN_POINT('Ctrl Pts',(150.582709291195,38.6415601415749,189.904601964429));
#93360=CARTESIAN_POINT('Ctrl Pts',(150.625700340104,38.5584761124776,190.698119455572));
#93361=CARTESIAN_POINT('Ctrl Pts',(151.840447122378,37.9152978809689,189.581958775083));
#93362=CARTESIAN_POINT('Ctrl Pts',(151.144695308609,37.5643261489478,189.757074220131));
#93363=CARTESIAN_POINT('Ctrl Pts',(151.196085224642,37.4561565472252,190.546670641828));
#93364=CARTESIAN_POINT('Ctrl Pts',(152.330726510846,36.7970892201137,189.376750805581));
#93365=CARTESIAN_POINT('Ctrl Pts',(151.62608674106,36.4755683238397,189.554480961614));
#93366=CARTESIAN_POINT('Ctrl Pts',(151.683367009845,36.3389829613473,190.335210178467));
#93367=CARTESIAN_POINT('Ctrl Pts',(153.15652020628,34.534931176203,188.851579727408));
#93368=CARTESIAN_POINT('Ctrl Pts',(152.445883342067,34.2654524607601,189.035735458266));
#93369=CARTESIAN_POINT('Ctrl Pts',(152.505948245037,34.0798980737316,189.793027255753));
#93370=CARTESIAN_POINT('Ctrl Pts',(153.491958385796,33.390916814621,188.531634280545));
#93371=CARTESIAN_POINT('Ctrl Pts',(152.782958948242,33.1498009792059,188.721591199022));
#93372=CARTESIAN_POINT('Ctrl Pts',(152.8411749936,32.9379252989499,189.462322785582));
#93373=CARTESIAN_POINT('Ctrl Pts',(153.884219724291,31.6583920225304,187.961341908996));
#93374=CARTESIAN_POINT('Ctrl Pts',(153.185398652578,31.4484371283528,188.157455545538));
#93375=CARTESIAN_POINT('Ctrl Pts',(153.234974567374,31.209126499478,188.872431610084));
#93376=CARTESIAN_POINT('Ctrl Pts',(153.996584103503,31.0765387279129,187.75544157011));
#93377=CARTESIAN_POINT('Ctrl Pts',(153.301912221398,30.8783831037092,187.954448638106));
#93378=CARTESIAN_POINT('Ctrl Pts',(153.348167691184,30.628630919208,188.659395307684));
#93379=CARTESIAN_POINT('Ctrl Pts',(154.182311310232,29.9244074378833,187.318655130299));
#93380=CARTESIAN_POINT('Ctrl Pts',(153.497581663401,29.7478870574723,187.523076488269));
#93381=CARTESIAN_POINT('Ctrl Pts',(153.536116366461,29.4793832870787,188.20737331349));
#93382=CARTESIAN_POINT('Ctrl Pts',(154.25617142518,29.3523851374075,187.087274026207));
#93383=CARTESIAN_POINT('Ctrl Pts',(153.577375107994,29.1862055274963,187.294578964887));
#93384=CARTESIAN_POINT('Ctrl Pts',(153.611369186077,28.9088901426605,187.967875908774));
#93385=CARTESIAN_POINT('Ctrl Pts',(154.424359066069,27.6487610028378,186.35421696411));
#93386=CARTESIAN_POINT('Ctrl Pts',(153.764597828238,27.5167379078432,186.571890016881));
#93387=CARTESIAN_POINT('Ctrl Pts',(153.784512596554,27.2100871723594,187.20899762199));
#93388=CARTESIAN_POINT('Ctrl Pts',(154.465433528124,26.5295110347379,185.813820974581));
#93389=CARTESIAN_POINT('Ctrl Pts',(153.822578759736,26.4144864228749,186.037727647489));
#93390=CARTESIAN_POINT('Ctrl Pts',(153.829924819726,26.0943597881929,186.649430085873));
#93391=CARTESIAN_POINT('Ctrl Pts',(154.442742286491,25.4284918940196,185.219477651461));
#93392=CARTESIAN_POINT('Ctrl Pts',(153.817575691237,25.3176612645029,185.442322230379));
#93393=CARTESIAN_POINT('Ctrl Pts',(153.812479229218,24.9971192497146,186.033932954963));
#93394=CARTESIAN_POINT('',(151.265364697496,39.0180386085597,189.729482705031));
#93395=CARTESIAN_POINT('Origin',(151.513845774243,39.0180386085744,190.698119455572));
#93396=CARTESIAN_POINT('Ctrl Pts',(151.26536469753,39.0180386085743,189.729482705023));
#93397=CARTESIAN_POINT('Ctrl Pts',(151.840421242892,37.9153475049247,189.58196541386));
#93398=CARTESIAN_POINT('Ctrl Pts',(152.330699670202,36.797162746522,189.376767875129));
#93399=CARTESIAN_POINT('Ctrl Pts',(152.743623347839,35.6660101936194,189.114165269229));
#93400=CARTESIAN_POINT('Ctrl Pts',(152.743647418205,35.6659442558763,189.114149961459));
#93401=CARTESIAN_POINT('Ctrl Pts',(152.743671488307,35.6658783180889,189.114134653494));
#93402=CARTESIAN_POINT('Ctrl Pts',(152.743695558146,35.6658123802572,189.114119345334));
#93403=CARTESIAN_POINT('Ctrl Pts',(153.156535386619,34.5348632769377,188.851557634363));
#93404=CARTESIAN_POINT('Ctrl Pts',(153.491959356164,33.3909113019664,188.531632564244));
#93405=CARTESIAN_POINT('Ctrl Pts',(153.753465858556,32.2359002590937,188.15143938991));
#93406=CARTESIAN_POINT('Ctrl Pts',(153.75352849967,32.2356235884284,188.151348318661));
#93407=CARTESIAN_POINT('Ctrl Pts',(153.753591136563,32.2353469167625,188.151257243784));
#93408=CARTESIAN_POINT('Ctrl Pts',(153.753653769237,32.2350702440973,188.151166165279));
#93409=CARTESIAN_POINT('Ctrl Pts',(153.884328977272,31.6578274745046,187.961142302926));
#93410=CARTESIAN_POINT('Ctrl Pts',(153.996637480094,31.0762076137486,187.755316040867));
#93411=CARTESIAN_POINT('Ctrl Pts',(154.089447697742,30.5004730803946,187.537048352865));
#93412=CARTESIAN_POINT('Ctrl Pts',(154.08951285666,30.5000688766304,187.536895114496));
#93413=CARTESIAN_POINT('Ctrl Pts',(154.089578006214,30.4996646749078,187.536741869751));
#93414=CARTESIAN_POINT('Ctrl Pts',(154.089643146404,30.4992604752267,187.536588618632));
#93415=CARTESIAN_POINT('Ctrl Pts',(154.182426783275,29.9235311698206,187.318302546945));
#93416=CARTESIAN_POINT('Ctrl Pts',(154.256217688442,29.3519165206558,187.087072383857));
#93417=CARTESIAN_POINT('Ctrl Pts',(154.312233949315,28.7845104204925,186.842921679277));
#93418=CARTESIAN_POINT('Ctrl Pts',(154.312273219189,28.7841126437454,186.842750518845));
#93419=CARTESIAN_POINT('Ctrl Pts',(154.312312480344,28.7837148690555,186.842579352087));
#93420=CARTESIAN_POINT('Ctrl Pts',(154.312351732781,28.7833170964228,186.842408179003));
#93421=CARTESIAN_POINT('Ctrl Pts',(154.417517426384,27.7175989418325,186.383798791121));
#93422=CARTESIAN_POINT('Ctrl Pts',(154.460104713933,26.6666603032434,185.879784621214));
#93423=CARTESIAN_POINT('Ctrl Pts',(154.44620363346,25.6318394819492,185.328524043399));
#93424=CARTESIAN_POINT('Ctrl Pts',(154.445292156395,25.56398752995,185.292378552803));
#93425=CARTESIAN_POINT('Ctrl Pts',(154.444137804104,25.4962048746116,185.256029929632));
#93426=CARTESIAN_POINT('Ctrl Pts',(154.44274228649,25.4284918940197,185.219477651461));
#93427=CARTESIAN_POINT('Ctrl Pts',(123.159109278332,54.5824004318885,194.066403916675));
#93428=CARTESIAN_POINT('Ctrl Pts',(123.226343764611,53.8982198229655,194.291916124396));
#93429=CARTESIAN_POINT('Ctrl Pts',(123.286717970418,53.9024781190629,195.01289889797));
#93430=CARTESIAN_POINT('Ctrl Pts',(123.83865733674,54.5931791852171,194.021690234304));
#93431=CARTESIAN_POINT('Ctrl Pts',(123.882504759287,53.9459026464787,194.265746571195));
#93432=CARTESIAN_POINT('Ctrl Pts',(123.956385232616,53.9497108975491,194.954566980795));
#93433=CARTESIAN_POINT('Ctrl Pts',(124.527075444545,54.599519113683,193.966755721732));
#93434=CARTESIAN_POINT('Ctrl Pts',(124.564090549894,53.9717473179622,194.217325738079));
#93435=CARTESIAN_POINT('Ctrl Pts',(124.625450088238,53.9731815252606,194.891331888951));
#93436=CARTESIAN_POINT('Ctrl Pts',(125.893284906873,54.6002480378726,193.842179627404));
#93437=CARTESIAN_POINT('Ctrl Pts',(125.901328293953,53.974575540568,194.09392865322));
#93438=CARTESIAN_POINT('Ctrl Pts',(125.96330325035,53.9731394972598,194.76538052756));
#93439=CARTESIAN_POINT('Ctrl Pts',(126.579778542857,54.5946481384655,193.771745245381));
#93440=CARTESIAN_POINT('Ctrl Pts',(126.579855830591,53.9516703754874,194.016863354465));
#93441=CARTESIAN_POINT('Ctrl Pts',(126.632097249348,53.9496036053775,194.702657351989));
#93442=CARTESIAN_POINT('Ctrl Pts',(127.255737937252,54.5846303501899,193.69266867861));
#93443=CARTESIAN_POINT('Ctrl Pts',(127.230565840969,53.907392591019,193.922470625941));
#93444=CARTESIAN_POINT('Ctrl Pts',(127.30024332108,53.9024781190574,194.634660522391));
#93445=CARTESIAN_POINT('Origin',(127.370600247112,54.9,194.634660522392));
#93446=CARTESIAN_POINT('Ctrl Pts',(127.272749841876,54.9000000000005,193.639459387849));
#93447=CARTESIAN_POINT('Ctrl Pts',(127.203543013627,53.909298557295,193.646263958256));
#93448=CARTESIAN_POINT('Ctrl Pts',(127.300243321063,53.9024781190585,194.634660522393));
#93449=CARTESIAN_POINT('Ctrl Pts',(128.52064511939,54.8116621740965,193.516763528339));
#93450=CARTESIAN_POINT('Ctrl Pts',(128.407405166125,53.8285119696612,193.528217006398));
#93451=CARTESIAN_POINT('Ctrl Pts',(128.510275384961,53.8171324859908,194.511516273623));
#93452=CARTESIAN_POINT('Ctrl Pts',(129.761927633803,54.643802091986,193.386070821232));
#93453=CARTESIAN_POINT('Ctrl Pts',(129.607546967154,53.6716622950793,193.402533723092));
#93454=CARTESIAN_POINT('Ctrl Pts',(129.714213057453,53.654958236656,194.380313990587));
#93455=CARTESIAN_POINT('Ctrl Pts',(131.6135224599,54.2702144010371,193.176442368403));
#93456=CARTESIAN_POINT('Ctrl Pts',(131.402782100654,53.3180517456064,193.200806873799));
#93457=CARTESIAN_POINT('Ctrl Pts',(131.510655492351,53.2940248395543,194.169798981518));
#93458=CARTESIAN_POINT('Ctrl Pts',(132.231120343818,54.1246783068022,193.104032183627));
#93459=CARTESIAN_POINT('Ctrl Pts',(132.000898867169,53.180233463908,193.13129396691));
#93460=CARTESIAN_POINT('Ctrl Pts',(132.109951292528,53.1534183951113,194.097071569746));
#93461=CARTESIAN_POINT('Ctrl Pts',(133.447960060778,53.795964138965,192.9562191062));
#93462=CARTESIAN_POINT('Ctrl Pts',(133.180061609208,52.8681545503538,192.989463215145));
#93463=CARTESIAN_POINT('Ctrl Pts',(133.290927472371,52.8358385491633,193.94858536401));
#93464=CARTESIAN_POINT('Ctrl Pts',(134.048018207581,53.6127861473261,192.880743397387));
#93465=CARTESIAN_POINT('Ctrl Pts',(133.761754639131,52.6940588112552,192.917106754388));
#93466=CARTESIAN_POINT('Ctrl Pts',(133.873399111762,52.6588652269854,193.87275353291));
#93467=CARTESIAN_POINT('Ctrl Pts',(135.823659132771,53.0080952690701,192.649586867277));
#93468=CARTESIAN_POINT('Ctrl Pts',(135.481197371613,52.11925883683,192.695966104266));
#93469=CARTESIAN_POINT('Ctrl Pts',(135.597302025426,52.0746566508346,193.640464175031));
#93470=CARTESIAN_POINT('Ctrl Pts',(136.97479908392,52.5316454904866,192.489156404314));
#93471=CARTESIAN_POINT('Ctrl Pts',(136.598560535411,51.6654276097848,192.542536330489));
#93472=CARTESIAN_POINT('Ctrl Pts',(136.715309703076,51.61434534683,193.479192548667));
#93473=CARTESIAN_POINT('Ctrl Pts',(138.6530486123,51.708035457433,192.239238024318));
#93474=CARTESIAN_POINT('Ctrl Pts',(138.233427443137,50.8764420724432,192.303042588419));
#93475=CARTESIAN_POINT('Ctrl Pts',(138.34589059586,50.818632922698,193.22785955661));
#93476=CARTESIAN_POINT('Ctrl Pts',(139.204365456023,51.415287483946,192.154391036192));
#93477=CARTESIAN_POINT('Ctrl Pts',(138.769728386523,50.596440619094,192.221944439597));
#93478=CARTESIAN_POINT('Ctrl Pts',(138.881656790172,50.5358010115302,193.142515545859));
#93479=CARTESIAN_POINT('Ctrl Pts',(140.290599308088,50.7928635888825,191.981721248658));
#93480=CARTESIAN_POINT('Ctrl Pts',(139.827189305459,50.0003680989601,192.056916645887));
#93481=CARTESIAN_POINT('Ctrl Pts',(139.937472164248,49.9344600777195,192.968796877316));
#93482=CARTESIAN_POINT('Ctrl Pts',(140.826728790772,50.4623774384289,191.89369145042));
#93483=CARTESIAN_POINT('Ctrl Pts',(140.34944784855,49.683754112497,191.972823987069));
#93484=CARTESIAN_POINT('Ctrl Pts',(140.458700441158,49.6151682704711,192.880213859559));
#93485=CARTESIAN_POINT('Ctrl Pts',(142.40172585476,49.4195194736428,191.626786341652));
#93486=CARTESIAN_POINT('Ctrl Pts',(141.881508560285,48.6857028891425,191.71841976379));
#93487=CARTESIAN_POINT('Ctrl Pts',(141.99025759904,48.6076343574705,192.611570669029));
#93488=CARTESIAN_POINT('Ctrl Pts',(143.395944403539,48.6640076534003,191.447054061697));
#93489=CARTESIAN_POINT('Ctrl Pts',(142.852474782588,47.9607749353619,191.546847984491));
#93490=CARTESIAN_POINT('Ctrl Pts',(142.957509894915,47.8777134995743,192.430587787633));
#93491=CARTESIAN_POINT('Ctrl Pts',(145.277446438577,47.0366597202735,191.087194166438));
#93492=CARTESIAN_POINT('Ctrl Pts',(144.692442366913,46.3952555402769,191.203195444119));
#93493=CARTESIAN_POINT('Ctrl Pts',(144.788791450931,46.3054876682523,192.068053266175));
#93494=CARTESIAN_POINT('Ctrl Pts',(146.164719382506,46.1648158566818,190.907052451028));
#93495=CARTESIAN_POINT('Ctrl Pts',(145.561937070811,45.5561147238115,191.031184857471));
#93496=CARTESIAN_POINT('Ctrl Pts',(145.652811102842,45.4631752067736,191.886487140678));
#93497=CARTESIAN_POINT('Ctrl Pts',(147.414929837981,44.7683638583841,190.640018592768));
#93498=CARTESIAN_POINT('Ctrl Pts',(146.791471289491,44.2057341261571,190.775475427974));
#93499=CARTESIAN_POINT('Ctrl Pts',(146.870806025728,44.1140243219997,191.617213295931));
#93500=CARTESIAN_POINT('Ctrl Pts',(147.81817715783,44.2880522144313,190.551549748198));
#93501=CARTESIAN_POINT('Ctrl Pts',(147.187487035208,43.7421608701101,190.690946555037));
#93502=CARTESIAN_POINT('Ctrl Pts',(147.263759692939,43.6499819630162,191.527980798402));
#93503=CARTESIAN_POINT('Ctrl Pts',(148.597101747504,43.2969309377458,190.376458300977));
#93504=CARTESIAN_POINT('Ctrl Pts',(147.952932529004,42.7847732161162,190.523620828458));
#93505=CARTESIAN_POINT('Ctrl Pts',(148.022976149422,42.6924322950368,191.351336094742));
#93506=CARTESIAN_POINT('Ctrl Pts',(148.97143365954,42.7876744441135,190.290130240647));
#93507=CARTESIAN_POINT('Ctrl Pts',(148.321195890274,42.2925616418689,190.441090549207));
#93508=CARTESIAN_POINT('Ctrl Pts',(148.387927948605,42.2004255165281,191.26422094652));
#93509=CARTESIAN_POINT('Ctrl Pts',(150.041310637799,41.2296646117753,190.037839922795));
#93510=CARTESIAN_POINT('Ctrl Pts',(149.371815095918,40.7891354956777,190.200429995867));
#93511=CARTESIAN_POINT('Ctrl Pts',(149.431228089319,40.6951891414559,191.009572227123));
#93512=CARTESIAN_POINT('Ctrl Pts',(150.687324774653,40.1465975881037,189.877765311828));
#93513=CARTESIAN_POINT('Ctrl Pts',(150.009650721621,39.7402487175424,190.04713963159));
#93514=CARTESIAN_POINT('Ctrl Pts',(150.061517666962,39.6488093520851,190.847921455656));
#93515=CARTESIAN_POINT('Ctrl Pts',(151.26536469753,39.0180386085743,189.729482705023));
#93516=CARTESIAN_POINT('Ctrl Pts',(150.582709291195,38.6415601415748,189.904601964429));
#93517=CARTESIAN_POINT('Ctrl Pts',(150.625700340104,38.5584761124775,190.698119455572));
#93518=CARTESIAN_POINT('Ctrl Pts',(130.970210996205,54.4,193.249273458763));
#93519=CARTESIAN_POINT('Ctrl Pts',(130.978915699594,54.3982519051478,193.248288933116));
#93520=CARTESIAN_POINT('Ctrl Pts',(130.987620092955,54.3964997672191,193.247303953753));
#93521=CARTESIAN_POINT('Ctrl Pts',(130.996324175466,54.394743585639,193.246318520373));
#93522=CARTESIAN_POINT('Ctrl Pts',(131.528258652909,54.2874176808117,193.18609551699));
#93523=CARTESIAN_POINT('Ctrl Pts',(132.060608026504,54.1644608290906,193.123976504334));
#93524=CARTESIAN_POINT('Ctrl Pts',(132.587072882371,54.0272948310328,193.060644636876));
#93525=CARTESIAN_POINT('Ctrl Pts',(132.671384407187,54.0053281711119,193.050502257465));
#93526=CARTESIAN_POINT('Ctrl Pts',(132.755547483063,53.9829974301109,193.040328484779));
#93527=CARTESIAN_POINT('Ctrl Pts',(132.839536755994,53.9603082180556,193.030126063637));
#93528=CARTESIAN_POINT('Ctrl Pts',(133.288581764007,53.8390013290499,192.97557926113));
#93529=CARTESIAN_POINT('Ctrl Pts',(133.733103527571,53.7074473366379,192.920173817067));
#93530=CARTESIAN_POINT('Ctrl Pts',(134.173150208173,53.5658027576502,192.863909643738));
#93531=CARTESIAN_POINT('Ctrl Pts',(134.329294379496,53.5155422367028,192.843945119276));
#93532=CARTESIAN_POINT('Ctrl Pts',(134.484875189166,53.4640102364994,192.823872469304));
#93533=CARTESIAN_POINT('Ctrl Pts',(134.639896091017,53.4112152443031,192.803691536399));
#93534=CARTESIAN_POINT('Ctrl Pts',(135.52206560457,53.1107774837966,192.688848934204));
#93535=CARTESIAN_POINT('Ctrl Pts',(136.386150108309,52.7695638810176,192.570489258043));
#93536=CARTESIAN_POINT('Ctrl Pts',(137.232334271804,52.3879729388403,192.448662213503));
#93537=CARTESIAN_POINT('Ctrl Pts',(137.521497146559,52.2575735073922,192.407030781551));
#93538=CARTESIAN_POINT('Ctrl Pts',(137.808605915557,52.1224240283374,192.364989126719));
#93539=CARTESIAN_POINT('Ctrl Pts',(138.093623908729,51.9825549712515,192.322545371402));
#93540=CARTESIAN_POINT('Ctrl Pts',(138.582860279063,51.742468269885,192.249690220878));
#93541=CARTESIAN_POINT('Ctrl Pts',(139.065917548896,51.4884308348136,192.175653643355));
#93542=CARTESIAN_POINT('Ctrl Pts',(139.54253534821,51.2204058123117,192.100502844523));
#93543=CARTESIAN_POINT('Ctrl Pts',(139.610982501645,51.1819146987483,192.089710427064));
#93544=CARTESIAN_POINT('Ctrl Pts',(139.67929688751,51.1431351852349,192.078895035667));
#93545=CARTESIAN_POINT('Ctrl Pts',(139.74747777422,51.1040672416763,192.068056874941));
#93546=CARTESIAN_POINT('Ctrl Pts',(139.879558530241,51.0283843960807,192.047061071988));
#93547=CARTESIAN_POINT('Ctrl Pts',(140.011209984247,50.9515712029546,192.025967578531));
#93548=CARTESIAN_POINT('Ctrl Pts',(140.142368765457,50.8736620979774,192.004788014758));
#93549=CARTESIAN_POINT('Ctrl Pts',(140.433548249307,50.7006997330856,191.957768254505));
#93550=CARTESIAN_POINT('Ctrl Pts',(140.722715780357,50.5220779847515,191.910256482707));
#93551=CARTESIAN_POINT('Ctrl Pts',(141.008893216184,50.3383113755541,191.862422646825));
#93552=CARTESIAN_POINT('Ctrl Pts',(141.123671784854,50.2646072125688,191.843237698855));
#93553=CARTESIAN_POINT('Ctrl Pts',(141.237969574942,50.1900759905089,191.824000990223));
#93554=CARTESIAN_POINT('Ctrl Pts',(141.351724540188,50.1147530003429,191.804723635321));
#93555=CARTESIAN_POINT('Ctrl Pts',(141.414571048868,50.073139107313,191.794073423705));
#93556=CARTESIAN_POINT('Ctrl Pts',(141.477211554499,50.031313156935,191.783417824362));
#93557=CARTESIAN_POINT('Ctrl Pts',(141.539643328611,49.9892780028454,191.772757758386));
#93558=CARTESIAN_POINT('Ctrl Pts',(141.996832974707,49.6814533815665,191.694693794001));
#93559=CARTESIAN_POINT('Ctrl Pts',(142.443279186456,49.3620733715139,191.61631369272));
#93560=CARTESIAN_POINT('Ctrl Pts',(142.879234659791,49.031386758862,191.537742560243));
#93561=CARTESIAN_POINT('Ctrl Pts',(143.378755062999,48.6524840493176,191.447715284119));
#93562=CARTESIAN_POINT('Ctrl Pts',(143.864466586805,48.2586932138852,191.357443433954));
#93563=CARTESIAN_POINT('Ctrl Pts',(144.336661238865,47.8502924156543,191.267130653307));
#93564=CARTESIAN_POINT('Ctrl Pts',(145.277629212541,47.0364499253106,191.087159461698));
#93565=CARTESIAN_POINT('Ctrl Pts',(146.164908890879,46.1645799402394,190.907011931677));
#93566=CARTESIAN_POINT('Ctrl Pts',(146.998187380399,45.2338425346647,190.729031083346));
#93567=CARTESIAN_POINT('Ctrl Pts',(147.2065276244,45.0011351497774,190.684531466669));
#93568=CARTESIAN_POINT('Ctrl Pts',(147.411482299837,44.764736358989,190.640170437272));
#93569=CARTESIAN_POINT('Ctrl Pts',(147.613014815304,44.5245956946798,190.59599572238));
#93570=CARTESIAN_POINT('Ctrl Pts',(147.814604235587,44.28438722414,190.551808534294));
#93571=CARTESIAN_POINT('Ctrl Pts',(148.012855510647,44.0403342210074,190.507788751385));
#93572=CARTESIAN_POINT('Ctrl Pts',(148.207638105612,43.792490454076,190.464004327389));
#93573=CARTESIAN_POINT('Ctrl Pts',(148.353953896311,43.6063164443546,190.431114568329));
#93574=CARTESIAN_POINT('Ctrl Pts',(148.498122737652,43.4182230180028,190.398399194814));
#93575=CARTESIAN_POINT('Ctrl Pts',(148.639973419214,43.2284516503636,190.365920168262));
#93576=CARTESIAN_POINT('Ctrl Pts',(148.861528696448,42.9320494934958,190.315191474874));
#93577=CARTESIAN_POINT('Ctrl Pts',(149.077359267845,42.6316595878099,190.265055846598));
#93578=CARTESIAN_POINT('Ctrl Pts',(149.287156197482,42.3277350997865,190.215670418501));
#93579=CARTESIAN_POINT('Ctrl Pts',(149.300814102149,42.3079494351891,190.212455397813));
#93580=CARTESIAN_POINT('Ctrl Pts',(149.314446420857,42.2881487801072,190.209243558129));
#93581=CARTESIAN_POINT('Ctrl Pts',(149.32805306199,42.268333255379,190.206034943533));
#93582=CARTESIAN_POINT('Ctrl Pts',(149.417400435735,42.1382155373879,190.184965725587));
#93583=CARTESIAN_POINT('Ctrl Pts',(149.505697057769,42.0073928187187,190.164022900144));
#93584=CARTESIAN_POINT('Ctrl Pts',(149.59295522357,41.8758397422702,190.143210337197));
#93585=CARTESIAN_POINT('Ctrl Pts',(150.13058284509,41.0652959158561,190.014976966573));
#93586=CARTESIAN_POINT('Ctrl Pts',(150.62797127562,40.2285141913915,189.891883007592));
#93587=CARTESIAN_POINT('Ctrl Pts',(151.084752919722,39.3649994489525,189.775631285513));
#93588=CARTESIAN_POINT('Ctrl Pts',(151.145679577168,39.2498217320022,189.760125345333));
#93589=CARTESIAN_POINT('Ctrl Pts',(151.205883795788,39.1341684866594,189.744741137557));
#93590=CARTESIAN_POINT('Ctrl Pts',(151.265364697529,39.0180386085774,189.729482705023));
#93591=CARTESIAN_POINT('Origin',(125.29348064571,25.4505574462982,200.));
#93592=CARTESIAN_POINT('Ctrl Pts',(1.55981000190379E-14,25.8701893108725,
195.999534166346));
#93593=CARTESIAN_POINT('Ctrl Pts',(1.55970277531197E-14,24.8757620423259,
195.993992404177));
#93594=CARTESIAN_POINT('Ctrl Pts',(1.54046147636829E-14,24.8757620423259,
194.999549694134));
#93595=CARTESIAN_POINT('Ctrl Pts',(-8.21740721796392,25.8701893108446,195.999534166345));
#93596=CARTESIAN_POINT('Ctrl Pts',(-8.21741052170387,24.8757620423259,195.993992404063));
#93597=CARTESIAN_POINT('Ctrl Pts',(-8.21804707909509,24.8757620423259,194.999549694362));
#93598=CARTESIAN_POINT('Ctrl Pts',(-16.4351123294179,25.8705045195437,196.008014433201));
#93599=CARTESIAN_POINT('Ctrl Pts',(-16.4284754963483,24.8757620422117,196.002778286315));
#93600=CARTESIAN_POINT('Ctrl Pts',(-16.4360935882987,24.8757620423259,195.008027382868));
#93601=CARTESIAN_POINT('Ctrl Pts',(-32.8716902536231,25.8672519270132,196.020072042458));
#93602=CARTESIAN_POINT('Ctrl Pts',(-32.8650631301397,24.8757620424398,196.011627858086));
#93603=CARTESIAN_POINT('Ctrl Pts',(-32.8721788518652,24.8757620423259,195.02010702045));
#93604=CARTESIAN_POINT('Ctrl Pts',(-41.0905284509966,25.8637497700185,196.024420502657));
#93605=CARTESIAN_POINT('Ctrl Pts',(-41.061781966308,24.8757620424403,196.012595535246));
#93606=CARTESIAN_POINT('Ctrl Pts',(-41.0902164350087,24.8757620423259,195.024465281298));
#93607=CARTESIAN_POINT('Ctrl Pts',(-57.530618958565,25.8495382670329,195.984820115083));
#93608=CARTESIAN_POINT('Ctrl Pts',(-57.5019615256235,24.8757620422122,195.959319017969));
#93609=CARTESIAN_POINT('Ctrl Pts',(-57.5261473827835,24.8757620423259,194.985146590421));
#93610=CARTESIAN_POINT('Ctrl Pts',(-65.752229349423,25.8388537616774,195.942570987272));
#93611=CARTESIAN_POINT('Ctrl Pts',(-65.6887149097543,24.8757620425557,195.907765994157));
#93612=CARTESIAN_POINT('Ctrl Pts',(-65.7444507976842,24.8757620423259,194.943132932891));
#93613=CARTESIAN_POINT('Ctrl Pts',(-78.0874808464977,25.8147115657548,195.767826780906));
#93614=CARTESIAN_POINT('Ctrl Pts',(-78.0708636749413,24.8757620422123,195.710593550958));
#93615=CARTESIAN_POINT('Ctrl Pts',(-78.0703083245555,24.8757620423259,194.769802366593));
#93616=CARTESIAN_POINT('Ctrl Pts',(-82.1988777916636,25.8053087434596,195.69044692859));
#93617=CARTESIAN_POINT('Ctrl Pts',(-82.1765025713025,24.875762042376,195.625301040975));
#93618=CARTESIAN_POINT('Ctrl Pts',(-82.1778160289154,24.8757620423259,194.693080125928));
#93619=CARTESIAN_POINT('Ctrl Pts',(-90.4203625136221,25.7832828451603,195.47321942372));
#93620=CARTESIAN_POINT('Ctrl Pts',(-90.3969486708277,24.8757620422763,195.389459554287));
#93621=CARTESIAN_POINT('Ctrl Pts',(-90.3892106396611,24.8757620423259,194.477917980567));
#93622=CARTESIAN_POINT('Ctrl Pts',(-94.5304565710492,25.770658639565,195.33357508742));
#93623=CARTESIAN_POINT('Ctrl Pts',(-94.5002180268611,24.8757620423259,195.240180499821));
#93624=CARTESIAN_POINT('Ctrl Pts',(-94.4931091307174,24.8757620423259,194.339675539885));
#93625=CARTESIAN_POINT('Ctrl Pts',(-102.748391728739,25.7416579173973,194.954772731233));
#93626=CARTESIAN_POINT('Ctrl Pts',(-102.715751986094,24.8757620423259,194.838866884368));
#93627=CARTESIAN_POINT('Ctrl Pts',(-102.695151200076,24.8757620423259,193.96509632142));
#93628=CARTESIAN_POINT('Ctrl Pts',(-106.856246027343,25.725278146861,194.715964350451));
#93629=CARTESIAN_POINT('Ctrl Pts',(-106.81543638418,24.875762042369,194.589246043723));
#93630=CARTESIAN_POINT('Ctrl Pts',(-106.793314622248,24.8757620423259,193.729097788723));
#93631=CARTESIAN_POINT('Ctrl Pts',(-115.068137297811,25.6882726032458,194.080718037657));
#93632=CARTESIAN_POINT('Ctrl Pts',(-115.022239145157,24.8757620422835,193.928538627727));
#93633=CARTESIAN_POINT('Ctrl Pts',(-114.980548200328,24.8757620423259,193.102103079899));
#93634=CARTESIAN_POINT('Ctrl Pts',(-119.172205639421,25.6676398016414,193.684925703402));
#93635=CARTESIAN_POINT('Ctrl Pts',(-119.116329484592,24.8757620423259,193.521895669482));
#93636=CARTESIAN_POINT('Ctrl Pts',(-119.069654868258,24.8757620423259,192.711729260958));
#93637=CARTESIAN_POINT('Ctrl Pts',(-125.323347744084,25.6332752863461,192.902977900697));
#93638=CARTESIAN_POINT('Ctrl Pts',(-125.288387595195,24.8757620423259,192.716487359207));
#93639=CARTESIAN_POINT('Ctrl Pts',(-125.192484832993,24.8757620423259,191.941567071429));
#93640=CARTESIAN_POINT('Ctrl Pts',(-127.374905650878,25.6212405876043,192.61026813322));
#93641=CARTESIAN_POINT('Ctrl Pts',(-127.336151672754,24.8757620423474,192.417706213037));
#93642=CARTESIAN_POINT('Ctrl Pts',(-127.233608145136,24.8757620423259,191.653411387743));
#93643=CARTESIAN_POINT('Ctrl Pts',(-131.463610310007,25.5961158342195,191.946252068015));
#93644=CARTESIAN_POINT('Ctrl Pts',(-131.417681393358,24.8757620423046,191.741054985749));
#93645=CARTESIAN_POINT('Ctrl Pts',(-131.299148124053,24.8757620423259,191.000170054907));
#93646=CARTESIAN_POINT('Ctrl Pts',(-133.500663498608,25.5830272913609,191.575072827975));
#93647=CARTESIAN_POINT('Ctrl Pts',(-133.450072443569,24.8757620423438,191.364331943371));
#93648=CARTESIAN_POINT('Ctrl Pts',(-133.323473052073,24.8757620423259,190.635208210175));
#93649=CARTESIAN_POINT('Ctrl Pts',(-137.556266128696,25.5558831018172,190.734424603672));
#93650=CARTESIAN_POINT('Ctrl Pts',(-137.49615141237,24.8757620423081,190.51226943187));
#93651=CARTESIAN_POINT('Ctrl Pts',(-137.350968148536,24.8757620423259,189.809240410191));
#93652=CARTESIAN_POINT('Ctrl Pts',(-139.574830376325,25.5418271597114,190.265017746423));
#93653=CARTESIAN_POINT('Ctrl Pts',(-139.50891157162,24.8757620423438,190.038258843073));
#93654=CARTESIAN_POINT('Ctrl Pts',(-139.354151496503,24.8757620423259,189.348294290982));
#93655=CARTESIAN_POINT('Ctrl Pts',(-142.584968697329,25.5201265620969,189.468074534053));
#93656=CARTESIAN_POINT('Ctrl Pts',(-142.517789134679,24.875762042317,189.232187304688));
#93657=CARTESIAN_POINT('Ctrl Pts',(-142.338980713026,24.8757620423259,188.56631973987));
#93658=CARTESIAN_POINT('Ctrl Pts',(-143.585385950339,25.5127907503976,189.186905273307));
#93659=CARTESIAN_POINT('Ctrl Pts',(-143.514862987652,24.8757620423259,188.948964700898));
#93660=CARTESIAN_POINT('Ctrl Pts',(-143.330589015116,24.8757620423259,188.290521463128));
#93661=CARTESIAN_POINT('Ctrl Pts',(-145.579494487103,25.4979389111357,188.589605422417));
#93662=CARTESIAN_POINT('Ctrl Pts',(-145.501925955778,24.8757620423259,188.347761030563));
#93663=CARTESIAN_POINT('Ctrl Pts',(-145.306300715501,24.8757620423259,187.704852113735));
#93664=CARTESIAN_POINT('Ctrl Pts',(-146.574200692161,25.49041488071,188.273089407368));
#93665=CARTESIAN_POINT('Ctrl Pts',(-146.492901158935,24.8757620423259,188.029599291115));
#93666=CARTESIAN_POINT('Ctrl Pts',(-146.291407749267,24.8757620423259,187.394603605153));
#93667=CARTESIAN_POINT('Ctrl Pts',(-149.530965389848,25.4677381713212,187.269955276074));
#93668=CARTESIAN_POINT('Ctrl Pts',(-149.429901591881,24.8757620423259,187.024697733763));
#93669=CARTESIAN_POINT('Ctrl Pts',(-149.218333471988,24.8757620423259,186.411710463469));
#93670=CARTESIAN_POINT('Ctrl Pts',(-151.469919324602,25.4524496338339,186.528895379912));
#93671=CARTESIAN_POINT('Ctrl Pts',(-151.360643558434,24.8757620423259,186.282461960026));
#93672=CARTESIAN_POINT('Ctrl Pts',(-151.135962079037,24.8757620423259,185.686074351676));
#93673=CARTESIAN_POINT('Ctrl Pts',(-155.268552533548,25.421878992293,184.870449086661));
#93674=CARTESIAN_POINT('Ctrl Pts',(-155.140301022575,24.8757620423259,184.622711642346));
#93675=CARTESIAN_POINT('Ctrl Pts',(-154.889283187975,24.8757620423259,184.063471352248));
#93676=CARTESIAN_POINT('Ctrl Pts',(-157.128318393194,25.4065973813273,183.953242115242));
#93677=CARTESIAN_POINT('Ctrl Pts',(-156.990494177067,24.8757620423259,183.707070687992));
#93678=CARTESIAN_POINT('Ctrl Pts',(-156.725059327294,24.8757620423259,183.166679353191));
#93679=CARTESIAN_POINT('Ctrl Pts',(-159.843877846741,25.3839693077877,182.4143228812));
#93680=CARTESIAN_POINT('Ctrl Pts',(-159.696302120373,24.8757620423259,182.167954674856));
#93681=CARTESIAN_POINT('Ctrl Pts',(-159.403034456653,24.8757620423259,181.663223290672));
#93682=CARTESIAN_POINT('Ctrl Pts',(-160.736671906421,25.3764758830308,181.874075657354));
#93683=CARTESIAN_POINT('Ctrl Pts',(-160.58348509393,24.8757620423331,181.629500993224));
#93684=CARTESIAN_POINT('Ctrl Pts',(-160.283036640086,24.8757620423259,181.135606802703));
#93685=CARTESIAN_POINT('Ctrl Pts',(-162.054867926021,25.3653482837207,181.017753243736));
#93686=CARTESIAN_POINT('Ctrl Pts',(-161.894451982614,24.8757620423223,180.775409581153));
#93687=CARTESIAN_POINT('Ctrl Pts',(-161.581727876928,24.8757620423259,180.299617979711));
#93688=CARTESIAN_POINT('Ctrl Pts',(-162.490762640011,25.361657861326,180.724643998008));
#93689=CARTESIAN_POINT('Ctrl Pts',(-162.32737504632,24.8757620423286,180.483534423218));
#93690=CARTESIAN_POINT('Ctrl Pts',(-162.011068383027,24.8757620423259,180.01351814156));
#93691=CARTESIAN_POINT('Ctrl Pts',(-163.355074229889,25.354321385116,180.122105972292));
#93692=CARTESIAN_POINT('Ctrl Pts',(-163.185636865372,24.8757620423232,179.883705522239));
#93693=CARTESIAN_POINT('Ctrl Pts',(-162.862182136119,24.8757620423259,179.42549510677));
#93694=CARTESIAN_POINT('Ctrl Pts',(-163.784024035092,25.3506707582467,179.812243966753));
#93695=CARTESIAN_POINT('Ctrl Pts',(-163.611544779999,24.8757620423259,179.575344130263));
#93696=CARTESIAN_POINT('Ctrl Pts',(-163.284479634629,24.8757620423259,179.123149423031));
#93697=CARTESIAN_POINT('Ctrl Pts',(-165.893924132154,25.3326733753055,178.230844182634));
#93698=CARTESIAN_POINT('Ctrl Pts',(-165.698702838315,24.8757620423259,178.007586069906));
#93699=CARTESIAN_POINT('Ctrl Pts',(-165.361175322346,24.8757620423259,177.580381667324));
#93700=CARTESIAN_POINT('Ctrl Pts',(-167.481106685865,25.3190005603972,176.856948482142));
#93701=CARTESIAN_POINT('Ctrl Pts',(-167.275278221452,24.8757620423152,176.642444583454));
#93702=CARTESIAN_POINT('Ctrl Pts',(-166.921818221905,24.8757620423259,176.240893842191));
#93703=CARTESIAN_POINT('Ctrl Pts',(-169.684665227087,25.2999653906393,174.605906246088));
#93704=CARTESIAN_POINT('Ctrl Pts',(-169.464760847503,24.8757620423312,174.403386973429));
#93705=CARTESIAN_POINT('Ctrl Pts',(-169.086795032884,24.8757620423259,174.047706451662));
#93706=CARTESIAN_POINT('Ctrl Pts',(-170.389548700331,25.2938670470603,173.823752953021));
#93707=CARTESIAN_POINT('Ctrl Pts',(-170.163773376106,24.8757620423223,173.627328010298));
#93708=CARTESIAN_POINT('Ctrl Pts',(-169.779023946969,24.8757620423259,173.285881474387));
#93709=CARTESIAN_POINT('Ctrl Pts',(-171.733708831765,25.2822654981617,172.189187311864));
#93710=CARTESIAN_POINT('Ctrl Pts',(-171.495932116079,24.8757620423295,172.006291779375));
#93711=CARTESIAN_POINT('Ctrl Pts',(-171.098494081107,24.8757620423259,171.694301405067));
#93712=CARTESIAN_POINT('Ctrl Pts',(-172.374791488579,25.2767480891279,171.333293369278));
#93713=CARTESIAN_POINT('Ctrl Pts',(-172.131402736303,24.8757620423313,171.157743137787));
#93714=CARTESIAN_POINT('Ctrl Pts',(-171.727502211852,24.8757620423259,170.861160982562));
#93715=CARTESIAN_POINT('Ctrl Pts',(-174.149962214451,25.2616143901389,168.706265498992));
#93716=CARTESIAN_POINT('Ctrl Pts',(-173.887056783482,24.8757620423152,168.558753202255));
#93717=CARTESIAN_POINT('Ctrl Pts',(-173.46844284384,24.8757620423259,168.304775190926));
#93718=CARTESIAN_POINT('Ctrl Pts',(-175.149896364286,25.2536804395812,166.860854093189));
#93719=CARTESIAN_POINT('Ctrl Pts',(-174.87876760015,24.8757620423401,166.730672448768));
#93720=CARTESIAN_POINT('Ctrl Pts',(-174.447418189425,24.8757620423259,166.510636295168));
#93721=CARTESIAN_POINT('Ctrl Pts',(-176.347229631101,25.2428388848927,163.944275786663));
#93722=CARTESIAN_POINT('Ctrl Pts',(-176.065432586062,24.8757620423188,163.840418898352));
#93723=CARTESIAN_POINT('Ctrl Pts',(-175.621308989244,24.8757620423259,163.673672937929));
#93724=CARTESIAN_POINT('Ctrl Pts',(-176.69550116753,25.239240468917,162.947498775422));
#93725=CARTESIAN_POINT('Ctrl Pts',(-176.410357889342,24.8757620423187,162.853899660982));
#93726=CARTESIAN_POINT('Ctrl Pts',(-175.96335024238,24.8757620423259,162.703646661311));
#93727=CARTESIAN_POINT('Ctrl Pts',(-177.143858779535,25.2329712637093,161.419747762863));
#93728=CARTESIAN_POINT('Ctrl Pts',(-176.85502728246,24.8757620423295,161.339448567081));
#93729=CARTESIAN_POINT('Ctrl Pts',(-176.405926433472,24.8757620423259,161.213730765013));
#93730=CARTESIAN_POINT('Ctrl Pts',(-177.281257913445,25.2307372146378,160.904114441399));
#93731=CARTESIAN_POINT('Ctrl Pts',(-176.991292739235,24.8757620423295,160.828489480191));
#93732=CARTESIAN_POINT('Ctrl Pts',(-176.54197824777,24.8757620423259,160.710339939802));
#93733=CARTESIAN_POINT('Ctrl Pts',(-177.530501036989,25.2260187908126,159.875002150419));
#93734=CARTESIAN_POINT('Ctrl Pts',(-177.238632774441,24.8757620423223,159.808152124321));
#93735=CARTESIAN_POINT('Ctrl Pts',(-176.789652532962,24.8757620423259,159.704364492039));
#93736=CARTESIAN_POINT('Ctrl Pts',(-177.642808421522,25.2235311200789,159.360184292277));
#93737=CARTESIAN_POINT('Ctrl Pts',(-177.350180560588,24.8757620423268,159.297529645419));
#93738=CARTESIAN_POINT('Ctrl Pts',(-176.901727564712,24.8757620423259,159.200477903653));
#93739=CARTESIAN_POINT('Ctrl Pts',(-178.150698495911,25.2105673597152,156.785499624353));
#93740=CARTESIAN_POINT('Ctrl Pts',(-177.853818377308,24.8757620423223,156.748431812088));
#93741=CARTESIAN_POINT('Ctrl Pts',(-177.410722924974,24.8757620423259,156.677118500037));
#93742=CARTESIAN_POINT('Ctrl Pts',(-178.38892700326,25.1986131825788,154.724292736304));
#93743=CARTESIAN_POINT('Ctrl Pts',(-178.092734343343,24.8757620423793,154.699739042078));
#93744=CARTESIAN_POINT('Ctrl Pts',(-177.656737843813,24.8757620423259,154.646113775664));
#93745=CARTESIAN_POINT('Ctrl Pts',(-178.535788240059,25.1869009068823,152.663678496546));
#93746=CARTESIAN_POINT('Ctrl Pts',(-178.240980734254,24.8757620423259,152.641070351893));
#93747=CARTESIAN_POINT('Ctrl Pts',(-177.813017113378,24.8757620423259,152.608250755187));
#93748=CARTESIAN_POINT('',(1.54046147636829E-14,24.8757620423259,194.999549694134));
#93749=CARTESIAN_POINT('',(1.58047048864619E-14,25.8701893108725,195.999534166346));
#93750=CARTESIAN_POINT('Origin',(1.54046147636829E-14,25.8757620423259,
194.999549694134));
#93751=CARTESIAN_POINT('',(-178.53578824005,25.1869009068724,152.663678496545));
#93752=CARTESIAN_POINT('Ctrl Pts',(-178.535788240059,25.1869009068823,152.663678496546));
#93753=CARTESIAN_POINT('Ctrl Pts',(-178.497300169629,25.1899703544864,153.203705718586));
#93754=CARTESIAN_POINT('Ctrl Pts',(-178.452605703909,25.1930505432942,153.74275174592));
#93755=CARTESIAN_POINT('Ctrl Pts',(-178.400429730265,25.1961079530536,154.280627961182));
#93756=CARTESIAN_POINT('Ctrl Pts',(-178.349499261461,25.1990923786713,154.805664407814));
#93757=CARTESIAN_POINT('Ctrl Pts',(-178.291439967185,25.202055092476,155.329586217056));
#93758=CARTESIAN_POINT('Ctrl Pts',(-178.225113983825,25.204965729571,155.85221882764));
#93759=CARTESIAN_POINT('Ctrl Pts',(-178.160952607745,25.2077813754435,156.357794859552));
#93760=CARTESIAN_POINT('Ctrl Pts',(-178.0890552258,25.2105482841908,156.862164463122));
#93761=CARTESIAN_POINT('Ctrl Pts',(-178.008439607117,25.2132398164984,157.365170531856));
#93762=CARTESIAN_POINT('Ctrl Pts',(-177.929150781168,25.21588705087,157.859897996418));
#93763=CARTESIAN_POINT('Ctrl Pts',(-177.841428154854,25.2184613643469,158.353306433683));
#93764=CARTESIAN_POINT('Ctrl Pts',(-177.744386392921,25.2209383168131,158.845247349922));
#93765=CARTESIAN_POINT('Ctrl Pts',(-177.743350247437,25.2209647640154,158.850499958162));
#93766=CARTESIAN_POINT('Ctrl Pts',(-177.742313016692,25.220991199489,158.855752396207));
#93767=CARTESIAN_POINT('Ctrl Pts',(-177.741274699235,25.2210176232105,158.861004663759));
#93768=CARTESIAN_POINT('Ctrl Pts',(-177.646352097481,25.2234332701475,159.341165039959));
#93769=CARTESIAN_POINT('Ctrl Pts',(-177.542342526488,25.2257507195669,159.819902563843));
#93770=CARTESIAN_POINT('Ctrl Pts',(-177.428152198495,25.2279524716699,160.297046148221));
#93771=CARTESIAN_POINT('Ctrl Pts',(-177.420819639305,25.2280938538508,160.327685201773));
#93772=CARTESIAN_POINT('Ctrl Pts',(-177.413445118906,25.228234759215,160.358317684296));
#93773=CARTESIAN_POINT('Ctrl Pts',(-177.406028355073,25.228375183231,160.388943551061));
#93774=CARTESIAN_POINT('Ctrl Pts',(-177.405978730098,25.2283761227969,160.38914846629));
#93775=CARTESIAN_POINT('Ctrl Pts',(-177.405929103243,25.228377062341,160.389353381181));
#93776=CARTESIAN_POINT('Ctrl Pts',(-177.405879474506,25.2283780018634,160.389558295734));
#93777=CARTESIAN_POINT('Ctrl Pts',(-177.327469296974,25.2298623861984,160.713309967531));
#93778=CARTESIAN_POINT('Ctrl Pts',(-177.244183872507,25.2312938639448,161.03674586819));
#93779=CARTESIAN_POINT('Ctrl Pts',(-177.156159366085,25.232669467775,161.358388065109));
#93780=CARTESIAN_POINT('Ctrl Pts',(-177.106238966282,25.2334495993085,161.540797574875));
#93781=CARTESIAN_POINT('Ctrl Pts',(-177.054793463084,25.2342117537668,161.722630946496));
#93782=CARTESIAN_POINT('Ctrl Pts',(-177.001840977559,25.2349553293434,161.903621195652));
#93783=CARTESIAN_POINT('Ctrl Pts',(-176.999365614225,25.2349900891795,161.912081924589));
#93784=CARTESIAN_POINT('Ctrl Pts',(-176.996886965513,25.2350248092209,161.920540784291));
#93785=CARTESIAN_POINT('Ctrl Pts',(-176.994405034784,25.2350594893758,161.928997741723));
#93786=CARTESIAN_POINT('Ctrl Pts',(-176.837547755075,25.2372512647935,162.463474921929));
#93787=CARTESIAN_POINT('Ctrl Pts',(-176.667267889636,25.2392828103483,162.991404312881));
#93788=CARTESIAN_POINT('Ctrl Pts',(-176.483342251063,25.2412384685856,163.512642511656));
#93789=CARTESIAN_POINT('Ctrl Pts',(-176.325980687731,25.242911674344,163.958599140999));
#93790=CARTESIAN_POINT('Ctrl Pts',(-176.158629659706,25.2445292808119,164.399657606776));
#93791=CARTESIAN_POINT('Ctrl Pts',(-175.981121483524,25.2461434645031,164.835716213452));
#93792=CARTESIAN_POINT('Ctrl Pts',(-175.970156859221,25.2462431721229,164.862651416659));
#93793=CARTESIAN_POINT('Ctrl Pts',(-175.959153364956,25.2463428834581,164.889567836151));
#93794=CARTESIAN_POINT('Ctrl Pts',(-175.94811096596,25.2464426111523,164.916465420591));
#93795=CARTESIAN_POINT('Ctrl Pts',(-175.659320785773,25.2490507743609,165.61991385235));
#93796=CARTESIAN_POINT('Ctrl Pts',(-175.344140309045,25.2517544614552,166.310398234908));
#93797=CARTESIAN_POINT('Ctrl Pts',(-175.003342450806,25.2546225778795,166.988304176856));
#93798=CARTESIAN_POINT('Ctrl Pts',(-174.654435203123,25.2575589420128,167.682341098376));
#93799=CARTESIAN_POINT('Ctrl Pts',(-174.278676824774,25.2606676279253,168.363193861084));
#93800=CARTESIAN_POINT('Ctrl Pts',(-173.87684769516,25.2640230810151,169.03125108838));
#93801=CARTESIAN_POINT('Ctrl Pts',(-173.623321907699,25.2661401348179,169.452747993748));
#93802=CARTESIAN_POINT('Ctrl Pts',(-173.359417112121,25.2683554311092,169.869150852764));
#93803=CARTESIAN_POINT('Ctrl Pts',(-173.085319953511,25.2706878379522,170.280552263732));
#93804=CARTESIAN_POINT('Ctrl Pts',(-173.04591944413,25.271023113291,170.339689779912));
#93805=CARTESIAN_POINT('Ctrl Pts',(-173.006317841426,25.271360622038,170.398709526143));
#93806=CARTESIAN_POINT('Ctrl Pts',(-172.966513141016,25.2717004535672,170.457616103021));
#93807=CARTESIAN_POINT('Ctrl Pts',(-172.789438023641,25.2732122274859,170.719667793079));
#93808=CARTESIAN_POINT('Ctrl Pts',(-172.608035715689,25.2747640234387,170.979815978787));
#93809=CARTESIAN_POINT('Ctrl Pts',(-172.422531449036,25.2763541171347,171.23792999103));
#93810=CARTESIAN_POINT('Ctrl Pts',(-172.345699804947,25.2770126977437,171.34483493872));
#93811=CARTESIAN_POINT('Ctrl Pts',(-172.268163938986,25.2776778538747,171.451390649919));
#93812=CARTESIAN_POINT('Ctrl Pts',(-172.18993771799,25.2783494853052,171.557586363661));
#93813=CARTESIAN_POINT('Ctrl Pts',(-171.979411745319,25.2801570104337,171.84338511048));
#93814=CARTESIAN_POINT('Ctrl Pts',(-171.764071045959,25.2820098626848,172.126315848985));
#93815=CARTESIAN_POINT('Ctrl Pts',(-171.544848096176,25.2838950226329,172.405334618166));
#93816=CARTESIAN_POINT('Ctrl Pts',(-171.441729184068,25.2847817712293,172.536580511737));
#93817=CARTESIAN_POINT('Ctrl Pts',(-171.337751912468,25.2856756597066,172.666961263959));
#93818=CARTESIAN_POINT('Ctrl Pts',(-171.233016183297,25.2865752923589,172.796371004303));
#93819=CARTESIAN_POINT('Ctrl Pts',(-171.17612444317,25.2870639667345,172.866665500515));
#93820=CARTESIAN_POINT('Ctrl Pts',(-171.118988187389,25.2875552733446,172.936700069534));
#93821=CARTESIAN_POINT('Ctrl Pts',(-171.061619131872,25.2880490444023,173.006462145406));
#93822=CARTESIAN_POINT('Ctrl Pts',(-170.680368993122,25.2913304350851,173.470070982369));
#93823=CARTESIAN_POINT('Ctrl Pts',(-170.288253320335,25.2947253627475,173.922762685443));
#93824=CARTESIAN_POINT('Ctrl Pts',(-169.885958968133,25.2982089938393,174.364917953415));
#93825=CARTESIAN_POINT('Ctrl Pts',(-169.652057198546,25.3002344447871,174.621995635577));
#93826=CARTESIAN_POINT('Ctrl Pts',(-169.414715275907,25.3022898525701,174.875512212633));
#93827=CARTESIAN_POINT('Ctrl Pts',(-169.174073915602,25.3043700857121,175.125548134129));
#93828=CARTESIAN_POINT('Ctrl Pts',(-169.099746717454,25.3050126099263,175.202777042149));
#93829=CARTESIAN_POINT('Ctrl Pts',(-169.02510205045,25.3056576781881,175.279676910402));
#93830=CARTESIAN_POINT('Ctrl Pts',(-168.950143152317,25.3063052525107,175.356251130019));
#93831=CARTESIAN_POINT('Ctrl Pts',(-168.078449890391,25.3138358617872,176.246728884361));
#93832=CARTESIAN_POINT('Ctrl Pts',(-167.164400855462,25.3217035673909,177.09331430014));
#93833=CARTESIAN_POINT('Ctrl Pts',(-166.211448824813,25.3298819796683,177.8995754802));
#93834=CARTESIAN_POINT('Ctrl Pts',(-165.665772060563,25.3345650795566,178.361254534051));
#93835=CARTESIAN_POINT('Ctrl Pts',(-165.107339947121,25.3393501326907,178.809712437871));
#93836=CARTESIAN_POINT('Ctrl Pts',(-164.536805415267,25.344232845357,179.245625184694));
#93837=CARTESIAN_POINT('Ctrl Pts',(-164.426984425153,25.345172708432,179.329533111009));
#93838=CARTESIAN_POINT('Ctrl Pts',(-164.31671449233,25.3461155817281,179.412976159758));
#93839=CARTESIAN_POINT('Ctrl Pts',(-164.206000395446,25.3470614307091,179.495959084527));
#93840=CARTESIAN_POINT('Ctrl Pts',(-163.784175350291,25.3506651523702,179.812127277856));
#93841=CARTESIAN_POINT('Ctrl Pts',(-163.35522805828,25.3543178969937,180.121997119112));
#93842=CARTESIAN_POINT('Ctrl Pts',(-162.922917985055,25.3579883154489,180.423374333965));
#93843=CARTESIAN_POINT('Ctrl Pts',(-162.614980433254,25.360602780721,180.638047475903));
#93844=CARTESIAN_POINT('Ctrl Pts',(-162.305066748929,25.3632285329527,180.848631163179));
#93845=CARTESIAN_POINT('Ctrl Pts',(-161.993261623921,25.3658651734537,181.05529624663));
#93846=CARTESIAN_POINT('Ctrl Pts',(-161.867636169548,25.3669274688888,181.1385610583));
#93847=CARTESIAN_POINT('Ctrl Pts',(-161.74170349846,25.3679913696006,181.221189795947));
#93848=CARTESIAN_POINT('Ctrl Pts',(-161.615469046877,25.3690568361265,181.303193728346));
#93849=CARTESIAN_POINT('Ctrl Pts',(-160.873076979922,25.3753229060188,181.785463569176));
#93850=CARTESIAN_POINT('Ctrl Pts',(-160.120260430856,25.3816429921167,182.246150230608));
#93851=CARTESIAN_POINT('Ctrl Pts',(-159.357962893647,25.3880105482161,182.68721140722));
#93852=CARTESIAN_POINT('Ctrl Pts',(-159.218520766211,25.3891753238131,182.767891857824));
#93853=CARTESIAN_POINT('Ctrl Pts',(-159.07876131923,25.3903412827711,182.847915451902));
#93854=CARTESIAN_POINT('Ctrl Pts',(-158.938690377899,25.391508366095,182.927294205919));
#93855=CARTESIAN_POINT('Ctrl Pts',(-157.86068685648,25.400490385642,183.538203046421));
#93856=CARTESIAN_POINT('Ctrl Pts',(-156.764294467523,25.4095384825695,184.111040501086));
#93857=CARTESIAN_POINT('Ctrl Pts',(-155.651548955509,25.418630158697,184.650020168367));
#93858=CARTESIAN_POINT('Ctrl Pts',(-155.059253323969,25.4234695042576,184.936909936937));
#93859=CARTESIAN_POINT('Ctrl Pts',(-154.462324779835,25.4283212431225,185.214207771741));
#93860=CARTESIAN_POINT('Ctrl Pts',(-153.861072648507,25.4331822909263,185.482554638578));
#93861=CARTESIAN_POINT('Ctrl Pts',(-153.697444572822,25.4345052033228,185.555584036977));
#93862=CARTESIAN_POINT('Ctrl Pts',(-153.533496042194,25.4358281612412,185.627950279612));
#93863=CARTESIAN_POINT('Ctrl Pts',(-153.369233365809,25.4371510777225,185.699666304073));
#93864=CARTESIAN_POINT('Ctrl Pts',(-152.168980557043,25.446817511129,186.223688934702));
#93865=CARTESIAN_POINT('Ctrl Pts',(-150.951918946651,25.4564813415511,186.712920141648));
#93866=CARTESIAN_POINT('Ctrl Pts',(-149.71990938609,25.4661146840139,187.171200413097));
#93867=CARTESIAN_POINT('Ctrl Pts',(-149.185779282653,25.4702911598878,187.369884982298));
#93868=CARTESIAN_POINT('Ctrl Pts',(-148.648839821616,25.4744619353068,187.562752628899));
#93869=CARTESIAN_POINT('Ctrl Pts',(-148.109243829216,25.4786248717976,187.750119081111));
#93870=CARTESIAN_POINT('Ctrl Pts',(-147.926402504759,25.4800354768286,187.813607933445));
#93871=CARTESIAN_POINT('Ctrl Pts',(-147.743247228578,25.4814447522696,187.876468024315));
#93872=CARTESIAN_POINT('Ctrl Pts',(-147.55978845866,25.4828525510777,187.938709975727));
#93873=CARTESIAN_POINT('Ctrl Pts',(-146.762673408406,25.4889693348008,188.209146740617));
#93874=CARTESIAN_POINT('Ctrl Pts',(-145.959131280017,25.4950633304527,188.468050410514));
#93875=CARTESIAN_POINT('Ctrl Pts',(-145.153130048878,25.5011006913591,188.715270729109));
#93876=CARTESIAN_POINT('Ctrl Pts',(-144.963043743523,25.5025245348775,188.773574854655));
#93877=CARTESIAN_POINT('Ctrl Pts',(-144.772797182542,25.5039455064929,188.831236637802));
#93878=CARTESIAN_POINT('Ctrl Pts',(-144.582440026613,25.5053631356726,188.888254699799));
#93879=CARTESIAN_POINT('Ctrl Pts',(-143.779879218403,25.5113399722913,189.128647353786));
#93880=CARTESIAN_POINT('Ctrl Pts',(-142.974694653033,25.5172625782225,189.357845213595));
#93881=CARTESIAN_POINT('Ctrl Pts',(-142.167290172813,25.5231223320602,189.576786264052));
#93882=CARTESIAN_POINT('Ctrl Pts',(-141.972188592948,25.5245382855994,189.629691277447));
#93883=CARTESIAN_POINT('Ctrl Pts',(-141.776953866285,25.5259504483271,189.681998426253));
#93884=CARTESIAN_POINT('Ctrl Pts',(-141.581589130899,25.5273587560137,189.733721790199));
#93885=CARTESIAN_POINT('Ctrl Pts',(-140.130979976262,25.5378156279707,190.117774649593));
#93886=CARTESIAN_POINT('Ctrl Pts',(-138.673224992468,25.5480587714908,190.469740822773));
#93887=CARTESIAN_POINT('Ctrl Pts',(-137.209373498613,25.5580722003362,190.794332526983));
#93888=CARTESIAN_POINT('Ctrl Pts',(-136.851595170103,25.5605195714322,190.873665627279));
#93889=CARTESIAN_POINT('Ctrl Pts',(-136.493452706413,25.5629532282201,190.951363735793));
#93890=CARTESIAN_POINT('Ctrl Pts',(-136.134961511771,25.5653729519654,191.027496107107));
#93891=CARTESIAN_POINT('Ctrl Pts',(-135.932905732926,25.5667367767211,191.070406465329));
#93892=CARTESIAN_POINT('Ctrl Pts',(-135.730739135609,25.5680958253213,191.112819318821));
#93893=CARTESIAN_POINT('Ctrl Pts',(-135.528464480754,25.5694500469772,191.154747092583));
#93894=CARTESIAN_POINT('Ctrl Pts',(-133.923642813523,25.5801942712463,191.487396775465));
#93895=CARTESIAN_POINT('Ctrl Pts',(-132.31200926945,25.590634688285,191.789469250514));
#93896=CARTESIAN_POINT('Ctrl Pts',(-130.694643085842,25.6007619388848,192.065796528307));
#93897=CARTESIAN_POINT('Ctrl Pts',(-130.475044601821,25.6021369700321,192.103314965327));
#93898=CARTESIAN_POINT('Ctrl Pts',(-130.2553404509,25.6035062306849,192.140358867938));
#93899=CARTESIAN_POINT('Ctrl Pts',(-130.035533347416,25.6048696998908,192.176940401655));
#93900=CARTESIAN_POINT('Ctrl Pts',(-129.830200894786,25.6061433824594,192.211112982614));
#93901=CARTESIAN_POINT('Ctrl Pts',(-129.624774577578,25.6074118350481,192.244882695885));
#93902=CARTESIAN_POINT('Ctrl Pts',(-129.419257839823,25.6086750127158,192.278259225451));
#93903=CARTESIAN_POINT('Ctrl Pts',(-128.048159852991,25.6171022599372,192.50092961714));
#93904=CARTESIAN_POINT('Ctrl Pts',(-126.673077985888,25.6252939765782,192.706038470115));
#93905=CARTESIAN_POINT('Ctrl Pts',(-125.296985611204,25.6332344356778,192.895668467366));
#93906=CARTESIAN_POINT('Ctrl Pts',(-124.827303057514,25.6359446426202,192.960392248272));
#93907=CARTESIAN_POINT('Ctrl Pts',(-124.357502920292,25.6386255864969,193.023313241805));
#93908=CARTESIAN_POINT('Ctrl Pts',(-123.887703735145,25.6412766658778,193.084515551574));
#93909=CARTESIAN_POINT('Ctrl Pts',(-123.682798716099,25.6424329460251,193.111209213133));
#93910=CARTESIAN_POINT('Ctrl Pts',(-123.47788354471,25.6435834960832,193.137577256653));
#93911=CARTESIAN_POINT('Ctrl Pts',(-123.272966987477,25.6447282671046,193.163626730597));
#93912=CARTESIAN_POINT('Ctrl Pts',(-121.444120246373,25.6549451611424,193.396114022849));
#93913=CARTESIAN_POINT('Ctrl Pts',(-119.613568752739,25.6647100991143,193.603766112159));
#93914=CARTESIAN_POINT('Ctrl Pts',(-117.7817201061,25.6740390861231,193.790689645519));
#93915=CARTESIAN_POINT('Ctrl Pts',(-115.810748231209,25.6840765807868,193.991809442007));
#93916=CARTESIAN_POINT('Ctrl Pts',(-113.838274697661,25.6936093935951,194.168932989191));
#93917=CARTESIAN_POINT('Ctrl Pts',(-111.864808666113,25.7026589407586,194.327234715607));
#93918=CARTESIAN_POINT('Ctrl Pts',(-111.760681072972,25.7031364293752,194.335587318337));
#93919=CARTESIAN_POINT('Ctrl Pts',(-111.656550716993,25.7036125728839,194.343887532483));
#93920=CARTESIAN_POINT('Ctrl Pts',(-111.552417673064,25.704087374533,194.352136121901));
#93921=CARTESIAN_POINT('Ctrl Pts',(-111.355686433126,25.7049843839128,194.367719602061));
#93922=CARTESIAN_POINT('Ctrl Pts',(-111.158944291909,25.7058764632696,194.383118901624));
#93923=CARTESIAN_POINT('Ctrl Pts',(-110.962191508823,25.7067636312559,194.398339186358));
#93924=CARTESIAN_POINT('Ctrl Pts',(-108.331895633658,25.7186237648639,194.601812049752));
#93925=CARTESIAN_POINT('Ctrl Pts',(-105.699684895831,25.7296088578491,194.77302215994));
#93926=CARTESIAN_POINT('Ctrl Pts',(-103.066012980214,25.7397901020854,194.919629802492));
#93927=CARTESIAN_POINT('Ctrl Pts',(-101.77346531473,25.744786830566,194.991581576364));
#93928=CARTESIAN_POINT('Ctrl Pts',(-100.480565724247,25.7495899739133,195.057608395254));
#93929=CARTESIAN_POINT('Ctrl Pts',(-99.1873679390386,25.7542081099002,195.118620245283));
#93930=CARTESIAN_POINT('Ctrl Pts',(-99.004725899309,25.7548603425176,195.127237124205));
#93931=CARTESIAN_POINT('Ctrl Pts',(-98.8220779192055,25.7555088353306,195.135753968689));
#93932=CARTESIAN_POINT('Ctrl Pts',(-98.6394241242379,25.7561536103568,195.144173347539));
#93933=CARTESIAN_POINT('Ctrl Pts',(-95.380241384999,25.7676586526498,195.294404522465));
#93934=CARTESIAN_POINT('Ctrl Pts',(-92.1191988411839,25.7779818585862,195.41337897528));
#93935=CARTESIAN_POINT('Ctrl Pts',(-88.8568519213988,25.787260115861,195.510390948637));
#93936=CARTESIAN_POINT('Ctrl Pts',(-88.1724603633154,25.7892065553749,195.530742608725));
#93937=CARTESIAN_POINT('Ctrl Pts',(-87.4880114041535,25.7911070139255,195.550127889636));
#93938=CARTESIAN_POINT('Ctrl Pts',(-86.8035101782839,25.7929627657666,195.568632876457));
#93939=CARTESIAN_POINT('Ctrl Pts',(-86.6388831801868,25.7934090861577,195.573083446179));
#93940=CARTESIAN_POINT('Ctrl Pts',(-86.4742531510357,25.7938528048312,195.577483095995));
#93941=CARTESIAN_POINT('Ctrl Pts',(-86.3096201486703,25.7942939388959,195.581833024548));
#93942=CARTESIAN_POINT('Ctrl Pts',(-82.3438711834279,25.8049201616776,195.686615932032));
#93943=CARTESIAN_POINT('Ctrl Pts',(-78.3763910652539,25.81404753251,195.762354575598));
#93944=CARTESIAN_POINT('Ctrl Pts',(-74.4078298020737,25.821907197684,195.819882597081));
#93945=CARTESIAN_POINT('Ctrl Pts',(-74.263798022696,25.8221924500678,195.821970472951));
#93946=CARTESIAN_POINT('Ctrl Pts',(-74.1197648633499,25.8224760292359,195.824034366091));
#93947=CARTESIAN_POINT('Ctrl Pts',(-73.9757303467128,25.8227579460834,195.82607479565));
#93948=CARTESIAN_POINT('Ctrl Pts',(-68.3928699838828,25.8336852045642,195.90516301405));
#93949=CARTESIAN_POINT('Ctrl Pts',(-62.8094936979019,25.8421199931682,195.950045641758));
#93950=CARTESIAN_POINT('Ctrl Pts',(-57.2260685167664,25.8486341168402,195.976904270453));
#93951=CARTESIAN_POINT('Ctrl Pts',(-54.6859273035473,25.8515976729854,195.98912342043));
#93952=CARTESIAN_POINT('Ctrl Pts',(-52.1457759576179,25.8541637485837,195.997612920801));
#93953=CARTESIAN_POINT('Ctrl Pts',(-49.605658395478,25.8563863803193,196.003899767975));
#93954=CARTESIAN_POINT('Ctrl Pts',(-49.5072967943702,25.8564724478381,196.004143215114));
#93955=CARTESIAN_POINT('Ctrl Pts',(-49.4089352305451,25.8565579998157,196.004383359602));
#93956=CARTESIAN_POINT('Ctrl Pts',(-49.310573704736,25.8566430393848,196.004620290147));
#93957=CARTESIAN_POINT('Ctrl Pts',(-41.1414030558168,25.8637057882182,196.024297964312));
#93958=CARTESIAN_POINT('Ctrl Pts',(-32.9721411092781,25.8672091692298,196.020124461517));
#93959=CARTESIAN_POINT('Ctrl Pts',(-24.8028804680956,25.8688484080511,196.014152702805));
#93960=CARTESIAN_POINT('Ctrl Pts',(-24.7530540772718,25.8688584061841,196.014116279535));
#93961=CARTESIAN_POINT('Ctrl Pts',(-24.7032276851075,25.868868334986,196.014079789476));
#93962=CARTESIAN_POINT('Ctrl Pts',(-24.6534012915206,25.8688781948416,196.014043237634));
#93963=CARTESIAN_POINT('Ctrl Pts',(-16.435603976083,25.8705043670193,196.008014793532));
#93964=CARTESIAN_POINT('Ctrl Pts',(-8.21780260152389,25.8701893108446,195.999534166345));
#93965=CARTESIAN_POINT('Ctrl Pts',(1.55981000190379E-14,25.8701893108725,
195.999534166346));
#93966=CARTESIAN_POINT('',(-177.813017113379,24.8757620423259,152.608250755187));
#93967=CARTESIAN_POINT('Origin',(-177.813017113379,25.8757620423259,152.608250755187));
#93968=CARTESIAN_POINT('Ctrl Pts',(1.54046147636829E-14,24.8757620423259,
194.999549694134));
#93969=CARTESIAN_POINT('Ctrl Pts',(-8.21488588608219,24.8757620423259,194.999549694362));
#93970=CARTESIAN_POINT('Ctrl Pts',(-16.4297691665589,24.8757620423259,195.008020860107));
#93971=CARTESIAN_POINT('Ctrl Pts',(-24.6446497557777,24.8757620423259,195.01406045846));
#93972=CARTESIAN_POINT('Ctrl Pts',(-24.64781191049,24.8757620423259,195.014062783283));
#93973=CARTESIAN_POINT('Ctrl Pts',(-24.6509740652016,24.8757620423259,195.014065107746));
#93974=CARTESIAN_POINT('Ctrl Pts',(-24.6541362199128,24.8757620423259,195.014067431847));
#93975=CARTESIAN_POINT('Ctrl Pts',(-32.8658546514293,24.875762042326,195.020102831808));
#93976=CARTESIAN_POINT('Ctrl Pts',(-41.0775680296323,24.8757620423251,195.024458577496));
#93977=CARTESIAN_POINT('Ctrl Pts',(-49.2892094763632,24.8757620423267,195.004852527973));
#93978=CARTESIAN_POINT('Ctrl Pts',(-49.2955336215858,24.8757620423267,195.004837428495));
#93979=CARTESIAN_POINT('Ctrl Pts',(-49.301857766761,24.8757620423267,195.004822314801));
#93980=CARTESIAN_POINT('Ctrl Pts',(-49.3081819118888,24.8757620423267,195.004807186881));
#93981=CARTESIAN_POINT('Ctrl Pts',(-57.5166612154801,24.8757620423282,194.985171771549));
#93982=CARTESIAN_POINT('Ctrl Pts',(-65.7254697695311,24.8757620423215,194.943230036326));
#93983=CARTESIAN_POINT('Ctrl Pts',(-73.9332331952951,24.8757620423304,194.827982077321));
#93984=CARTESIAN_POINT('Ctrl Pts',(-73.9427185287022,24.8757620423304,194.827848890574));
#93985=CARTESIAN_POINT('Ctrl Pts',(-73.9522038606495,24.8757620423304,194.827715605884));
#93986=CARTESIAN_POINT('Ctrl Pts',(-73.961689191135,24.8757620423304,194.827582223175));
#93987=CARTESIAN_POINT('Ctrl Pts',(-78.059246105284,24.8757620423347,194.769962381229));
#93988=CARTESIAN_POINT('Ctrl Pts',(-82.1556895284227,24.8757620423252,194.693493289495));
#93989=CARTESIAN_POINT('Ctrl Pts',(-86.2503383467373,24.8757620423266,194.58636884538));
#93990=CARTESIAN_POINT('Ctrl Pts',(-86.2613966994682,24.8757620423266,194.586079536104));
#93991=CARTESIAN_POINT('Ctrl Pts',(-86.2724550390773,24.8757620423266,194.585790003169));
#93992=CARTESIAN_POINT('Ctrl Pts',(-86.2835133655508,24.8757620423266,194.585500246345));
#93993=CARTESIAN_POINT('Ctrl Pts',(-90.3765727109929,24.875762042328,194.478251479603));
#93994=CARTESIAN_POINT('Ctrl Pts',(-94.4678439707547,24.8757620423236,194.340526346086));
#93995=CARTESIAN_POINT('Ctrl Pts',(-98.5562591476545,24.8757620423282,194.154116211922));
#93996=CARTESIAN_POINT('Ctrl Pts',(-98.5688828803835,24.8757620423282,194.153540636397));
#93997=CARTESIAN_POINT('Ctrl Pts',(-98.5815065858776,24.8757620423282,194.152964596616));
#93998=CARTESIAN_POINT('Ctrl Pts',(-98.5941302641051,24.8757620423282,194.152388092042));
#93999=CARTESIAN_POINT('Ctrl Pts',(-102.680949843047,24.8757620423327,193.965749131845));
#94000=CARTESIAN_POINT('Ctrl Pts',(-106.764931224453,24.8757620423183,193.730731754961));
#94001=CARTESIAN_POINT('Ctrl Pts',(-110.84440359735,24.8757620423337,193.418858454368));
#94002=CARTESIAN_POINT('Ctrl Pts',(-110.858579691179,24.8757620423337,193.417774700204));
#94003=CARTESIAN_POINT('Ctrl Pts',(-110.872755730562,24.8757620423338,193.416690017724));
#94004=CARTESIAN_POINT('Ctrl Pts',(-110.886931715427,24.8757620423338,193.415604405734));
#94005=CARTESIAN_POINT('Ctrl Pts',(-114.96479763357,24.875762042349,193.103317098939));
#94006=CARTESIAN_POINT('Ctrl Pts',(-119.03818825583,24.8757620423139,192.714732197115));
#94007=CARTESIAN_POINT('Ctrl Pts',(-123.104423976305,24.8757620423383,192.204214021647));
#94008=CARTESIAN_POINT('Ctrl Pts',(-123.120130138159,24.8757620423384,192.202242104217));
#94009=CARTESIAN_POINT('Ctrl Pts',(-123.135836193123,24.8757620423385,192.20026836683));
#94010=CARTESIAN_POINT('Ctrl Pts',(-123.151542141045,24.8757620423386,192.198292806863));
#94011=CARTESIAN_POINT('Ctrl Pts',(-125.175994041311,24.8757620423502,191.943648760649));
#94012=CARTESIAN_POINT('Ctrl Pts',(-127.200620383331,24.8757620423257,191.658066442003));
#94013=CARTESIAN_POINT('Ctrl Pts',(-129.217100987035,24.8757620423261,191.334701322639));
#94014=CARTESIAN_POINT('Ctrl Pts',(-129.233527280793,24.8757620423261,191.332067183519));
#94015=CARTESIAN_POINT('Ctrl Pts',(-129.249953033335,24.8757620423261,191.329430536661));
#94016=CARTESIAN_POINT('Ctrl Pts',(-129.266378240165,24.8757620423261,191.326791378358));
#94017=CARTESIAN_POINT('Ctrl Pts',(-131.281943276968,24.8757620423265,191.00293577899));
#94018=CARTESIAN_POINT('Ctrl Pts',(-133.289200652704,24.8757620423246,190.641384293948));
#94019=CARTESIAN_POINT('Ctrl Pts',(-135.286079698496,24.8757620423273,190.232703307421));
#94020=CARTESIAN_POINT('Ctrl Pts',(-135.303127536398,24.8757620423273,190.229214299298));
#94021=CARTESIAN_POINT('Ctrl Pts',(-135.320174617604,24.8757620423273,190.225721855634));
#94022=CARTESIAN_POINT('Ctrl Pts',(-135.337220940819,24.8757620423273,190.222225970564));
#94023=CARTESIAN_POINT('Ctrl Pts',(-137.333147727731,24.8757620423299,189.812898365584));
#94024=CARTESIAN_POINT('Ctrl Pts',(-139.31869551455,24.8757620423247,189.356449033943));
#94025=CARTESIAN_POINT('Ctrl Pts',(-141.291204979638,24.8757620423271,188.840805830176));
#94026=CARTESIAN_POINT('Ctrl Pts',(-141.308817044353,24.8757620423272,188.836201775475));
#94027=CARTESIAN_POINT('Ctrl Pts',(-141.326428069381,24.8757620423272,188.831593000313));
#94028=CARTESIAN_POINT('Ctrl Pts',(-141.344038052832,24.8757620423272,188.826979496123));
#94029=CARTESIAN_POINT('Ctrl Pts',(-142.320988421435,24.8757620423283,188.571035779219));
#94030=CARTESIAN_POINT('Ctrl Pts',(-143.294722983287,24.8757620423258,188.300491718125));
#94031=CARTESIAN_POINT('Ctrl Pts',(-144.264847386162,24.875762042326,188.013557547871));
#94032=CARTESIAN_POINT('Ctrl Pts',(-144.282714465166,24.875762042326,188.008272993154));
#94033=CARTESIAN_POINT('Ctrl Pts',(-144.300580331459,24.875762042326,188.002982874821));
#94034=CARTESIAN_POINT('Ctrl Pts',(-144.318444981918,24.875762042326,187.997687181806));
#94035=CARTESIAN_POINT('Ctrl Pts',(-145.288057437586,24.8757620423261,187.710260908361));
#94036=CARTESIAN_POINT('Ctrl Pts',(-146.255054777119,24.8757620423277,187.406047757954));
#94037=CARTESIAN_POINT('Ctrl Pts',(-147.212983965987,24.8757620423268,187.085108796902));
#94038=CARTESIAN_POINT('Ctrl Pts',(-147.23100919069,24.8757620423268,187.079069731639));
#94039=CARTESIAN_POINT('Ctrl Pts',(-147.249031241071,24.8757620423268,187.073024733291));
#94040=CARTESIAN_POINT('Ctrl Pts',(-147.267050074644,24.8757620423268,187.066973802089));
#94041=CARTESIAN_POINT('Ctrl Pts',(-149.083477336966,24.8757620423251,186.456996671566));
#94042=CARTESIAN_POINT('Ctrl Pts',(-150.870857453158,24.8757620423225,185.785994488404));
#94043=CARTESIAN_POINT('Ctrl Pts',(-152.623123968799,24.8757620423294,185.041686563971));
#94044=CARTESIAN_POINT('Ctrl Pts',(-152.73504513073,24.8757620423299,184.994145960419));
#94045=CARTESIAN_POINT('Ctrl Pts',(-152.846823049118,24.8757620423304,184.946306310615));
#94046=CARTESIAN_POINT('Ctrl Pts',(-152.958456146666,24.875762042331,184.898164421556));
#94047=CARTESIAN_POINT('Ctrl Pts',(-152.976515861628,24.8757620423311,184.890376150755));
#94048=CARTESIAN_POINT('Ctrl Pts',(-152.994571791993,24.8757620423311,184.882579966051));
#94049=CARTESIAN_POINT('Ctrl Pts',(-153.012623931258,24.8757620423312,184.874775853854));
#94050=CARTESIAN_POINT('Ctrl Pts',(-154.870511769106,24.8757620423408,184.071593199207));
#94051=CARTESIAN_POINT('Ctrl Pts',(-156.688325422377,24.8757620423189,183.1846136828));
#94052=CARTESIAN_POINT('Ctrl Pts',(-158.456781621831,24.8757620423332,182.194428286473));
#94053=CARTESIAN_POINT('Ctrl Pts',(-158.47465212741,24.8757620423334,182.184422319882));
#94054=CARTESIAN_POINT('Ctrl Pts',(-158.492517591448,24.8757620423335,182.174405810671));
#94055=CARTESIAN_POINT('Ctrl Pts',(-158.510378004392,24.8757620423336,182.164378738907));
#94056=CARTESIAN_POINT('Ctrl Pts',(-159.384833046953,24.8757620423397,181.673448126429));
#94057=CARTESIAN_POINT('Ctrl Pts',(-160.247140085049,24.8757620423256,181.157114890314));
#94058=CARTESIAN_POINT('Ctrl Pts',(-161.095845403919,24.8757620423262,180.612340916905));
#94059=CARTESIAN_POINT('Ctrl Pts',(-161.113513241408,24.8757620423262,180.601000139586));
#94060=CARTESIAN_POINT('Ctrl Pts',(-161.131175182557,24.8757620423262,180.589647032195));
#94061=CARTESIAN_POINT('Ctrl Pts',(-161.148831214264,24.8757620423262,180.578281567396));
#94062=CARTESIAN_POINT('Ctrl Pts',(-161.563905737138,24.8757620423264,180.311091580601));
#94063=CARTESIAN_POINT('Ctrl Pts',(-161.975710072057,24.8757620423259,180.037063261309));
#94064=CARTESIAN_POINT('Ctrl Pts',(-162.384044953281,24.8757620423259,179.755780375325));
#94065=CARTESIAN_POINT('Ctrl Pts',(-162.401578082186,24.8757620423259,179.743702619234));
#94066=CARTESIAN_POINT('Ctrl Pts',(-162.419104898429,24.8757620423259,179.731611433976));
#94067=CARTESIAN_POINT('Ctrl Pts',(-162.436625375847,24.8757620423259,179.719506792461));
#94068=CARTESIAN_POINT('Ctrl Pts',(-162.844501949097,24.875762042326,179.437710835434));
#94069=CARTESIAN_POINT('Ctrl Pts',(-163.249423819711,24.8757620423319,179.148232630283));
#94070=CARTESIAN_POINT('Ctrl Pts',(-163.64800894658,24.8757620423299,178.85302979587));
#94071=CARTESIAN_POINT('Ctrl Pts',(-163.665291233915,24.8757620423298,178.840230070385));
#94072=CARTESIAN_POINT('Ctrl Pts',(-163.682561810057,24.8757620423297,178.827419445818));
#94073=CARTESIAN_POINT('Ctrl Pts',(-163.699820408872,24.8757620423297,178.814598075025));
#94074=CARTESIAN_POINT('Ctrl Pts',(-164.709308917564,24.875762042325,178.064651534152));
#94075=CARTESIAN_POINT('Ctrl Pts',(-165.681737714684,24.8757620423251,177.275740093117));
#94076=CARTESIAN_POINT('Ctrl Pts',(-166.613250849857,24.8757620423274,176.444043333016));
#94077=CARTESIAN_POINT('Ctrl Pts',(-167.198094243251,24.8757620423289,175.921868886853));
#94078=CARTESIAN_POINT('Ctrl Pts',(-167.766809867722,24.8757620423314,175.382829696395));
#94079=CARTESIAN_POINT('Ctrl Pts',(-168.318450873044,24.8757620423482,174.825987926454));
#94080=CARTESIAN_POINT('Ctrl Pts',(-168.334027852459,24.8757620423487,174.810264090293));
#94081=CARTESIAN_POINT('Ctrl Pts',(-168.349591230718,24.8757620423491,174.794526036491));
#94082=CARTESIAN_POINT('Ctrl Pts',(-168.365140987195,24.8757620423495,174.77877374356));
#94083=CARTESIAN_POINT('Ctrl Pts',(-169.070974410657,24.8757620423678,174.063746800061));
#94084=CARTESIAN_POINT('Ctrl Pts',(-169.748646290608,24.8757620423234,173.319282963081));
#94085=CARTESIAN_POINT('Ctrl Pts',(-170.395306107718,24.8757620423285,172.542403589941));
#94086=CARTESIAN_POINT('Ctrl Pts',(-170.409806583172,24.8757620423286,172.524983116328));
#94087=CARTESIAN_POINT('Ctrl Pts',(-170.424291533727,24.8757620423288,172.507546270103));
#94088=CARTESIAN_POINT('Ctrl Pts',(-170.43876092208,24.875762042329,172.490093021554));
#94089=CARTESIAN_POINT('Ctrl Pts',(-170.88928987737,24.8757620423346,171.946656516614));
#94090=CARTESIAN_POINT('Ctrl Pts',(-171.325552583136,24.8757620424712,171.385736098847));
#94091=CARTESIAN_POINT('Ctrl Pts',(-171.741692841451,24.8757620425566,170.813322812391));
#94092=CARTESIAN_POINT('Ctrl Pts',(-171.921338161584,24.8757620425934,170.566215338314));
#94093=CARTESIAN_POINT('Ctrl Pts',(-172.09723391366,24.8757620425925,170.316966519992));
#94094=CARTESIAN_POINT('Ctrl Pts',(-172.268911669619,24.8757620425312,170.066059798355));
#94095=CARTESIAN_POINT('Ctrl Pts',(-172.28190915054,24.8757620425265,170.047064004118));
#94096=CARTESIAN_POINT('Ctrl Pts',(-172.294882644394,24.8757620425221,170.028058474253));
#94097=CARTESIAN_POINT('Ctrl Pts',(-172.307831949918,24.8757620425178,170.009043413777));
#94098=CARTESIAN_POINT('Ctrl Pts',(-172.881333308836,24.8757620423296,169.166900721047));
#94099=CARTESIAN_POINT('Ctrl Pts',(-173.410591971626,24.8757620423975,168.302660920235));
#94100=CARTESIAN_POINT('Ctrl Pts',(-173.893716192591,24.8757620424271,167.415541053399));
#94101=CARTESIAN_POINT('Ctrl Pts',(-174.376840413556,24.8757620424566,166.528421186564));
#94102=CARTESIAN_POINT('Ctrl Pts',(-174.813829816887,24.875762042452,165.618421053482));
#94103=CARTESIAN_POINT('Ctrl Pts',(-175.202841307782,24.8757620423681,164.684786982141));
#94104=CARTESIAN_POINT('Ctrl Pts',(-175.211927010215,24.8757620423662,164.662981144647));
#94105=CARTESIAN_POINT('Ctrl Pts',(-175.220986583199,24.8757620423644,164.641162380823));
#94106=CARTESIAN_POINT('Ctrl Pts',(-175.230020003396,24.8757620423629,164.619330678862));
#94107=CARTESIAN_POINT('Ctrl Pts',(-175.612126116306,24.8757620422975,163.695867960076));
#94108=CARTESIAN_POINT('Ctrl Pts',(-175.947287153428,24.8757620424648,162.749178442011));
#94109=CARTESIAN_POINT('Ctrl Pts',(-176.237555075868,24.8757620423541,161.780272945005));
#94110=CARTESIAN_POINT('Ctrl Pts',(-176.244531782355,24.8757620423515,161.756984910939));
#94111=CARTESIAN_POINT('Ctrl Pts',(-176.251482514742,24.8757620423493,161.733684386156));
#94112=CARTESIAN_POINT('Ctrl Pts',(-176.258407335464,24.8757620423475,161.710371268223));
#94113=CARTESIAN_POINT('Ctrl Pts',(-176.360806953651,24.8757620423206,161.365632469767));
#94114=CARTESIAN_POINT('Ctrl Pts',(-176.457676806858,24.8757620423462,161.017688127655));
#94115=CARTESIAN_POINT('Ctrl Pts',(-176.548849501517,24.8757620423492,160.668545469221));
#94116=CARTESIAN_POINT('Ctrl Pts',(-176.582804133289,24.8757620423503,160.538517389574));
#94117=CARTESIAN_POINT('Ctrl Pts',(-176.615968076816,24.8757620423472,160.408323068285));
#94118=CARTESIAN_POINT('Ctrl Pts',(-176.648330823726,24.8757620423399,160.278066605508));
#94119=CARTESIAN_POINT('Ctrl Pts',(-176.654186619902,24.8757620423386,160.254497676123));
#94120=CARTESIAN_POINT('Ctrl Pts',(-176.660016327933,24.8757620423374,160.230926318362));
#94121=CARTESIAN_POINT('Ctrl Pts',(-176.665819842891,24.8757620423364,160.207353312146));
#94122=CARTESIAN_POINT('Ctrl Pts',(-176.768995240264,24.875762042318,159.788270342399));
#94123=CARTESIAN_POINT('Ctrl Pts',(-176.86420175272,24.8757620423259,159.367762185166));
#94124=CARTESIAN_POINT('Ctrl Pts',(-176.952169714707,24.8757620423259,158.946132895978));
#94125=CARTESIAN_POINT('Ctrl Pts',(-176.964994102294,24.875762042326,158.884665774307));
#94126=CARTESIAN_POINT('Ctrl Pts',(-176.977664737325,24.875762042326,158.823174832625));
#94127=CARTESIAN_POINT('Ctrl Pts',(-176.990183971956,24.875762042326,158.761661020592));
#94128=CARTESIAN_POINT('Ctrl Pts',(-176.99465092232,24.875762042326,158.739712462785));
#94129=CARTESIAN_POINT('Ctrl Pts',(-176.999098629657,24.875762042326,158.717760829857));
#94130=CARTESIAN_POINT('Ctrl Pts',(-177.003527206417,24.8757620423261,158.695806137836));
#94131=CARTESIAN_POINT('Ctrl Pts',(-177.118219982101,24.8757620423264,158.127216113678));
#94132=CARTESIAN_POINT('Ctrl Pts',(-177.220333395014,24.8757620423267,157.556593568297));
#94133=CARTESIAN_POINT('Ctrl Pts',(-177.311324060744,24.8757620423267,156.984178905084));
#94134=CARTESIAN_POINT('Ctrl Pts',(-177.404696611944,24.8757620423267,156.396779999712));
#94135=CARTESIAN_POINT('Ctrl Pts',(-177.486356724851,24.8757620423264,155.807493942056));
#94136=CARTESIAN_POINT('Ctrl Pts',(-177.557934404858,24.8757620423262,155.216584754304));
#94137=CARTESIAN_POINT('Ctrl Pts',(-177.632922386434,24.875762042326,154.597521838599));
#94138=CARTESIAN_POINT('Ctrl Pts',(-177.69684448066,24.8757620423259,153.976677454172));
#94139=CARTESIAN_POINT('Ctrl Pts',(-177.751632462613,24.8757620423259,153.354359553465));
#94140=CARTESIAN_POINT('Ctrl Pts',(-177.77350781823,24.8757620423259,153.105884889862));
#94141=CARTESIAN_POINT('Ctrl Pts',(-177.793927627997,24.8757620423259,152.857175365898));
#94142=CARTESIAN_POINT('Ctrl Pts',(-177.813017113379,24.8757620423259,152.608250755187));
#94143=CARTESIAN_POINT('Ctrl Pts',(-175.73950529146,23.8567983454203,151.608424919145));
#94144=CARTESIAN_POINT('Ctrl Pts',(-176.388687107557,23.0874449616485,151.623023103975));
#94145=CARTESIAN_POINT('Ctrl Pts',(-176.384335038167,23.0735478218188,150.616361820745));
#94146=CARTESIAN_POINT('Ctrl Pts',(-176.003304916941,23.9680637154176,151.606384577597));
#94147=CARTESIAN_POINT('Ctrl Pts',(-176.593854313756,23.2639762965151,151.537709600337));
#94148=CARTESIAN_POINT('Ctrl Pts',(-176.656254705308,23.3029629324784,150.615565005799));
#94149=CARTESIAN_POINT('Ctrl Pts',(-176.258810630189,24.0795828100808,151.622206832873));
#94150=CARTESIAN_POINT('Ctrl Pts',(-176.815150128392,23.4580026124915,151.487215027469));
#94151=CARTESIAN_POINT('Ctrl Pts',(-176.919885733397,23.5331341645717,150.650684462557));
#94152=CARTESIAN_POINT('Ctrl Pts',(-176.736237334262,24.2964053110708,151.694271183075));
#94153=CARTESIAN_POINT('Ctrl Pts',(-177.237181962352,23.8405921073048,151.47948246492));
#94154=CARTESIAN_POINT('Ctrl Pts',(-177.413116931558,23.9811970433833,150.802131799252));
#94155=CARTESIAN_POINT('Ctrl Pts',(-176.962392794808,24.4033211362568,151.749272834437));
#94156=CARTESIAN_POINT('Ctrl Pts',(-177.443743421448,24.0332847294644,151.513241822621));
#94157=CARTESIAN_POINT('Ctrl Pts',(-177.647053524624,24.2023887513038,150.91600535664));
#94158=CARTESIAN_POINT('Ctrl Pts',(-177.261937401879,24.5519309185043,151.868767106029));
#94159=CARTESIAN_POINT('Ctrl Pts',(-177.721629599937,24.3032107970142,151.639069912478));
#94160=CARTESIAN_POINT('Ctrl Pts',(-177.957529153403,24.5103483072772,151.161146031839));
#94161=CARTESIAN_POINT('Ctrl Pts',(-177.356706714869,24.6002596109534,151.9155000569));
#94162=CARTESIAN_POINT('Ctrl Pts',(-177.809527175111,24.3904184950665,151.692946627691));
#94163=CARTESIAN_POINT('Ctrl Pts',(-178.055876609326,24.6105915832425,151.256755643874));
#94164=CARTESIAN_POINT('Ctrl Pts',(-177.525039051065,24.6888716230439,152.02203145606));
#94165=CARTESIAN_POINT('Ctrl Pts',(-177.965962925957,24.5495763065596,151.825376775102));
#94166=CARTESIAN_POINT('Ctrl Pts',(-178.230880519265,24.7946312006147,151.474169337755));
#94167=CARTESIAN_POINT('Ctrl Pts',(-177.598939664808,24.7292916556483,152.081679209295));
#94168=CARTESIAN_POINT('Ctrl Pts',(-178.035464730705,24.6223780008855,151.90353429491));
#94169=CARTESIAN_POINT('Ctrl Pts',(-178.307882838118,24.8787077221551,151.595672377231));
#94170=CARTESIAN_POINT('Ctrl Pts',(-177.720286934346,24.7991411953602,152.216892436631));
#94171=CARTESIAN_POINT('Ctrl Pts',(-178.149684748747,24.7467279407185,152.086964131903));
#94172=CARTESIAN_POINT('Ctrl Pts',(-178.434830427082,25.0243673086006,151.870608949261));
#94173=CARTESIAN_POINT('Ctrl Pts',(-177.765084499851,24.8270347155314,152.289484845931));
#94174=CARTESIAN_POINT('Ctrl Pts',(-178.192532655266,24.7961598874315,152.188512755172));
#94175=CARTESIAN_POINT('Ctrl Pts',(-178.482003941885,25.0827471702104,152.017997656931));
#94176=CARTESIAN_POINT('Ctrl Pts',(-177.821660312508,24.8682175857358,152.455831581551));
#94177=CARTESIAN_POINT('Ctrl Pts',(-178.247166957742,24.8667382439783,152.423392974383));
#94178=CARTESIAN_POINT('Ctrl Pts',(-178.542611941005,25.1696189974259,152.355268021077));
#94179=CARTESIAN_POINT('Ctrl Pts',(-177.826854605526,24.8780047222983,152.546670848957));
#94180=CARTESIAN_POINT('Ctrl Pts',(-178.253157647747,24.8819396453427,152.553901526939));
#94181=CARTESIAN_POINT('Ctrl Pts',(-178.549220219017,25.1908520618554,152.539188683824));
#94182=CARTESIAN_POINT('Ctrl Pts',(-177.807677777613,24.8753312313243,152.637557271751));
#94183=CARTESIAN_POINT('Ctrl Pts',(-178.236377845671,24.87399890951,152.682737783154));
#94184=CARTESIAN_POINT('Ctrl Pts',(-178.53072563814,25.1863823136132,152.722941452113));
#94185=CARTESIAN_POINT('',(-176.430593086108,23.1126512166031,150.616656461876));
#94186=CARTESIAN_POINT('',(-175.784380109018,23.8757620423259,151.608250755187));
#94187=CARTESIAN_POINT('Origin',(-175.784380109018,23.8757620423259,150.608250755187));
#94188=CARTESIAN_POINT('Ctrl Pts',(-175.784380109018,23.8757620423259,151.608250755187));
#94189=CARTESIAN_POINT('Ctrl Pts',(-175.888159349634,23.9197029023221,151.608250755187));
#94190=CARTESIAN_POINT('Ctrl Pts',(-175.991448416971,23.9640264362152,151.611061269963));
#94191=CARTESIAN_POINT('Ctrl Pts',(-176.094195590625,24.008769736127,151.617048131169));
#94192=CARTESIAN_POINT('Ctrl Pts',(-176.19694276428,24.0535130360388,151.623034992374));
#94193=CARTESIAN_POINT('Ctrl Pts',(-176.299148251002,24.098676111631,151.6321977244));
#94194=CARTESIAN_POINT('Ctrl Pts',(-176.400736032712,24.1442953670243,151.644955074084));
#94195=CARTESIAN_POINT('Ctrl Pts',(-176.435432451251,24.1598762247998,151.649312235315));
#94196=CARTESIAN_POINT('Ctrl Pts',(-176.470014453398,24.1754907487728,151.654083487016));
#94197=CARTESIAN_POINT('Ctrl Pts',(-176.504510507143,24.1911550184597,151.659289601702));
#94198=CARTESIAN_POINT('Ctrl Pts',(-176.560530785521,24.2165931962569,151.667744133809));
#94199=CARTESIAN_POINT('Ctrl Pts',(-176.616510806086,24.242257960854,151.677408353266));
#94200=CARTESIAN_POINT('Ctrl Pts',(-176.672282380912,24.2680844183909,151.688422405043));
#94201=CARTESIAN_POINT('Ctrl Pts',(-176.724797335908,24.2924028146258,151.698793323118));
#94202=CARTESIAN_POINT('Ctrl Pts',(-176.777128105327,24.3168648944967,151.710361068092));
#94203=CARTESIAN_POINT('Ctrl Pts',(-176.82910008493,24.3414050138239,151.723270748686));
#94204=CARTESIAN_POINT('Ctrl Pts',(-176.877613351544,24.364311998718,151.735321295565));
#94205=CARTESIAN_POINT('Ctrl Pts',(-176.925814331434,24.3872871657492,151.748541188469));
#94206=CARTESIAN_POINT('Ctrl Pts',(-176.973523867365,24.410263427155,151.76307286238));
#94207=CARTESIAN_POINT('Ctrl Pts',(-176.982726986036,24.4146955235108,151.765876006801));
#94208=CARTESIAN_POINT('Ctrl Pts',(-176.991911691641,24.4191276124988,151.768728038266));
#94209=CARTESIAN_POINT('Ctrl Pts',(-177.001076508298,24.4235591398025,151.771630090036));
#94210=CARTESIAN_POINT('Ctrl Pts',(-177.042173845054,24.4434312198195,151.784643618111));
#94211=CARTESIAN_POINT('Ctrl Pts',(-177.082911866297,24.4633059029067,151.79866930332));
#94212=CARTESIAN_POINT('Ctrl Pts',(-177.123173784831,24.4831461072352,151.813841057898));
#94213=CARTESIAN_POINT('Ctrl Pts',(-177.13619974057,24.4895650170348,151.818749582151));
#94214=CARTESIAN_POINT('Ctrl Pts',(-177.149175539937,24.4959801962463,151.823778263238));
#94215=CARTESIAN_POINT('Ctrl Pts',(-177.162096243315,24.5023900130613,151.828932215432));
#94216=CARTESIAN_POINT('Ctrl Pts',(-177.196296802062,24.519356528747,151.842574510253));
#94217=CARTESIAN_POINT('Ctrl Pts',(-177.230294880457,24.5363753306636,151.857180131003));
#94218=CARTESIAN_POINT('Ctrl Pts',(-177.263867635009,24.5533452343922,151.872819968914));
#94219=CARTESIAN_POINT('Ctrl Pts',(-177.27137398005,24.5571394405689,151.876316793089));
#94220=CARTESIAN_POINT('Ctrl Pts',(-177.278858881439,24.5609311195225,151.879865361306));
#94221=CARTESIAN_POINT('Ctrl Pts',(-177.286319519695,24.5647189898801,151.883466541106));
#94222=CARTESIAN_POINT('Ctrl Pts',(-177.314373267698,24.5789622699892,151.897007820972));
#94223=CARTESIAN_POINT('Ctrl Pts',(-177.342131087439,24.5931782747943,151.911315989472));
#94224=CARTESIAN_POINT('Ctrl Pts',(-177.369451368433,24.6073035761847,151.926466315716));
#94225=CARTESIAN_POINT('Ctrl Pts',(-177.393647488778,24.6198136046291,151.939884154176));
#94226=CARTESIAN_POINT('Ctrl Pts',(-177.417500241383,24.6322524359504,151.953962709686));
#94227=CARTESIAN_POINT('Ctrl Pts',(-177.440880693276,24.6445625833218,151.968762109259));
#94228=CARTESIAN_POINT('Ctrl Pts',(-177.466603695553,24.6581061174811,151.985044300496));
#94229=CARTESIAN_POINT('Ctrl Pts',(-177.491786560729,24.6715066684446,152.002183768001));
#94230=CARTESIAN_POINT('Ctrl Pts',(-177.516292176977,24.6847047655833,152.020331144545));
#94231=CARTESIAN_POINT('Ctrl Pts',(-177.527198432,24.6905785951475,152.028407657071));
#94232=CARTESIAN_POINT('Ctrl Pts',(-177.537970014763,24.6964120880033,152.036684115516));
#94233=CARTESIAN_POINT('Ctrl Pts',(-177.548592113994,24.7021987720431,152.045175385715));
#94234=CARTESIAN_POINT('Ctrl Pts',(-177.568202820616,24.7128822500032,152.060852118261));
#94235=CARTESIAN_POINT('Ctrl Pts',(-177.587313346476,24.7234120143457,152.077266089796));
#94236=CARTESIAN_POINT('Ctrl Pts',(-177.605849017592,24.7337606599818,152.094564516487));
#94237=CARTESIAN_POINT('Ctrl Pts',(-177.624384688707,24.744109305618,152.111862943177));
#94238=CARTESIAN_POINT('Ctrl Pts',(-177.642346062884,24.7542771121623,152.130045515296));
#94239=CARTESIAN_POINT('Ctrl Pts',(-177.659613299577,24.7642164255042,152.149285822963));
#94240=CARTESIAN_POINT('Ctrl Pts',(-177.675506713529,24.7733649432519,152.166995325632));
#94241=CARTESIAN_POINT('Ctrl Pts',(-177.690630352488,24.782214663373,152.18539780105));
#94242=CARTESIAN_POINT('Ctrl Pts',(-177.704840532489,24.7906991998897,152.204610352547));
#94243=CARTESIAN_POINT('Ctrl Pts',(-177.718477366732,24.798841406259,152.22304772492));
#94244=CARTESIAN_POINT('Ctrl Pts',(-177.731273086947,24.8066473872866,152.242231073656));
#94245=CARTESIAN_POINT('Ctrl Pts',(-177.743059463349,24.8140378964531,152.26227770449));
#94246=CARTESIAN_POINT('Ctrl Pts',(-177.747198803758,24.8166334213367,152.269318021739));
#94247=CARTESIAN_POINT('Ctrl Pts',(-177.751213259865,24.8191775046934,152.276464947716));
#94248=CARTESIAN_POINT('Ctrl Pts',(-177.755094216052,24.8216660422822,152.283724011869));
#94249=CARTESIAN_POINT('Ctrl Pts',(-177.766667220852,24.8290868571729,152.305370528925));
#94250=CARTESIAN_POINT('Ctrl Pts',(-177.776998408874,24.8359795863142,152.32792109276));
#94251=CARTESIAN_POINT('Ctrl Pts',(-177.785818285655,24.8421983688494,152.351336130936));
#94252=CARTESIAN_POINT('Ctrl Pts',(-177.787884465384,24.8436552058024,152.356821431744));
#94253=CARTESIAN_POINT('Ctrl Pts',(-177.789867903047,24.8450751394032,152.362354114282));
#94254=CARTESIAN_POINT('Ctrl Pts',(-177.791765513594,24.8464564548674,152.367933553429));
#94255=CARTESIAN_POINT('Ctrl Pts',(-177.799045366706,24.8517556316108,152.38933810216));
#94256=CARTESIAN_POINT('Ctrl Pts',(-177.804942413803,24.8564054048408,152.41117000322));
#94257=CARTESIAN_POINT('Ctrl Pts',(-177.809351695265,24.8603379619669,152.433309469188));
#94258=CARTESIAN_POINT('Ctrl Pts',(-177.813741723205,24.8642533472315,152.455352261202));
#94259=CARTESIAN_POINT('Ctrl Pts',(-177.816656889232,24.8674576873292,152.477699726678));
#94260=CARTESIAN_POINT('Ctrl Pts',(-177.818039597892,24.8699057546573,152.500225529015));
#94261=CARTESIAN_POINT('Ctrl Pts',(-177.819419519771,24.8723488880258,152.522705931702));
#94262=CARTESIAN_POINT('Ctrl Pts',(-177.819273139007,24.8740387349888,152.545363729093));
#94263=CARTESIAN_POINT('Ctrl Pts',(-177.817589716999,24.8749530460444,152.568068511054));
#94264=CARTESIAN_POINT('Ctrl Pts',(-177.816597164382,24.8754921276451,152.581455344921));
#94265=CARTESIAN_POINT('Ctrl Pts',(-177.815071168718,24.8757620423259,152.59485843705));
#94266=CARTESIAN_POINT('Ctrl Pts',(-177.813017113379,24.8757620423259,152.608250755187));
#94267=CARTESIAN_POINT('Ctrl Pts',(-178.535788240059,25.1869009068823,152.663678496546));
#94268=CARTESIAN_POINT('Ctrl Pts',(-178.547796223577,25.1859432627129,152.495194134801));
#94269=CARTESIAN_POINT('Ctrl Pts',(-178.538609818861,25.163582676433,152.329284557108));
#94270=CARTESIAN_POINT('Ctrl Pts',(-178.479567260233,25.0795971521013,152.008723248302));
#94271=CARTESIAN_POINT('Ctrl Pts',(-178.431254315525,25.0200759880067,151.860897232914));
#94272=CARTESIAN_POINT('Ctrl Pts',(-178.302546191152,24.8727975366848,151.586410602999));
#94273=CARTESIAN_POINT('Ctrl Pts',(-178.225101795571,24.7884206874165,151.465908921215));
#94274=CARTESIAN_POINT('Ctrl Pts',(-178.049596269999,24.604137587983,151.250262654017));
#94275=CARTESIAN_POINT('Ctrl Pts',(-177.951438762234,24.5042156002709,151.15576939922));
#94276=CARTESIAN_POINT('Ctrl Pts',(-177.641856056835,24.1974334944718,150.913299742263));
#94277=CARTESIAN_POINT('Ctrl Pts',(-177.409356901872,23.9777223770421,150.800741214681));
#94278=CARTESIAN_POINT('Ctrl Pts',(-176.932746614676,23.5448805316748,150.655018674087));
#94279=CARTESIAN_POINT('Ctrl Pts',(-176.685562735176,23.3285973273397,150.61976374185));
#94280=CARTESIAN_POINT('Ctrl Pts',(-176.430593086108,23.1126512166033,150.616656461907));
#94281=CARTESIAN_POINT('Ctrl Pts',(1.55202975899355E-14,24.8757620423259,
194.999549694134));
#94282=CARTESIAN_POINT('Ctrl Pts',(1.58565405550443E-14,24.8757620423259,
195.993992404177));
#94283=CARTESIAN_POINT('Ctrl Pts',(1.58584143467919E-14,25.8701893108725,
195.999534166346));
#94284=CARTESIAN_POINT('Ctrl Pts',(8.03327402494744,24.8757620423259,194.999549693465));
#94285=CARTESIAN_POINT('Ctrl Pts',(8.03265114999351,24.8757620423259,195.993992403173));
#94286=CARTESIAN_POINT('Ctrl Pts',(8.0326478760129,25.870189310896,195.999534166346));
#94287=CARTESIAN_POINT('Ctrl Pts',(16.0665519263718,24.8757620423259,195.007625218402));
#94288=CARTESIAN_POINT('Ctrl Pts',(16.05956801298,24.8757620423259,196.002365960777));
#94289=CARTESIAN_POINT('Ctrl Pts',(16.0655869046176,25.8704939364008,196.007612037979));
#94290=CARTESIAN_POINT('Ctrl Pts',(32.1331056843908,24.8757620423259,195.019685540921));
#94291=CARTESIAN_POINT('Ctrl Pts',(32.1265589240983,24.8757620423259,196.011429209992));
#94292=CARTESIAN_POINT('Ctrl Pts',(32.1325694456472,25.8674762936769,196.019652230615));
#94293=CARTESIAN_POINT('Ctrl Pts',(40.1663819277293,24.8757620423259,195.02433275779));
#94294=CARTESIAN_POINT('Ctrl Pts',(40.1403350532895,24.8757620423259,196.012908330767));
#94295=CARTESIAN_POINT('Ctrl Pts',(40.166583673479,25.8642139458239,196.024289902376));
#94296=CARTESIAN_POINT('Ctrl Pts',(56.2329144880606,24.8757620423259,194.990277721149));
#94297=CARTESIAN_POINT('Ctrl Pts',(56.2107775732178,24.8757620423259,195.965813387242));
#94298=CARTESIAN_POINT('Ctrl Pts',(56.2369512836255,25.8509477599953,195.989985501537));
#94299=CARTESIAN_POINT('Ctrl Pts',(64.2664422769928,24.8757620423259,194.952999205055));
#94300=CARTESIAN_POINT('Ctrl Pts',(64.2154476695745,24.8757620423259,195.919527238438));
#94301=CARTESIAN_POINT('Ctrl Pts',(64.2735317794456,25.8409667594794,195.952498173634));
#94302=CARTESIAN_POINT('Ctrl Pts',(76.314252180968,24.8757620423259,194.798403354012));
#94303=CARTESIAN_POINT('Ctrl Pts',(76.3147727001544,24.8757620423259,195.742698385788));
#94304=CARTESIAN_POINT('Ctrl Pts',(76.3299297419014,25.8184315808282,195.796667959559));
#94305=CARTESIAN_POINT('Ctrl Pts',(80.3298095531146,24.8757620423259,194.729928811641));
#94306=CARTESIAN_POINT('Ctrl Pts',(80.3286011897685,24.8757620423259,195.666169004327));
#94307=CARTESIAN_POINT('Ctrl Pts',(80.3490350159167,25.8096555448394,195.727620035734));
#94308=CARTESIAN_POINT('Ctrl Pts',(88.3596963527688,24.8757620423259,194.538124415895));
#94309=CARTESIAN_POINT('Ctrl Pts',(88.3667666841118,24.8757620423259,195.455007000289));
#94310=CARTESIAN_POINT('Ctrl Pts',(88.3880903624907,25.7890987455482,195.534021357848));
#94311=CARTESIAN_POINT('Ctrl Pts',(92.3740336964655,24.8757620423259,194.41496224834));
#94312=CARTESIAN_POINT('Ctrl Pts',(92.3804567159732,24.8757620423259,195.321439749224));
#94313=CARTESIAN_POINT('Ctrl Pts',(92.4080506792306,25.7773172405769,195.40964281312));
#94314=CARTESIAN_POINT('Ctrl Pts',(96.3873930174844,24.8757620423259,194.248481295077));
#94315=CARTESIAN_POINT('Ctrl Pts',(96.4244308304192,24.8757620423259,195.141352513976));
#94316=CARTESIAN_POINT('Ctrl Pts',(96.4285783862348,25.7637803812362,195.241337716207));
#94317=CARTESIAN_POINT('Ctrl Pts',(95.8129090247637,24.8757620423259,194.272017475705));
#94318=CARTESIAN_POINT('Ctrl Pts',(91.9909515239712,24.8757620423259,194.42665335126));
#94319=CARTESIAN_POINT('Ctrl Pts',(88.1681288624907,24.8757620425647,194.542724031316));
#94320=CARTESIAN_POINT('Ctrl Pts',(84.3447532974164,24.8757620424299,194.634041035195));
#94321=CARTESIAN_POINT('Ctrl Pts',(84.1771313987723,24.875762042424,194.638044494785));
#94322=CARTESIAN_POINT('Ctrl Pts',(84.0095084240956,24.8757620424174,194.64200008328));
#94323=CARTESIAN_POINT('Ctrl Pts',(83.8418843898354,24.8757620424104,194.645908558742));
#94324=CARTESIAN_POINT('Ctrl Pts',(79.9945138556477,24.8757620422484,194.735617372831));
#94325=CARTESIAN_POINT('Ctrl Pts',(76.1465874264899,24.8757620434871,194.800604548745));
#94326=CARTESIAN_POINT('Ctrl Pts',(72.2983160265908,24.8757620430265,194.849972733157));
#94327=CARTESIAN_POINT('Ctrl Pts',(72.1546046067635,24.8757620430093,194.851816358811));
#94328=CARTESIAN_POINT('Ctrl Pts',(72.0108926622784,24.8757620429891,194.853638836942));
#94329=CARTESIAN_POINT('Ctrl Pts',(71.8671802044666,24.8757620429662,194.855440421815));
#94330=CARTESIAN_POINT('Ctrl Pts',(63.9789651784272,24.8757620417107,194.954327387389));
#94331=CARTESIAN_POINT('Ctrl Pts',(56.0891782843935,24.8757620427095,194.990613753671));
#94332=CARTESIAN_POINT('Ctrl Pts',(48.1996482431872,24.8757620424645,195.007321889678));
#94333=CARTESIAN_POINT('Ctrl Pts',(48.1038239921383,24.8757620424615,195.007524822503));
#94334=CARTESIAN_POINT('Ctrl Pts',(48.0079997403916,24.8757620424585,195.007724664509));
#94335=CARTESIAN_POINT('Ctrl Pts',(47.912175487993,24.8757620424554,195.007921449932));
#94336=CARTESIAN_POINT('Ctrl Pts',(39.9747332096749,24.8757620421988,195.024221842576));
#94337=CARTESIAN_POINT('Ctrl Pts',(32.0372813112697,24.8757620423402,195.019619730156));
#94338=CARTESIAN_POINT('Ctrl Pts',(24.0998288030149,24.8757620423309,195.013658532168));
#94339=CARTESIAN_POINT('Ctrl Pts',(24.0519166148576,24.8757620423308,195.013622549081));
#94340=CARTESIAN_POINT('Ctrl Pts',(24.0040044266648,24.8757620423307,195.013586492909));
#94341=CARTESIAN_POINT('Ctrl Pts',(23.9560922384375,24.8757620423307,195.013550365792));
#94342=CARTESIAN_POINT('Ctrl Pts',(15.9707275303564,24.8757620423211,195.007529179632));
#94343=CARTESIAN_POINT('Ctrl Pts',(7.98536193554124,24.8757620423259,194.999549694134));
#94344=CARTESIAN_POINT('Ctrl Pts',(1.55202975899355E-14,24.8757620423259,
194.999549694134));
#94345=CARTESIAN_POINT('Ctrl Pts',(1.58047048864619E-14,25.8701893108725,
195.999534166346));
#94346=CARTESIAN_POINT('Ctrl Pts',(7.9786085072197,25.8701893108725,195.999534166346));
#94347=CARTESIAN_POINT('Ctrl Pts',(15.9572208444829,25.8704907335884,196.007496139866));
#94348=CARTESIAN_POINT('Ctrl Pts',(31.9144423244155,25.8675403396453,196.019522756113));
#94349=CARTESIAN_POINT('Ctrl Pts',(39.8930517912443,25.8643466712877,196.024234148174));
#94350=CARTESIAN_POINT('Ctrl Pts',(55.8502484700875,25.8513562852167,195.991424613018));
#94351=CARTESIAN_POINT('Ctrl Pts',(63.8291245674269,25.8415812736672,195.955278690271));
#94352=CARTESIAN_POINT('Ctrl Pts',(75.7949891858004,25.8195295821858,195.804927091771));
#94353=CARTESIAN_POINT('Ctrl Pts',(79.7832351076495,25.8109441238302,195.738304913061));
#94354=CARTESIAN_POINT('Ctrl Pts',(87.7585153676325,25.7908447875607,195.55171229018));
#94355=CARTESIAN_POINT('Ctrl Pts',(91.7455532525854,25.779330193458,195.431898989199));
#94356=CARTESIAN_POINT('Ctrl Pts',(95.731638354173,25.7661094150367,195.270070553806));
#94357=CARTESIAN_POINT('Ctrl Pts',(-175.118478031602,23.3269112215416,151.608250755187));
#94358=CARTESIAN_POINT('Ctrl Pts',(-175.744203657372,22.5468679911663,151.608250755187));
#94359=CARTESIAN_POINT('Ctrl Pts',(-175.744203657372,22.5468679911663,150.608250755187));
#94360=CARTESIAN_POINT('Ctrl Pts',(-175.343333626061,23.5072831574842,151.608250755187));
#94361=CARTESIAN_POINT('Ctrl Pts',(-175.973848539976,22.7347343216712,151.608250755187));
#94362=CARTESIAN_POINT('Ctrl Pts',(-175.975961504203,22.7327766922334,150.611103991362));
#94363=CARTESIAN_POINT('Ctrl Pts',(-175.565295636808,23.6902382307512,151.608250755187));
#94364=CARTESIAN_POINT('Ctrl Pts',(-176.200866106771,22.9254561683507,151.608250755183));
#94365=CARTESIAN_POINT('Ctrl Pts',(-176.20475353061,22.9213767890848,150.613904186401));
#94366=CARTESIAN_POINT('Ctrl Pts',(-175.784380109018,23.8757620423259,151.608250755187));
#94367=CARTESIAN_POINT('Ctrl Pts',(-176.425206487511,23.1190122335564,151.608250755187));
#94368=CARTESIAN_POINT('Ctrl Pts',(-176.430593086108,23.1126512166033,150.616656461907));
#94369=CARTESIAN_POINT('',(-175.744203657372,22.5468679911664,150.608250755186));
#94370=CARTESIAN_POINT('',(-175.118478031602,23.3269112215416,151.608250755187));
#94371=CARTESIAN_POINT('Origin',(-175.118478031602,23.3269112215417,150.608250755187));
#94372=CARTESIAN_POINT('Origin',(-154.804630390602,48.6513968890273,151.608250754885));
#94373=CARTESIAN_POINT('Origin',(-154.870164447103,48.5744178866766,150.300300299738));
#94374=CARTESIAN_POINT('Ctrl Pts',(177.813017113378,24.8757620423259,152.608250755187));
#94375=CARTESIAN_POINT('Ctrl Pts',(178.240980734254,24.8757620423259,152.641070351893));
#94376=CARTESIAN_POINT('Ctrl Pts',(178.535788240059,25.1869009068823,152.663678496546));
#94377=CARTESIAN_POINT('Ctrl Pts',(177.825566679641,24.8757620423259,152.526428293251));
#94378=CARTESIAN_POINT('Ctrl Pts',(178.251679320414,24.8784434436938,152.524853998483));
#94379=CARTESIAN_POINT('Ctrl Pts',(178.54758409262,25.1859601727659,152.498170456853));
#94380=CARTESIAN_POINT('Ctrl Pts',(177.818423466009,24.865861047641,152.446309988772));
#94381=CARTESIAN_POINT('Ctrl Pts',(178.244029236806,24.8627191690581,152.410014683625));
#94382=CARTESIAN_POINT('Ctrl Pts',(178.539112920021,25.1646159030061,152.335970744568));
#94383=CARTESIAN_POINT('Ctrl Pts',(177.765101637553,24.8270475515925,152.289539707351));
#94384=CARTESIAN_POINT('Ctrl Pts',(178.192522347297,24.7961838564161,152.188597127195));
#94385=CARTESIAN_POINT('Ctrl Pts',(178.48199168857,25.0827439046829,152.018126940536));
#94386=CARTESIAN_POINT('Ctrl Pts',(177.720007588841,24.7989783444832,152.216559013661));
#94387=CARTESIAN_POINT('Ctrl Pts',(178.149396328714,24.7464442378946,152.086521065475));
#94388=CARTESIAN_POINT('Ctrl Pts',(178.434507805055,25.0239982148635,151.86995404495));
#94389=CARTESIAN_POINT('Ctrl Pts',(177.599043397733,24.7293534239432,152.081816985205));
#94390=CARTESIAN_POINT('Ctrl Pts',(178.035536927632,24.6224967346167,151.903739043874));
#94391=CARTESIAN_POINT('Ctrl Pts',(178.307963263112,24.878810018743,151.595984391803));
#94392=CARTESIAN_POINT('Ctrl Pts',(177.524708125271,24.6886957305656,152.021807528286));
#94393=CARTESIAN_POINT('Ctrl Pts',(177.965629460751,24.5492727794077,151.82510958591));
#94394=CARTESIAN_POINT('Ctrl Pts',(178.230508883466,24.7942404010545,151.473748939335));
#94395=CARTESIAN_POINT('Ctrl Pts',(177.356757151249,24.6002878535161,151.915546497388));
#94396=CARTESIAN_POINT('Ctrl Pts',(177.809547956828,24.3904862015032,151.693026376618));
#94397=CARTESIAN_POINT('Ctrl Pts',(178.055904211603,24.6106280179359,151.256894473064));
#94398=CARTESIAN_POINT('Ctrl Pts',(177.261863754394,24.5518950929903,151.868742623834));
#94399=CARTESIAN_POINT('Ctrl Pts',(177.721535105475,24.3031663131539,151.639064057359));
#94400=CARTESIAN_POINT('Ctrl Pts',(177.957429169392,24.5102532970104,151.161143710607));
#94401=CARTESIAN_POINT('Ctrl Pts',(177.06248138814,24.452976281066,151.789195261869));
#94402=CARTESIAN_POINT('Ctrl Pts',(177.538716234914,24.1255898483891,151.556268560496));
#94403=CARTESIAN_POINT('Ctrl Pts',(177.750773427807,24.3052696647133,150.997960420331));
#94404=CARTESIAN_POINT('Ctrl Pts',(176.957127456991,24.4019796098267,151.755840098305));
#94405=CARTESIAN_POINT('Ctrl Pts',(177.442509904882,24.0339937760569,151.526995608583));
#94406=CARTESIAN_POINT('Ctrl Pts',(177.641692710208,24.1996827677703,150.929280961348));
#94407=CARTESIAN_POINT('Ctrl Pts',(176.736712019782,24.2976666717929,151.699677511058));
#94408=CARTESIAN_POINT('Ctrl Pts',(177.243766764194,23.8479909141434,151.489142631931));
#94409=CARTESIAN_POINT('Ctrl Pts',(177.413666278864,23.9838543743893,150.813119343421));
#94410=CARTESIAN_POINT('Ctrl Pts',(176.621429091326,24.2442684005504,151.676957335305));
#94411=CARTESIAN_POINT('Ctrl Pts',(177.140590331384,23.7531010317192,151.481294705877));
#94412=CARTESIAN_POINT('Ctrl Pts',(177.294493508481,23.8734448220722,150.765810854267));
#94413=CARTESIAN_POINT('Ctrl Pts',(176.272211171489,24.0856625592316,151.624198290699));
#94414=CARTESIAN_POINT('Ctrl Pts',(176.827686158777,23.4694432056994,151.486934169814));
#94415=CARTESIAN_POINT('Ctrl Pts',(176.93371995992,23.5456907356619,150.654945935944));
#94416=CARTESIAN_POINT('Ctrl Pts',(176.031572249751,23.9804249323003,151.608250755187));
#94417=CARTESIAN_POINT('Ctrl Pts',(176.619316842118,23.2864267698944,151.532148617704));
#94418=CARTESIAN_POINT('Ctrl Pts',(176.685418012928,23.3284747550706,150.61976197741));
#94419=CARTESIAN_POINT('Ctrl Pts',(175.784380109018,23.8757620423259,151.608250755187));
#94420=CARTESIAN_POINT('Ctrl Pts',(176.425206487511,23.1190122335564,151.608250755187));
#94421=CARTESIAN_POINT('Ctrl Pts',(176.430593086108,23.1126512166033,150.616656461907));
#94422=CARTESIAN_POINT('',(177.813017113379,24.8757620423259,152.608250755187));
#94423=CARTESIAN_POINT('',(178.535788240059,25.1869009068823,152.663678496546));
#94424=CARTESIAN_POINT('Origin',(177.813017113378,25.8757620423259,152.608250755187));
#94425=CARTESIAN_POINT('',(175.784380109018,23.8757620423259,151.608250755187));
#94426=CARTESIAN_POINT('Ctrl Pts',(175.784380109018,23.8757620423259,151.608250755187));
#94427=CARTESIAN_POINT('Ctrl Pts',(175.888180218743,23.9197117384257,151.608250755187));
#94428=CARTESIAN_POINT('Ctrl Pts',(175.991532071282,23.9640615485664,151.611059044171));
#94429=CARTESIAN_POINT('Ctrl Pts',(176.094384782567,24.0088514257039,151.617055154659));
#94430=CARTESIAN_POINT('Ctrl Pts',(176.197237493852,24.0536413028414,151.623051265146));
#94431=CARTESIAN_POINT('Ctrl Pts',(176.299591232898,24.0988712414086,151.632234747727));
#94432=CARTESIAN_POINT('Ctrl Pts',(176.401375438295,24.1445818688343,151.645033982858));
#94433=CARTESIAN_POINT('Ctrl Pts',(176.436027334069,24.1601438107991,151.649391414937));
#94434=CARTESIAN_POINT('Ctrl Pts',(176.470564826423,24.1757406050875,151.654162192433));
#94435=CARTESIAN_POINT('Ctrl Pts',(176.505029440578,24.1913935197761,151.659368902388));
#94436=CARTESIAN_POINT('Ctrl Pts',(176.558262537659,24.2155705821821,151.667411043676));
#94437=CARTESIAN_POINT('Ctrl Pts',(176.611498776826,24.2399670802618,151.676560125858));
#94438=CARTESIAN_POINT('Ctrl Pts',(176.664512322343,24.2644906804516,151.686907893715));
#94439=CARTESIAN_POINT('Ctrl Pts',(176.712038321724,24.286475790032,151.696184541862));
#94440=CARTESIAN_POINT('Ctrl Pts',(176.759385912566,24.3085633732731,151.706424858618));
#94441=CARTESIAN_POINT('Ctrl Pts',(176.806356876171,24.3306751310717,151.717716698402));
#94442=CARTESIAN_POINT('Ctrl Pts',(176.81991182181,24.3370561727181,151.720975313143));
#94443=CARTESIAN_POINT('Ctrl Pts',(176.833435128408,24.3434391303508,151.72432163475));
#94444=CARTESIAN_POINT('Ctrl Pts',(176.846921303972,24.349821858476,151.727758114264));
#94445=CARTESIAN_POINT('Ctrl Pts',(176.895195965378,24.3726692578471,151.740059220992));
#94446=CARTESIAN_POINT('Ctrl Pts',(176.943039615744,24.3955301215035,151.753495797282));
#94447=CARTESIAN_POINT('Ctrl Pts',(176.990442789502,24.4184161773618,151.76827863874));
#94448=CARTESIAN_POINT('Ctrl Pts',(176.994268160631,24.4202630506911,151.769471593778));
#94449=CARTESIAN_POINT('Ctrl Pts',(176.998090645382,24.4221100825407,151.770673337412));
#94450=CARTESIAN_POINT('Ctrl Pts',(177.001910229157,24.4239572760715,151.771883991953));
#94451=CARTESIAN_POINT('Ctrl Pts',(177.0444989963,24.4445536812752,151.785382919412));
#94452=CARTESIAN_POINT('Ctrl Pts',(177.08665352189,24.4651324708619,151.79996132566));
#94453=CARTESIAN_POINT('Ctrl Pts',(177.12839171876,24.4857188059926,151.815813193461));
#94454=CARTESIAN_POINT('Ctrl Pts',(177.13968511927,24.491288996971,151.820102345973));
#94455=CARTESIAN_POINT('Ctrl Pts',(177.150947856937,24.4968596820121,151.824484949505));
#94456=CARTESIAN_POINT('Ctrl Pts',(177.162179864868,24.5024312232115,151.828965353137));
#94457=CARTESIAN_POINT('Ctrl Pts',(177.195487427009,24.5189531537376,151.84225160821));
#94458=CARTESIAN_POINT('Ctrl Pts',(177.228624808266,24.5355367352923,151.856465474584));
#94459=CARTESIAN_POINT('Ctrl Pts',(177.261374704995,24.5520821064625,151.871664050034));
#94460=CARTESIAN_POINT('Ctrl Pts',(177.26991614724,24.5563972752534,151.875627963431));
#94461=CARTESIAN_POINT('Ctrl Pts',(177.27843099085,24.560709735723,151.879658911046));
#94462=CARTESIAN_POINT('Ctrl Pts',(177.28691483948,24.5650174701844,151.883758017371));
#94463=CARTESIAN_POINT('Ctrl Pts',(177.314410277666,24.5789784744137,151.8970428754));
#94464=CARTESIAN_POINT('Ctrl Pts',(177.341592500569,24.5928993205188,151.911050511792));
#94465=CARTESIAN_POINT('Ctrl Pts',(177.368326940738,24.6067183609374,151.925844650535));
#94466=CARTESIAN_POINT('Ctrl Pts',(177.392890006516,24.6194150172597,151.93943720758));
#94467=CARTESIAN_POINT('Ctrl Pts',(177.417075156271,24.6320258038282,151.953693827921));
#94468=CARTESIAN_POINT('Ctrl Pts',(177.440743155166,24.6444877057936,151.968672101291));
#94469=CARTESIAN_POINT('Ctrl Pts',(177.465429074447,24.6574855729723,151.984294564731));
#94470=CARTESIAN_POINT('Ctrl Pts',(177.489662827417,24.6703770455339,152.00074916361));
#94471=CARTESIAN_POINT('Ctrl Pts',(177.513302330664,24.683097490483,152.018148254101));
#94472=CARTESIAN_POINT('Ctrl Pts',(177.525339790684,24.6895748621053,152.027008036558));
#94473=CARTESIAN_POINT('Ctrl Pts',(177.537222502338,24.6960075867644,152.036112982289));
#94474=CARTESIAN_POINT('Ctrl Pts',(177.548927160266,24.7023850415595,152.045479650782));
#94475=CARTESIAN_POINT('Ctrl Pts',(177.570211034337,24.7139818729737,152.062512100076));
#94476=CARTESIAN_POINT('Ctrl Pts',(177.590992424048,24.725444492759,152.080478691788));
#94477=CARTESIAN_POINT('Ctrl Pts',(177.611061345678,24.7366768879423,152.099491146059));
#94478=CARTESIAN_POINT('Ctrl Pts',(177.627758076354,24.7460218981362,152.115308928116));
#94479=CARTESIAN_POINT('Ctrl Pts',(177.643961093387,24.7552072817013,152.131850812328));
#94480=CARTESIAN_POINT('Ctrl Pts',(177.659525493287,24.7641658842132,152.149187999433));
#94481=CARTESIAN_POINT('Ctrl Pts',(177.677793426276,24.7746805941549,152.169536652404));
#94482=CARTESIAN_POINT('Ctrl Pts',(177.695042493007,24.7848015699428,152.190821330371));
#94483=CARTESIAN_POINT('Ctrl Pts',(177.711012304548,24.7943992985756,152.213126541485));
#94484=CARTESIAN_POINT('Ctrl Pts',(177.719375281163,24.7994253804369,152.224807202742));
#94485=CARTESIAN_POINT('Ctrl Pts',(177.727386726949,24.8043075848329,152.23676782866));
#94486=CARTESIAN_POINT('Ctrl Pts',(177.735004212646,24.809024585629,152.249021220301));
#94487=CARTESIAN_POINT('Ctrl Pts',(177.741978345054,24.8133432006452,152.260239721936));
#94488=CARTESIAN_POINT('Ctrl Pts',(177.748622222903,24.8175233231468,152.27170363004));
#94489=CARTESIAN_POINT('Ctrl Pts',(177.754900516826,24.8215470776803,152.283423111307));
#94490=CARTESIAN_POINT('Ctrl Pts',(177.758407711195,24.8237948362933,152.289969873725));
#94491=CARTESIAN_POINT('Ctrl Pts',(177.761805375059,24.8259967232679,152.29660500088));
#94492=CARTESIAN_POINT('Ctrl Pts',(177.765085505741,24.8281486580691,152.303329793373));
#94493=CARTESIAN_POINT('Ctrl Pts',(177.77517402172,24.8347672445639,152.324012864603));
#94494=CARTESIAN_POINT('Ctrl Pts',(177.784149435374,24.8409126354964,152.345541699617));
#94495=CARTESIAN_POINT('Ctrl Pts',(177.791762551781,24.8464542996167,152.367924848061));
#94496=CARTESIAN_POINT('Ctrl Pts',(177.799661503614,24.8522040262227,152.391148374666));
#94497=CARTESIAN_POINT('Ctrl Pts',(177.805997059918,24.8572289222201,152.414969007613));
#94498=CARTESIAN_POINT('Ctrl Pts',(177.810561932378,24.861415583222,152.439360104592));
#94499=CARTESIAN_POINT('Ctrl Pts',(177.814618969591,24.8651364844365,152.461037728438));
#94500=CARTESIAN_POINT('Ctrl Pts',(177.81722943523,24.8681523378528,152.482924377057));
#94501=CARTESIAN_POINT('Ctrl Pts',(177.818364411308,24.8704356907676,152.504933805796));
#94502=CARTESIAN_POINT('Ctrl Pts',(177.819498002199,24.8727162569556,152.526916373043));
#94503=CARTESIAN_POINT('Ctrl Pts',(177.819159697831,24.8742660736894,152.549021416549));
#94504=CARTESIAN_POINT('Ctrl Pts',(177.817367217729,24.8750808954348,152.571158938715));
#94505=CARTESIAN_POINT('Ctrl Pts',(177.816366483363,24.8755358071082,152.583518227493));
#94506=CARTESIAN_POINT('Ctrl Pts',(177.814913325236,24.8757620423259,152.59588756713));
#94507=CARTESIAN_POINT('Ctrl Pts',(177.813017113379,24.8757620423259,152.608250755187));
#94508=CARTESIAN_POINT('',(176.430596903941,23.1126467080106,150.616656511736));
#94509=CARTESIAN_POINT('Origin',(175.784380109018,23.8757620423259,150.608250755187));
#94510=CARTESIAN_POINT('Ctrl Pts',(176.430593086108,23.1126512166033,150.616656461907));
#94511=CARTESIAN_POINT('Ctrl Pts',(176.620942243517,23.273867111808,150.618976220831));
#94512=CARTESIAN_POINT('Ctrl Pts',(176.807287751197,23.4355523540411,150.639197828199));
#94513=CARTESIAN_POINT('Ctrl Pts',(176.989159692478,23.5976629315714,150.679854720897));
#94514=CARTESIAN_POINT('Ctrl Pts',(177.050901364054,23.6526960387475,150.693656874756));
#94515=CARTESIAN_POINT('Ctrl Pts',(177.11212758244,23.707778192619,150.709813675416));
#94516=CARTESIAN_POINT('Ctrl Pts',(177.172820282514,23.7629077585044,150.728422933407));
#94517=CARTESIAN_POINT('Ctrl Pts',(177.173292023554,23.7633362594394,150.728567576019));
#94518=CARTESIAN_POINT('Ctrl Pts',(177.173763731008,23.7637647620101,150.728712366428));
#94519=CARTESIAN_POINT('Ctrl Pts',(177.174235404887,23.7641932662315,150.728857304682));
#94520=CARTESIAN_POINT('Ctrl Pts',(177.259960857398,23.8420727502167,150.755199440557));
#94521=CARTESIAN_POINT('Ctrl Pts',(177.345014579002,23.9204305734928,150.786762479351));
#94522=CARTESIAN_POINT('Ctrl Pts',(177.428034382514,23.998042726141,150.8237109945));
#94523=CARTESIAN_POINT('Ctrl Pts',(177.460499505064,24.028393171944,150.838159812994));
#94524=CARTESIAN_POINT('Ctrl Pts',(177.492653610754,24.0586297153941,150.85343273917));
#94525=CARTESIAN_POINT('Ctrl Pts',(177.524414819681,24.0886792232459,150.869541775791));
#94526=CARTESIAN_POINT('Ctrl Pts',(177.525503416018,24.0897091520578,150.870093903334));
#94527=CARTESIAN_POINT('Ctrl Pts',(177.526591550734,24.0907388611171,150.870647013372));
#94528=CARTESIAN_POINT('Ctrl Pts',(177.527679220282,24.0917683472481,150.871201106284));
#94529=CARTESIAN_POINT('Ctrl Pts',(177.639922830175,24.1980076365004,150.928381514429));
#94530=CARTESIAN_POINT('Ctrl Pts',(177.747432873769,24.3020358637303,150.995859328735));
#94531=CARTESIAN_POINT('Ctrl Pts',(177.849416010482,24.403116055102,151.075868335985));
#94532=CARTESIAN_POINT('Ctrl Pts',(177.850978666586,24.4046648756532,151.07709428929));
#94533=CARTESIAN_POINT('Ctrl Pts',(177.852540009189,24.4062129884345,151.078323175045));
#94534=CARTESIAN_POINT('Ctrl Pts',(177.854100036342,24.4077603916609,151.079555001813));
#94535=CARTESIAN_POINT('Ctrl Pts',(177.916984382241,24.4701358698746,151.129209663512));
#94536=CARTESIAN_POINT('Ctrl Pts',(177.978066376459,24.5317217937356,151.184101986091));
#94537=CARTESIAN_POINT('Ctrl Pts',(178.035969220689,24.591114122828,151.24395542159));
#94538=CARTESIAN_POINT('Ctrl Pts',(178.073149186829,24.6292505013424,151.282387880907));
#94539=CARTESIAN_POINT('Ctrl Pts',(178.10901808617,24.6664823060443,151.322866578078));
#94540=CARTESIAN_POINT('Ctrl Pts',(178.14320414749,24.7024320267223,151.365325418936));
#94541=CARTESIAN_POINT('Ctrl Pts',(178.189881763411,24.7515177414698,151.423298680247));
#94542=CARTESIAN_POINT('Ctrl Pts',(178.233801900382,24.7985951004967,151.485285816535));
#94543=CARTESIAN_POINT('Ctrl Pts',(178.274300365435,24.8429464492918,151.551510019952));
#94544=CARTESIAN_POINT('Ctrl Pts',(178.307825929647,24.8796615196029,151.606331944218));
#94545=CARTESIAN_POINT('Ctrl Pts',(178.339006378201,24.9145082772951,151.664057880399));
#94546=CARTESIAN_POINT('Ctrl Pts',(178.367447537254,24.9470634889582,151.724827914402));
#94547=CARTESIAN_POINT('Ctrl Pts',(178.368715166528,24.9485144825435,151.72753644938));
#94548=CARTESIAN_POINT('Ctrl Pts',(178.369977231717,24.9499607849485,151.730250787971));
#94549=CARTESIAN_POINT('Ctrl Pts',(178.371233703054,24.9514023638144,151.732970946095));
#94550=CARTESIAN_POINT('Ctrl Pts',(178.397594887464,24.9816471654459,151.790040763632));
#94551=CARTESIAN_POINT('Ctrl Pts',(178.421217785221,25.0094902291248,151.849052198428));
#94552=CARTESIAN_POINT('Ctrl Pts',(178.441897120666,25.0346736294332,151.910064285732));
#94553=CARTESIAN_POINT('Ctrl Pts',(178.461639263896,25.0587157122757,151.968311291274));
#94554=CARTESIAN_POINT('Ctrl Pts',(178.478698736833,25.0803339837904,152.02838190416));
#94555=CARTESIAN_POINT('Ctrl Pts',(178.492865080253,25.0992740523429,152.09034605596));
#94556=CARTESIAN_POINT('Ctrl Pts',(178.498894652275,25.1073354485726,152.116719644752));
#94557=CARTESIAN_POINT('Ctrl Pts',(178.504399693808,25.1149112646649,152.143436484153));
#94558=CARTESIAN_POINT('Ctrl Pts',(178.509362013848,25.1219799614452,152.170502939887));
#94559=CARTESIAN_POINT('Ctrl Pts',(178.50976172314,25.1225493370133,152.172683112426));
#94560=CARTESIAN_POINT('Ctrl Pts',(178.510157869719,25.1231153641414,152.174865339501));
#94561=CARTESIAN_POINT('Ctrl Pts',(178.510550445545,25.1236780327978,152.177049621895));
#94562=CARTESIAN_POINT('Ctrl Pts',(178.524799466834,25.1441007820793,152.256330831494));
#94563=CARTESIAN_POINT('Ctrl Pts',(178.53405773826,25.1596591700609,152.336459756157));
#94564=CARTESIAN_POINT('Ctrl Pts',(178.53828485658,25.170241131487,152.41753159637));
#94565=CARTESIAN_POINT('Ctrl Pts',(178.542284907349,25.1802546630996,152.494248511332));
#94566=CARTESIAN_POINT('Ctrl Pts',(178.54177950378,25.1858118327628,152.571809812277));
#94567=CARTESIAN_POINT('Ctrl Pts',(178.536697911727,25.186780381516,152.650302317055));
#94568=CARTESIAN_POINT('Ctrl Pts',(178.536409449221,25.1868353623168,152.654758035734));
#94569=CARTESIAN_POINT('Ctrl Pts',(178.536106230804,25.1868755467193,152.659216756742));
#94570=CARTESIAN_POINT('Ctrl Pts',(178.535788240059,25.1869009068823,152.663678496546));
#94571=CARTESIAN_POINT('Ctrl Pts',(7.58040827681699E-15,-2.96262874552467,
151.608250755187));
#94572=CARTESIAN_POINT('Ctrl Pts',(7.71069817591099E-15,-3.96262874552467,
151.608250755187));
#94573=CARTESIAN_POINT('Ctrl Pts',(7.71069817591099E-15,-3.96262874552467,
150.608250755187));
#94574=CARTESIAN_POINT('Ctrl Pts',(-7.48001477234627,-2.96262874562523,
151.608250755187));
#94575=CARTESIAN_POINT('Ctrl Pts',(-7.47915914848108,-3.96262874562523,
151.608250755187));
#94576=CARTESIAN_POINT('Ctrl Pts',(-7.47915914848117,-3.96262874552467,
150.608250755187));
#94577=CARTESIAN_POINT('Ctrl Pts',(-14.9601902827936,-2.9704066144946,151.608250755187));
#94578=CARTESIAN_POINT('Ctrl Pts',(-14.9611695836601,-3.97041247107443,
151.608250755187));
#94579=CARTESIAN_POINT('Ctrl Pts',(-14.96116958366,-3.97041247104644,150.608250755187));
#94580=CARTESIAN_POINT('Ctrl Pts',(-29.9184179910251,-2.90250945369316,
151.608250755187));
#94581=CARTESIAN_POINT('Ctrl Pts',(-29.9265168326519,-3.90248299383942,
151.608250755187));
#94582=CARTESIAN_POINT('Ctrl Pts',(-29.926516832652,-3.90248299386741,150.608250755187));
#94583=CARTESIAN_POINT('Ctrl Pts',(-37.3964862791675,-2.82824484200836,
151.608250755187));
#94584=CARTESIAN_POINT('Ctrl Pts',(-37.4098860289911,-3.82817884079897,
151.608250755083));
#94585=CARTESIAN_POINT('Ctrl Pts',(-37.4098860290166,-3.82817884077274,
150.608250755083));
#94586=CARTESIAN_POINT('Ctrl Pts',(-52.3486036457515,-2.52473868654688,
151.608250755187));
#94587=CARTESIAN_POINT('Ctrl Pts',(-52.3757926152852,-3.52439278430538,
151.60825075529));
#94588=CARTESIAN_POINT('Ctrl Pts',(-52.3757926152598,-3.52439278433161,
150.60825075529));
#94589=CARTESIAN_POINT('Ctrl Pts',(-59.8226717303696,-2.29623000265189,
151.608250755187));
#94590=CARTESIAN_POINT('Ctrl Pts',(-59.8583568649177,-3.29564767497403,
151.60825075529));
#94591=CARTESIAN_POINT('Ctrl Pts',(-59.8583568649164,-3.29564767494582,
150.60825075529));
#94592=CARTESIAN_POINT('Ctrl Pts',(-71.0292449211431,-1.77883547863047,
151.608250755187));
#94593=CARTESIAN_POINT('Ctrl Pts',(-71.0805819281094,-2.7775305221053,151.608250755135));
#94594=CARTESIAN_POINT('Ctrl Pts',(-71.0805819281101,-2.77753052211941,
150.608250755135));
#94595=CARTESIAN_POINT('Ctrl Pts',(-74.7640118647851,-1.57716395400885,
151.608250755187));
#94596=CARTESIAN_POINT('Ctrl Pts',(-74.8210574168792,-2.57555542360394,
151.608250755135));
#94597=CARTESIAN_POINT('Ctrl Pts',(-74.821057416878,-2.57555542358512,150.608250755135));
#94598=CARTESIAN_POINT('Ctrl Pts',(-82.2317153529343,-1.10324244350201,
151.608250755187));
#94599=CARTESIAN_POINT('Ctrl Pts',(-82.3013406088045,-2.10083556964149,
151.608250755239));
#94600=CARTESIAN_POINT('Ctrl Pts',(-82.3013406088056,-2.10083556966032,
150.608250755239));
#94601=CARTESIAN_POINT('Ctrl Pts',(-85.9661068731236,-0.830903349436501,
151.608250755187));
#94602=CARTESIAN_POINT('Ctrl Pts',(-86.0426053104115,-1.82800207668471,
151.608250755135));
#94603=CARTESIAN_POINT('Ctrl Pts',(-86.04260531041,-1.8280020766666,150.608250755135));
#94604=CARTESIAN_POINT('Ctrl Pts',(-97.1555011499729,0.113239291570469,
151.608250755187));
#94605=CARTESIAN_POINT('Ctrl Pts',(-97.2547429890782,-0.881940384928872,
151.60825075529));
#94606=CARTESIAN_POINT('Ctrl Pts',(-97.2547429890811,-0.881940384965111,
150.60825075529));
#94607=CARTESIAN_POINT('Ctrl Pts',(-104.589500516371,0.908590385417737,
151.608250755187));
#94608=CARTESIAN_POINT('Ctrl Pts',(-104.706623983818,-0.0847860000410842,
151.608250755187));
#94609=CARTESIAN_POINT('Ctrl Pts',(-104.70662398386,-0.0847859999660353,
150.608250755187));
#94610=CARTESIAN_POINT('Ctrl Pts',(-115.6832946476,2.47242844681118,151.608250755187));
#94611=CARTESIAN_POINT('Ctrl Pts',(-115.834110543524,1.48380151869801,151.608250755187));
#94612=CARTESIAN_POINT('Ctrl Pts',(-115.834110543502,1.48380151866048,150.608250755187));
#94613=CARTESIAN_POINT('Ctrl Pts',(-119.371604706226,3.0560747245114,151.608250755187));
#94614=CARTESIAN_POINT('Ctrl Pts',(-119.534815140111,2.06938108833564,151.608250755031));
#94615=CARTESIAN_POINT('Ctrl Pts',(-119.534815140076,2.06938108832628,150.608250755083));
#94616=CARTESIAN_POINT('Ctrl Pts',(-126.724082256959,4.37986325499499,151.608250755187));
#94617=CARTESIAN_POINT('Ctrl Pts',(-126.915266651803,3.39820623507059,151.608250755342));
#94618=CARTESIAN_POINT('Ctrl Pts',(-126.915266651838,3.39820623507995,150.60825075529));
#94619=CARTESIAN_POINT('Ctrl Pts',(-130.3882896118,5.11974710981558,151.608250755187));
#94620=CARTESIAN_POINT('Ctrl Pts',(-130.595044169067,4.14118311580342,151.608250755135));
#94621=CARTESIAN_POINT('Ctrl Pts',(-130.595044169049,4.14118311588002,150.608250755135));
#94622=CARTESIAN_POINT('Ctrl Pts',(-135.861220457415,6.38112699928991,151.608250755187));
#94623=CARTESIAN_POINT('Ctrl Pts',(-136.094725659691,5.4087283902617,151.608250755213));
#94624=CARTESIAN_POINT('Ctrl Pts',(-136.0947256597,5.4087283902234,150.608250755213));
#94625=CARTESIAN_POINT('Ctrl Pts',(-137.681613722953,6.82697768764861,151.608250755187));
#94626=CARTESIAN_POINT('Ctrl Pts',(-137.924606380511,5.85689247239123,151.608250755161));
#94627=CARTESIAN_POINT('Ctrl Pts',(-137.924606380501,5.85689247242799,150.608250755161));
#94628=CARTESIAN_POINT('Ctrl Pts',(-141.313341356547,7.77740028733485,151.608250755187));
#94629=CARTESIAN_POINT('Ctrl Pts',(-141.576696462501,6.81264392189733,151.608250755213));
#94630=CARTESIAN_POINT('Ctrl Pts',(-141.576696462511,6.81264392186057,150.608250755213));
#94631=CARTESIAN_POINT('Ctrl Pts',(-143.1189853136,8.28050120342763,151.608250755187));
#94632=CARTESIAN_POINT('Ctrl Pts',(-143.39318392604,7.31875148009332,151.608250755135));
#94633=CARTESIAN_POINT('Ctrl Pts',(-143.393183926052,7.31875148011453,150.608250755161));
#94634=CARTESIAN_POINT('Ctrl Pts',(-148.49688844256,9.88460944395078,151.608250755187));
#94635=CARTESIAN_POINT('Ctrl Pts',(-148.805991124598,8.93327082393873,151.60825075529));
#94636=CARTESIAN_POINT('Ctrl Pts',(-148.805991124574,8.93327082389632,150.608250755239));
#94637=CARTESIAN_POINT('Ctrl Pts',(-152.032276636241,11.0793251114952,151.608250755187));
#94638=CARTESIAN_POINT('Ctrl Pts',(-152.367777204989,10.1366936288938,151.608250755031));
#94639=CARTESIAN_POINT('Ctrl Pts',(-152.367777204931,10.1366936289926,150.608250755083));
#94640=CARTESIAN_POINT('Ctrl Pts',(-158.966663136563,13.8113957628694,151.608250755187));
#94641=CARTESIAN_POINT('Ctrl Pts',(-159.364291195684,12.8932418158741,151.608250755342));
#94642=CARTESIAN_POINT('Ctrl Pts',(-159.364291195742,12.8932418157753,150.60825075529));
#94643=CARTESIAN_POINT('Ctrl Pts',(-162.366411372621,15.3468667695571,151.608250755187));
#94644=CARTESIAN_POINT('Ctrl Pts',(-162.799768640706,14.4443390394639,151.60825075503));
#94645=CARTESIAN_POINT('Ctrl Pts',(-162.799768640555,14.4443390396976,150.608250755083));
#94646=CARTESIAN_POINT('Ctrl Pts',(-166.491318743796,17.5796732143735,151.608250755187));
#94647=CARTESIAN_POINT('Ctrl Pts',(-166.97802048339,16.7060207701578,151.608250755226));
#94648=CARTESIAN_POINT('Ctrl Pts',(-166.978020483428,16.7060207700994,150.608250755213));
#94649=CARTESIAN_POINT('Ctrl Pts',(-167.309955007446,18.0421749712842,151.608250755187));
#94650=CARTESIAN_POINT('Ctrl Pts',(-167.807762984048,17.1747832534819,151.608250755173));
#94651=CARTESIAN_POINT('Ctrl Pts',(-167.807762983994,17.1747832535731,150.608250755173));
#94652=CARTESIAN_POINT('Ctrl Pts',(-168.93299683872,19.0029289063352,151.608250755187));
#94653=CARTESIAN_POINT('Ctrl Pts',(-169.453970557405,18.1492500685391,151.6082507552));
#94654=CARTESIAN_POINT('Ctrl Pts',(-169.453970557459,18.1492500684478,150.6082507552));
#94655=CARTESIAN_POINT('Ctrl Pts',(-169.737204958192,19.5011635886747,151.608250755187));
#94656=CARTESIAN_POINT('Ctrl Pts',(-170.270238326363,18.6549382700629,151.608250755187));
#94657=CARTESIAN_POINT('Ctrl Pts',(-170.27023832632,18.6549382701294,150.608250755187));
#94658=CARTESIAN_POINT('Ctrl Pts',(-172.109848566929,21.0455107820461,151.608250755187));
#94659=CARTESIAN_POINT('Ctrl Pts',(-172.680332460927,20.22366190761,151.608250755187));
#94660=CARTESIAN_POINT('Ctrl Pts',(-172.680332461013,20.2236619074771,150.608250755187));
#94661=CARTESIAN_POINT('Ctrl Pts',(-173.643681898189,22.1438771319804,151.608250755187));
#94662=CARTESIAN_POINT('Ctrl Pts',(-174.24092113324,21.3409830339438,151.608250755108));
#94663=CARTESIAN_POINT('Ctrl Pts',(-174.240921133641,21.3409830334629,150.608250755029));
#94664=CARTESIAN_POINT('Ctrl Pts',(-175.118478031529,23.3269112214833,151.608250755187));
#94665=CARTESIAN_POINT('Ctrl Pts',(-175.744203657298,22.5468679911069,151.608250755187));
#94666=CARTESIAN_POINT('Ctrl Pts',(-175.744203657298,22.5468679911069,150.608250755187));
#94667=CARTESIAN_POINT('',(7.71069817591099E-15,-3.96262874552467,150.608250755187));
#94668=CARTESIAN_POINT('',(7.59225281309826E-15,-2.96262874552467,151.608250755187));
#94669=CARTESIAN_POINT('Origin',(7.59225281309826E-15,-2.96262874552467,
150.608250755187));
#94670=CARTESIAN_POINT('Ctrl Pts',(-175.118478031529,23.3269112214833,151.608250755187));
#94671=CARTESIAN_POINT('Ctrl Pts',(-173.643670919279,22.1438683242896,151.608250755187));
#94672=CARTESIAN_POINT('Ctrl Pts',(-172.109848567067,21.0455107819602,151.608250755187));
#94673=CARTESIAN_POINT('Ctrl Pts',(-170.528086161207,20.0159459864725,151.608250755187));
#94674=CARTESIAN_POINT('Ctrl Pts',(-169.737204958277,19.5011635887287,151.608250755187));
#94675=CARTESIAN_POINT('Ctrl Pts',(-168.932996838842,19.0029289062917,151.608250755187));
#94676=CARTESIAN_POINT('Ctrl Pts',(-168.121475923185,18.5225519388115,151.608250755187));
#94677=CARTESIAN_POINT('Ctrl Pts',(-167.309955007528,18.0421749713315,151.608250755187));
#94678=CARTESIAN_POINT('Ctrl Pts',(-166.491318743916,17.5796732143511,151.608250755187));
#94679=CARTESIAN_POINT('Ctrl Pts',(-165.666337269668,17.133111925397,151.608250755187));
#94680=CARTESIAN_POINT('Ctrl Pts',(-162.366411372674,15.3468667695806,151.608250755187));
#94681=CARTESIAN_POINT('Ctrl Pts',(-158.966663136623,13.8113957627309,151.608250755187));
#94682=CARTESIAN_POINT('Ctrl Pts',(-155.499469886505,12.4453604371405,151.608250755187));
#94683=CARTESIAN_POINT('Ctrl Pts',(-152.032276636387,11.07932511155,151.608250755187));
#94684=CARTESIAN_POINT('Ctrl Pts',(-148.496888442587,9.8846094438595,151.608250755187));
#94685=CARTESIAN_POINT('Ctrl Pts',(-144.911619690001,8.81520395025918,151.608250755187));
#94686=CARTESIAN_POINT('Ctrl Pts',(-143.118985313708,8.28050120345901,151.608250755187));
#94687=CARTESIAN_POINT('Ctrl Pts',(-141.313341356563,7.77740028730139,151.608250755187));
#94688=CARTESIAN_POINT('Ctrl Pts',(-139.497477539825,7.30218898749211,151.608250755187));
#94689=CARTESIAN_POINT('Ctrl Pts',(-137.681613723086,6.82697768768278,151.608250755187));
#94690=CARTESIAN_POINT('Ctrl Pts',(-135.861220457474,6.38112699926441,151.608250755187));
#94691=CARTESIAN_POINT('Ctrl Pts',(-134.036910175617,5.96066703612229,151.608250755187));
#94692=CARTESIAN_POINT('Ctrl Pts',(-130.388289611904,5.11974710983809,151.608250755187));
#94693=CARTESIAN_POINT('Ctrl Pts',(-126.724082256978,4.37986325495167,151.608250755187));
#94694=CARTESIAN_POINT('Ctrl Pts',(-123.047843481659,3.71796898974137,151.608250755187));
#94695=CARTESIAN_POINT('Ctrl Pts',(-119.37160470634,3.05607472453107,151.608250755187));
#94696=CARTESIAN_POINT('Ctrl Pts',(-115.683294647706,2.47242844679211,151.608250755187));
#94697=CARTESIAN_POINT('Ctrl Pts',(-111.985363270584,1.95114909299883,151.608250755187));
#94698=CARTESIAN_POINT('Ctrl Pts',(-104.589500516342,0.908590385412271,
151.608250755187));
#94699=CARTESIAN_POINT('Ctrl Pts',(-97.1555011500406,0.113239291541015,
151.608250755187));
#94700=CARTESIAN_POINT('Ctrl Pts',(-89.6959049654537,-0.516189135775493,
151.608250755187));
#94701=CARTESIAN_POINT('Ctrl Pts',(-85.9661068731603,-0.830903349433756,
151.608250755187));
#94702=CARTESIAN_POINT('Ctrl Pts',(-82.2317153529779,-1.10324244351832,
151.608250755187));
#94703=CARTESIAN_POINT('Ctrl Pts',(-78.4978636089007,-1.3402031987625,151.608250755187));
#94704=CARTESIAN_POINT('Ctrl Pts',(-74.7640118648235,-1.57716395400667,
151.608250755187));
#94705=CARTESIAN_POINT('Ctrl Pts',(-71.0292449211827,-1.77883547864296,
151.608250755187));
#94706=CARTESIAN_POINT('Ctrl Pts',(-67.2937205242537,-1.95130031997899,
151.608250755187));
#94707=CARTESIAN_POINT('Ctrl Pts',(-59.8226717303959,-2.29623000265104,
151.608250755187));
#94708=CARTESIAN_POINT('Ctrl Pts',(-52.3486036457986,-2.52473868657067,
151.608250755187));
#94709=CARTESIAN_POINT('Ctrl Pts',(-44.8725449624828,-2.6764917642896,151.608250755187));
#94710=CARTESIAN_POINT('Ctrl Pts',(-37.3964862791671,-2.82824484200852,
151.608250755187));
#94711=CARTESIAN_POINT('Ctrl Pts',(-29.9184179909671,-2.90250945372239,
151.608250755187));
#94712=CARTESIAN_POINT('Ctrl Pts',(-22.4393041369209,-2.93645803410833,
151.608250755187));
#94713=CARTESIAN_POINT('Ctrl Pts',(-14.9601902828747,-2.97040661449427,
151.608250755187));
#94714=CARTESIAN_POINT('Ctrl Pts',(-7.47999428485685,-2.96262874562523,
151.608250755187));
#94715=CARTESIAN_POINT('Ctrl Pts',(7.58040827681699E-15,-2.96262874552467,
151.608250755187));
#94716=CARTESIAN_POINT('Ctrl Pts',(7.71069817591099E-15,-3.96262874552467,
150.608250755187));
#94717=CARTESIAN_POINT('Ctrl Pts',(-7.50819538729109,-3.96262874552467,
150.608250755187));
#94718=CARTESIAN_POINT('Ctrl Pts',(-15.016593604005,-3.97044580329555,150.608250755187));
#94719=CARTESIAN_POINT('Ctrl Pts',(-30.0312011445192,-3.90171985843133,
150.608250755187));
#94720=CARTESIAN_POINT('Ctrl Pts',(-37.5374476689956,-3.82661057201559,
150.608250755187));
#94721=CARTESIAN_POINT('Ctrl Pts',(-52.5458801835575,-3.51989876720754,
150.608250755187));
#94722=CARTESIAN_POINT('Ctrl Pts',(-60.0480854211127,-3.28903804741979,
150.608250755187));
#94723=CARTESIAN_POINT('Ctrl Pts',(-71.2968182978101,-2.76642698606123,
150.608250755187));
#94724=CARTESIAN_POINT('Ctrl Pts',(-75.0456307554615,-2.56273368294278,
150.608250755187));
#94725=CARTESIAN_POINT('Ctrl Pts',(-82.541406464583,-2.08407856275224,150.608250755187));
#94726=CARTESIAN_POINT('Ctrl Pts',(-86.2899316135277,-1.80901706075654,
150.608250755187));
#94727=CARTESIAN_POINT('Ctrl Pts',(-97.5206070789962,-0.855541349070317,
150.608250755187));
#94728=CARTESIAN_POINT('Ctrl Pts',(-104.981869714816,-0.0523559943782628,
150.608250755187));
#94729=CARTESIAN_POINT('Ctrl Pts',(-116.115973027981,1.52690259340425,150.608250755187));
#94730=CARTESIAN_POINT('Ctrl Pts',(-119.817620868547,2.11630680211849,150.608250755187));
#94731=CARTESIAN_POINT('Ctrl Pts',(-127.196527399596,3.45315573247565,150.608250755187));
#94732=CARTESIAN_POINT('Ctrl Pts',(-130.873826011882,4.20034176276589,150.608250755187));
#94733=CARTESIAN_POINT('Ctrl Pts',(-138.196939381026,5.89872768376561,150.608250755187));
#94734=CARTESIAN_POINT('Ctrl Pts',(-141.849976625069,6.85208769613199,150.608250755187));
#94735=CARTESIAN_POINT('Ctrl Pts',(-149.04273478531,9.01070097414105,150.608250755187));
#94736=CARTESIAN_POINT('Ctrl Pts',(-152.588815574637,10.2162896078986,150.608250755187));
#94737=CARTESIAN_POINT('Ctrl Pts',(-159.543790312038,12.9718966302658,150.608250755187));
#94738=CARTESIAN_POINT('Ctrl Pts',(-162.953403385689,14.5201095377957,150.608250755187));
#94739=CARTESIAN_POINT('Ctrl Pts',(-167.090526771118,16.7689396411949,150.608250755187));
#94740=CARTESIAN_POINT('Ctrl Pts',(-167.911603711878,17.2346426806634,150.608250755187));
#94741=CARTESIAN_POINT('Ctrl Pts',(-169.539551113397,18.2017164255323,150.608250755187));
#94742=CARTESIAN_POINT('Ctrl Pts',(-170.345912390848,18.7028771029668,150.608250755186));
#94743=CARTESIAN_POINT('Ctrl Pts',(-172.725350664097,20.2557684708299,150.608250755186));
#94744=CARTESIAN_POINT('Ctrl Pts',(-174.26395189805,21.3594575729593,150.608250755187));
#94745=CARTESIAN_POINT('Ctrl Pts',(-175.744203657372,22.5468679911664,150.608250755186));
#94746=CARTESIAN_POINT('Ctrl Pts',(175.744203657372,22.5468679911664,150.608250755187));
#94747=CARTESIAN_POINT('Ctrl Pts',(175.744203657372,22.5468679911664,151.608250755187));
#94748=CARTESIAN_POINT('Ctrl Pts',(175.118478031602,23.3269112215417,151.608250755187));
#94749=CARTESIAN_POINT('Ctrl Pts',(175.975959514274,22.7327750959766,150.611103966871));
#94750=CARTESIAN_POINT('Ctrl Pts',(175.973846570991,22.7347327109198,151.608250755179));
#94751=CARTESIAN_POINT('Ctrl Pts',(175.343331695395,23.5072816087761,151.608250755187));
#94752=CARTESIAN_POINT('Ctrl Pts',(176.204751595057,22.9213751497708,150.613904162808));
#94753=CARTESIAN_POINT('Ctrl Pts',(176.200864181503,22.9254545071624,151.608250755187));
#94754=CARTESIAN_POINT('Ctrl Pts',(175.565293759208,23.6902366406671,151.608250755187));
#94755=CARTESIAN_POINT('Ctrl Pts',(176.430593086108,23.1126512166033,150.616656461907));
#94756=CARTESIAN_POINT('Ctrl Pts',(176.425206487511,23.1190122335564,151.608250755187));
#94757=CARTESIAN_POINT('Ctrl Pts',(175.784380109018,23.8757620423259,151.608250755187));
#94758=CARTESIAN_POINT('',(175.118478031602,23.3269112215418,151.608250755187));
#94759=CARTESIAN_POINT('',(175.744216329386,22.5468739627075,150.608257703203));
#94760=CARTESIAN_POINT('Origin',(175.118478031602,23.3269112215418,150.608250755187));
#94761=CARTESIAN_POINT('Origin',(154.866194135799,48.5801870238026,150.281756698687));
#94762=CARTESIAN_POINT('Origin',(154.804630199197,48.6513971212518,151.608250754784));
#94763=CARTESIAN_POINT('Ctrl Pts',(175.118478031529,23.3269112214834,151.608250755187));
#94764=CARTESIAN_POINT('Ctrl Pts',(175.744203657298,22.546867991107,151.608250755187));
#94765=CARTESIAN_POINT('Ctrl Pts',(175.744203657298,22.546867991107,150.608250755187));
#94766=CARTESIAN_POINT('Ctrl Pts',(173.120080073127,21.7238605655503,151.608250755187));
#94767=CARTESIAN_POINT('Ctrl Pts',(173.707215155453,20.9128612407145,151.608250755436));
#94768=CARTESIAN_POINT('Ctrl Pts',(173.707215156076,20.9128612399726,150.608250755435));
#94769=CARTESIAN_POINT('Ctrl Pts',(171.037782482163,20.2938924020537,151.608250755187));
#94770=CARTESIAN_POINT('Ctrl Pts',(171.589969109119,19.4593526556396,151.608250755187));
#94771=CARTESIAN_POINT('Ctrl Pts',(171.589969109234,19.4593526554507,150.608250755187));
#94772=CARTESIAN_POINT('Ctrl Pts',(166.754172906568,17.6818243599797,151.608250755187));
#94773=CARTESIAN_POINT('Ctrl Pts',(167.243233378372,16.8087914199981,151.608250755187));
#94774=CARTESIAN_POINT('Ctrl Pts',(167.243233378257,16.8087914201871,150.608250755187));
#94775=CARTESIAN_POINT('Ctrl Pts',(164.55225250787,16.5005018421618,151.608250755187));
#94776=CARTESIAN_POINT('Ctrl Pts',(165.013075266338,15.6125556413792,151.608250755187));
#94777=CARTESIAN_POINT('Ctrl Pts',(165.013075266415,15.6125556412203,150.608250755187));
#94778=CARTESIAN_POINT('Ctrl Pts',(160.0571058438,14.3272733601118,151.608250755187));
#94779=CARTESIAN_POINT('Ctrl Pts',(160.466806870505,13.414611791432,151.608250755187));
#94780=CARTESIAN_POINT('Ctrl Pts',(160.466806870428,13.4146117915908,150.608250755187));
#94781=CARTESIAN_POINT('Ctrl Pts',(157.763687679101,13.3357654966317,151.608250755187));
#94782=CARTESIAN_POINT('Ctrl Pts',(158.150493359254,12.4133327114123,151.608250755152));
#94783=CARTESIAN_POINT('Ctrl Pts',(158.150493359297,12.4133327113047,150.608250755152));
#94784=CARTESIAN_POINT('Ctrl Pts',(153.104239295307,11.5033854913725,151.608250755187));
#94785=CARTESIAN_POINT('Ctrl Pts',(153.449389725816,10.5645713149919,151.608250755221));
#94786=CARTESIAN_POINT('Ctrl Pts',(153.449389725773,10.5645713150995,150.608250755221));
#94787=CARTESIAN_POINT('Ctrl Pts',(150.738093671782,10.6627043727942,151.608250755187));
#94788=CARTESIAN_POINT('Ctrl Pts',(151.064489900424,9.71729891062486,151.608250755222));
#94789=CARTESIAN_POINT('Ctrl Pts',(151.064489900386,9.71729891075825,150.608250755222));
#94790=CARTESIAN_POINT('Ctrl Pts',(148.342276748097,9.8836739626675,151.608250755187));
#94791=CARTESIAN_POINT('Ctrl Pts',(148.651502801043,8.93268539902455,151.608250755187));
#94792=CARTESIAN_POINT('Ctrl Pts',(148.651502801043,8.93268539902455,150.608250755187));
#94793=CARTESIAN_POINT('Ctrl Pts',(150.890074370997,10.7399699375689,151.608250755187));
#94794=CARTESIAN_POINT('Ctrl Pts',(152.418601106946,11.2709967454126,151.608250755187));
#94795=CARTESIAN_POINT('Ctrl Pts',(153.933840147718,11.829615202147,151.608250755022));
#94796=CARTESIAN_POINT('Ctrl Pts',(155.433971914984,12.4195540635097,151.608250754921));
#94797=CARTESIAN_POINT('Ctrl Pts',(156.056167411372,12.664237437793,151.60825075488));
#94798=CARTESIAN_POINT('Ctrl Pts',(156.675772237677,12.9142950898713,151.60825075491));
#94799=CARTESIAN_POINT('Ctrl Pts',(157.292603196614,13.1701058677585,151.608250755012));
#94800=CARTESIAN_POINT('Ctrl Pts',(158.98541137872,13.8721435518337,151.608250755293));
#94801=CARTESIAN_POINT('Ctrl Pts',(160.657393444049,14.6173931442985,151.60825075146));
#94802=CARTESIAN_POINT('Ctrl Pts',(162.304716085384,15.4138112567312,151.608250751591));
#94803=CARTESIAN_POINT('Ctrl Pts',(162.70488712863,15.6072788015308,151.608250751623));
#94804=CARTESIAN_POINT('Ctrl Pts',(163.103608897851,15.803753154363,151.608250752144));
#94805=CARTESIAN_POINT('Ctrl Pts',(163.500798283409,16.003405836179,151.608250752999));
#94806=CARTESIAN_POINT('Ctrl Pts',(164.887524176526,16.7004625893846,151.608250755985));
#94807=CARTESIAN_POINT('Ctrl Pts',(166.255673442885,17.4360498920816,151.608250748576));
#94808=CARTESIAN_POINT('Ctrl Pts',(167.601685487584,18.2175677714455,151.608250744422));
#94809=CARTESIAN_POINT('Ctrl Pts',(168.035481204944,18.4694370696759,151.608250743083));
#94810=CARTESIAN_POINT('Ctrl Pts',(168.466977276069,18.7260768217338,151.608250742812));
#94811=CARTESIAN_POINT('Ctrl Pts',(168.896053436859,18.9877341686053,151.608250744604));
#94812=CARTESIAN_POINT('Ctrl Pts',(169.086720473706,19.1040059067164,151.6082507454));
#94813=CARTESIAN_POINT('Ctrl Pts',(169.276914485451,19.2212622613973,151.60825074658));
#94814=CARTESIAN_POINT('Ctrl Pts',(169.466617875306,19.3395384011703,151.608250747987));
#94815=CARTESIAN_POINT('Ctrl Pts',(170.713449384169,20.1169120576391,151.608250757236));
#94816=CARTESIAN_POINT('Ctrl Pts',(171.939119545222,20.9381212638537,151.608250755117));
#94817=CARTESIAN_POINT('Ctrl Pts',(173.138860719752,21.8131269850015,151.608250755171));
#94818=CARTESIAN_POINT('Ctrl Pts',(173.807052403966,22.3004583852424,151.608250755202));
#94819=CARTESIAN_POINT('Ctrl Pts',(174.467200766754,22.8044775175799,151.608250755187));
#94820=CARTESIAN_POINT('Ctrl Pts',(175.118478031529,23.3269112214834,151.608250755187));
#94821=CARTESIAN_POINT('Ctrl Pts',(175.744203657372,22.5468679911664,150.608250755187));
#94822=CARTESIAN_POINT('Ctrl Pts',(173.733839581004,20.9342184982058,150.608250755187));
#94823=CARTESIAN_POINT('Ctrl Pts',(171.640407580167,19.493722137766,150.608250755187));
#94824=CARTESIAN_POINT('Ctrl Pts',(167.333937892112,16.8606047997096,150.608250755187));
#94825=CARTESIAN_POINT('Ctrl Pts',(165.12049074122,15.6688324102149,150.608250755187));
#94826=CARTESIAN_POINT('Ctrl Pts',(160.601711271341,13.4757139554807,150.608250755187));
#94827=CARTESIAN_POINT('Ctrl Pts',(158.296197081565,12.4747448061917,150.608250755187));
#94828=CARTESIAN_POINT('Ctrl Pts',(153.611908863468,10.6246329890705,150.608250755187));
#94829=CARTESIAN_POINT('Ctrl Pts',(151.233043212517,9.77568020346336,150.608250755187));
#94830=CARTESIAN_POINT('Ctrl Pts',(148.824154304563,8.98894875990614,150.608250755187));
#94831=CARTESIAN_POINT('Origin',(-205.7,-9.35236728728476,151.608250755187));
#94832=CARTESIAN_POINT('',(-178.303739692644,23.8757620423259,151.608250755187));
#94833=CARTESIAN_POINT('',(-178.303739692644,23.8757620423259,151.608250755187));
#94834=CARTESIAN_POINT('Ctrl Pts',(7.105427357601E-15,-2.96262874552467,
151.608250755187));
#94835=CARTESIAN_POINT('Ctrl Pts',(9.02624649977933,-2.9626287456421,151.608250755187));
#94836=CARTESIAN_POINT('Ctrl Pts',(18.0527444291047,-2.9728621931889,151.60825074306));
#94837=CARTESIAN_POINT('Ctrl Pts',(27.0774432067146,-2.91001683511451,151.608250751144));
#94838=CARTESIAN_POINT('Ctrl Pts',(27.3305429265962,-2.9082543228228,151.608250751371));
#94839=CARTESIAN_POINT('Ctrl Pts',(27.5836412653319,-2.90643461439096,151.608250751582));
#94840=CARTESIAN_POINT('Ctrl Pts',(27.8367381802904,-2.90455588038999,151.608250751779));
#94841=CARTESIAN_POINT('Ctrl Pts',(36.6082400286613,-2.83944517461597,151.608250758593));
#94842=CARTESIAN_POINT('Ctrl Pts',(45.3780717103661,-2.70648749187338,151.608250755332));
#94843=CARTESIAN_POINT('Ctrl Pts',(54.1447641976466,-2.44599594155881,151.608250755033));
#94844=CARTESIAN_POINT('Ctrl Pts',(54.6506804038063,-2.43096325995591,151.608250755016));
#94845=CARTESIAN_POINT('Ctrl Pts',(55.1565862129384,-2.41550562764502,151.608250755));
#94846=CARTESIAN_POINT('Ctrl Pts',(55.6624813336477,-2.39961161868985,151.608250754986));
#94847=CARTESIAN_POINT('Ctrl Pts',(64.1758609249135,-2.13214169078735,151.608250754755));
#94848=CARTESIAN_POINT('Ctrl Pts',(72.6862574775868,-1.74295631081683,151.608250759293));
#94849=CARTESIAN_POINT('Ctrl Pts',(81.1919376197577,-1.16313723768181,151.608250750562));
#94850=CARTESIAN_POINT('Ctrl Pts',(81.9500796395524,-1.11145586760035,151.608250749784));
#94851=CARTESIAN_POINT('Ctrl Pts',(82.7082017514622,-1.05825235857909,151.608250749472));
#94852=CARTESIAN_POINT('Ctrl Pts',(83.4662947054053,-1.00347988218016,151.60825074959));
#94853=CARTESIAN_POINT('Ctrl Pts',(86.6559785797055,-0.773024126304283,
151.608250750086));
#94854=CARTESIAN_POINT('Ctrl Pts',(89.8432471884515,-0.514663737175523,
151.608250754812));
#94855=CARTESIAN_POINT('Ctrl Pts',(93.024774958763,-0.223757922142914,151.608250755027));
#94856=CARTESIAN_POINT('Ctrl Pts',(93.5808398870228,-0.172913631963855,
151.608250755064));
#94857=CARTESIAN_POINT('Ctrl Pts',(94.1367294898188,-0.121075272080125,
151.608250755069));
#94858=CARTESIAN_POINT('Ctrl Pts',(94.6924260755016,-0.068218227171274,
151.60825075503));
#94859=CARTESIAN_POINT('Ctrl Pts',(95.5740503470334,0.0156405815990452,
151.608250754969));
#94860=CARTESIAN_POINT('Ctrl Pts',(96.4552583878779,0.102078414550722,151.608250754932));
#94861=CARTESIAN_POINT('Ctrl Pts',(97.3359839441123,0.19119707264984,151.608250754931));
#94862=CARTESIAN_POINT('Ctrl Pts',(100.941451049396,0.556026261457694,151.608250754926));
#94863=CARTESIAN_POINT('Ctrl Pts',(104.539950590689,0.965744460923742,151.608250755187));
#94864=CARTESIAN_POINT('Ctrl Pts',(108.129330685163,1.43018233510906,151.608250755187));
#94865=CARTESIAN_POINT('',(-178.303739692644,23.8757620423259,151.608250755187));
#94866=CARTESIAN_POINT('',(-178.303739692644,23.8757620423259,151.608250755187));
#94867=CARTESIAN_POINT('Origin',(-160.5,51.8013867006571,102.225104347671));
#94868=CARTESIAN_POINT('',(-190.499797482064,51.8013867006572,102.335336081498));
#94869=CARTESIAN_POINT('',(-190.499797482064,59.,102.335336081498));
#94870=CARTESIAN_POINT('',(-190.5,51.8013867006572,102.225104347682));
#94871=CARTESIAN_POINT('',(-190.5,59.,102.225104347671));
#94872=CARTESIAN_POINT('Origin',(-160.5,51.8013867006572,102.225104347682));
#94873=CARTESIAN_POINT('Ctrl Pts',(-190.491663305814,52.7378649121229,102.843638895579));
#94874=CARTESIAN_POINT('Ctrl Pts',(-190.497736632342,52.3999363590591,102.904908304561));
#94875=CARTESIAN_POINT('Ctrl Pts',(-190.497486577525,52.0619530244292,102.966101522029));
#94876=CARTESIAN_POINT('Ctrl Pts',(-190.500794397929,52.1777803689832,102.165012668779));
#94877=CARTESIAN_POINT('Ctrl Pts',(-190.500218467073,52.0402913792871,102.219565731378));
#94878=CARTESIAN_POINT('Ctrl Pts',(-190.500020296148,51.9028032385845,102.274119986721));
#94879=CARTESIAN_POINT('Ctrl Pts',(-190.500380950584,51.8120846909133,102.197587822659));
#94880=CARTESIAN_POINT('Ctrl Pts',(-190.500101610712,51.8080280356141,102.252459235273));
#94881=CARTESIAN_POINT('Ctrl Pts',(-190.499901046205,51.8039712376326,102.307330335762));
#94882=CARTESIAN_POINT('Ctrl Pts',(-190.499485036411,51.5910001868266,102.262672212471));
#94883=CARTESIAN_POINT('Ctrl Pts',(-190.499861738055,51.6678861088951,102.318186867608));
#94884=CARTESIAN_POINT('Ctrl Pts',(-190.499656096965,51.7447735126223,102.373700417183));
#94885=CARTESIAN_POINT('Ctrl Pts',(-190.499276641726,51.5555442395852,102.277696646539));
#94886=CARTESIAN_POINT('Ctrl Pts',(-190.499806182338,51.6454376861142,102.333360080156));
#94887=CARTESIAN_POINT('Ctrl Pts',(-190.499599365699,51.7353333285508,102.389022107829));
#94888=CARTESIAN_POINT('Ctrl Pts',(-190.498637284839,51.4609849811862,102.323405682444));
#94889=CARTESIAN_POINT('Ctrl Pts',(-190.49963641837,51.5856027243035,102.379522755427));
#94890=CARTESIAN_POINT('Ctrl Pts',(-190.499425997259,51.7102254535205,102.435637407256));
#94891=CARTESIAN_POINT('Ctrl Pts',(-190.498179537645,51.4122959822613,102.355661727505));
#94892=CARTESIAN_POINT('Ctrl Pts',(-190.499515675854,51.5548458240518,102.412100111793));
#94893=CARTESIAN_POINT('Ctrl Pts',(-190.49930268195,51.6974029923146,102.468535392115));
#94894=CARTESIAN_POINT('Ctrl Pts',(-190.496764137211,51.2786905629959,102.453983419634));
#94895=CARTESIAN_POINT('Ctrl Pts',(-190.49914429648,51.4705106049134,102.511405737649));
#94896=CARTESIAN_POINT('Ctrl Pts',(-190.498923349085,51.6623471528931,102.568822318432));
#94897=CARTESIAN_POINT('Ctrl Pts',(-190.495771571132,51.209415072178,102.521125183006));
#94898=CARTESIAN_POINT('Ctrl Pts',(-190.498886347067,51.4268861937162,102.579224820903));
#94899=CARTESIAN_POINT('Ctrl Pts',(-190.498659830336,51.6443814238632,102.63731713971));
#94900=CARTESIAN_POINT('Ctrl Pts',(-190.492708303722,51.0187369204825,102.723145628418));
#94901=CARTESIAN_POINT('Ctrl Pts',(-190.498096192236,51.3069405894523,102.783302214059));
#94902=CARTESIAN_POINT('Ctrl Pts',(-190.497852468908,51.5951979523677,102.843444114641));
#94903=CARTESIAN_POINT('Ctrl Pts',(-190.490539813272,50.917161842527,102.85947607439));
#94904=CARTESIAN_POINT('Ctrl Pts',(-190.497544477131,51.2432568804925,102.921043654985));
#94905=CARTESIAN_POINT('Ctrl Pts',(-190.497288537386,51.569430449523,102.982592460488));
#94906=CARTESIAN_POINT('Ctrl Pts',(-190.483704239377,50.6334868253324,103.269643650079));
#94907=CARTESIAN_POINT('Ctrl Pts',(-190.49582522282,51.0656966540016,103.335535923897));
#94908=CARTESIAN_POINT('Ctrl Pts',(-190.495530565148,51.4980839253095,103.401385430389));
#94909=CARTESIAN_POINT('Ctrl Pts',(-190.478715221144,50.4768968387938,103.544270661594));
#94910=CARTESIAN_POINT('Ctrl Pts',(-190.494595543656,50.9681482986425,103.61315472568));
#94911=CARTESIAN_POINT('Ctrl Pts',(-190.494272325443,51.4596635555447,103.681982740741));
#94912=CARTESIAN_POINT('Ctrl Pts',(-190.462385362509,50.029883727716,104.369079428756));
#94913=CARTESIAN_POINT('Ctrl Pts',(-190.490647214857,50.6904232796527,104.447283745944));
#94914=CARTESIAN_POINT('Ctrl Pts',(-190.490229110897,51.3515886158552,104.525337933961));
#94915=CARTESIAN_POINT('Ctrl Pts',(-190.449683809442,49.7677262399101,104.92040760936));
#94916=CARTESIAN_POINT('Ctrl Pts',(-190.487668736046,50.5286860699985,105.005251885913));
#94917=CARTESIAN_POINT('Ctrl Pts',(-190.487175061528,51.2906141049957,105.089881803614));
#94918=CARTESIAN_POINT('Ctrl Pts',(-190.419875471187,49.2494562758818,106.023570052378));
#94919=CARTESIAN_POINT('Ctrl Pts',(-190.48093224589,50.2104897205784,106.122573675973));
#94920=CARTESIAN_POINT('Ctrl Pts',(-190.480254718442,51.1734947861719,106.22126805386));
#94921=CARTESIAN_POINT('Ctrl Pts',(-190.402769507585,48.9964283476031,106.575456298919));
#94922=CARTESIAN_POINT('Ctrl Pts',(-190.477173973333,50.0559837220552,106.682014500456));
#94923=CARTESIAN_POINT('Ctrl Pts',(-190.476388550459,51.1181863857103,106.788162672421));
#94924=CARTESIAN_POINT('Ctrl Pts',(-190.363099295219,48.4854361039805,107.679453599572));
#94925=CARTESIAN_POINT('Ctrl Pts',(-190.46877721616,49.7454964240051,107.802071096718));
#94926=CARTESIAN_POINT('Ctrl Pts',(-190.467733478659,51.0100384384107,107.924109474718));
#94927=CARTESIAN_POINT('Ctrl Pts',(-190.340537373167,48.2278592407325,108.231574631801));
#94928=CARTESIAN_POINT('Ctrl Pts',(-190.464138162999,49.5897493763273,108.36274109052));
#94929=CARTESIAN_POINT('Ctrl Pts',(-190.462944593205,50.9573036985215,108.493171689549));
#94930=CARTESIAN_POINT('Ctrl Pts',(-190.262632780692,47.4366289996939,109.888091607918));
#94931=CARTESIAN_POINT('Ctrl Pts',(-190.448733141734,49.1135245761933,110.046748125528));
#94932=CARTESIAN_POINT('Ctrl Pts',(-190.447010747744,50.8008981564959,110.203650811467));
#94933=CARTESIAN_POINT('Ctrl Pts',(-190.197333416625,46.8843769038143,110.992633024223));
#94934=CARTESIAN_POINT('Ctrl Pts',(-190.436483465423,48.7840526999304,111.171862472543));
#94935=CARTESIAN_POINT('Ctrl Pts',(-190.434305733042,50.6989369523421,111.34834113016));
#94936=CARTESIAN_POINT('Ctrl Pts',(-190.024035203772,45.6901117243083,113.201763481001));
#94937=CARTESIAN_POINT('Ctrl Pts',(-190.40704122806,48.0776487632177,113.426803183689));
#94938=CARTESIAN_POINT('Ctrl Pts',(-190.403599601366,50.4961283561593,113.647636636137));
#94939=CARTESIAN_POINT('Ctrl Pts',(-189.916118308262,45.0481787304179,114.306444419514));
#94940=CARTESIAN_POINT('Ctrl Pts',(-190.389831561577,47.7005628031284,114.557490865841));
#94941=CARTESIAN_POINT('Ctrl Pts',(-190.385599241613,50.3954125375369,114.802333478777));
#94942=CARTESIAN_POINT('Ctrl Pts',(-189.632120997169,43.6438029112513,116.515418563294));
#94943=CARTESIAN_POINT('Ctrl Pts',(-190.349296245468,46.8797597830052,116.824076695157));
#94944=CARTESIAN_POINT('Ctrl Pts',(-190.342926802733,50.1951730686192,117.12309103697));
#94945=CARTESIAN_POINT('Ctrl Pts',(-189.455515647208,42.8796590900541,117.619682593116));
#94946=CARTESIAN_POINT('Ctrl Pts',(-190.325937170929,46.4346322736547,117.961190795854));
#94947=CARTESIAN_POINT('Ctrl Pts',(-190.318259073436,50.0957162763353,118.289113661344));
#94948=CARTESIAN_POINT('Ctrl Pts',(-189.002145676919,41.2276412744401,119.827671012508));
#94949=CARTESIAN_POINT('Ctrl Pts',(-190.271688789567,45.4690939131192,120.241849554135));
#94950=CARTESIAN_POINT('Ctrl Pts',(-190.260543746634,49.8985024053798,120.634770552665));
#94951=CARTESIAN_POINT('Ctrl Pts',(-188.723384078107,40.3379738271532,120.931404423614));
#94952=CARTESIAN_POINT('Ctrl Pts',(-190.240733969511,44.9465217448158,121.387150250019));
#94953=CARTESIAN_POINT('Ctrl Pts',(-190.227500694656,49.800817210661,121.814404993884));
#94954=CARTESIAN_POINT('Ctrl Pts',(-188.06484104112,38.5294426245587,123.138051727137));
#94955=CARTESIAN_POINT('Ctrl Pts',(-190.169533062177,43.8657138954457,123.686077965342));
#94956=CARTESIAN_POINT('Ctrl Pts',(-190.150875780102,49.6062079663902,124.190105192337));
#94957=CARTESIAN_POINT('Ctrl Pts',(-187.68678109675,37.6174522484167,124.240963108104));
#94958=CARTESIAN_POINT('Ctrl Pts',(-190.129193199196,43.3099745219927,124.841340387957));
#94959=CARTESIAN_POINT('Ctrl Pts',(-190.10730109644,49.5092579859229,125.38615523586));
#94960=CARTESIAN_POINT('Ctrl Pts',(-186.887860552158,35.8988473048903,126.445328122734));
#94961=CARTESIAN_POINT('Ctrl Pts',(-190.036990023442,42.2318697577437,127.162839519027));
#94962=CARTESIAN_POINT('Ctrl Pts',(-190.006839455965,49.312572598589,127.798107978239));
#94963=CARTESIAN_POINT('Ctrl Pts',(-186.468827260737,35.0921688914378,127.546773447421));
#94964=CARTESIAN_POINT('Ctrl Pts',(-189.985031715257,41.709649458652,128.329913067888));
#94965=CARTESIAN_POINT('Ctrl Pts',(-189.94996479732,49.2127662094606,129.013981648704));
#94966=CARTESIAN_POINT('Ctrl Pts',(-185.622971106415,33.5951852320465,129.74743532292));
#94967=CARTESIAN_POINT('Ctrl Pts',(-189.866769695801,40.7086313682495,130.678624682498));
#94968=CARTESIAN_POINT('Ctrl Pts',(-189.819235897465,49.0062073327181,131.470286553815));
#94969=CARTESIAN_POINT('Ctrl Pts',(-185.195344088968,32.9022054207578,130.846652192156));
#94970=CARTESIAN_POINT('Ctrl Pts',(-189.800375510914,40.2286538411534,131.860497562516));
#94971=CARTESIAN_POINT('Ctrl Pts',(-189.745402573328,48.8994524120374,132.710684641086));
#94972=CARTESIAN_POINT('Ctrl Pts',(-184.332316899999,31.5951495873319,133.042097933749));
#94973=CARTESIAN_POINT('Ctrl Pts',(-189.649582724457,39.2936837439378,134.243547879917));
#94974=CARTESIAN_POINT('Ctrl Pts',(-189.575717682786,48.6755045049199,135.222940428359));
#94975=CARTESIAN_POINT('Ctrl Pts',(-183.896498248529,30.9805270643031,134.138330157969));
#94976=CARTESIAN_POINT('Ctrl Pts',(-189.56508157479,38.8385274591103,135.444827376579));
#94977=CARTESIAN_POINT('Ctrl Pts',(-189.479904579247,48.5583284722341,136.494741229239));
#94978=CARTESIAN_POINT('Ctrl Pts',(-183.007879854772,29.7992916323161,136.326983635148));
#94979=CARTESIAN_POINT('Ctrl Pts',(-189.373108647856,37.9355866103639,137.873607563424));
#94980=CARTESIAN_POINT('Ctrl Pts',(-189.259006538894,48.3103221431259,139.080158339632));
#94981=CARTESIAN_POINT('Ctrl Pts',(-182.555006195201,29.2327350916608,137.419409487353));
#94982=CARTESIAN_POINT('Ctrl Pts',(-189.265506543082,37.4878383145516,139.101327514706));
#94983=CARTESIAN_POINT('Ctrl Pts',(-189.13399969732,48.1795106830979,140.393659401794));
#94984=CARTESIAN_POINT('Ctrl Pts',(-181.620484012305,28.1255995839538,139.599441768215));
#94985=CARTESIAN_POINT('Ctrl Pts',(-189.02019842515,36.5848378699127,141.594013188396));
#94986=CARTESIAN_POINT('Ctrl Pts',(-188.843611611567,47.9007227666897,143.078697426969));
#94987=CARTESIAN_POINT('Ctrl Pts',(-181.138886935942,27.5851446107169,140.687055901723));
#94988=CARTESIAN_POINT('Ctrl Pts',(-188.882324844217,36.1295124585929,142.859405486123));
#94989=CARTESIAN_POINT('Ctrl Pts',(-188.678410370255,47.7527728507809,144.449973724618));
#94990=CARTESIAN_POINT('Ctrl Pts',(-180.132246584594,26.5129406317024,142.856096076585));
#94991=CARTESIAN_POINT('Ctrl Pts',(-188.565410200897,35.1965622431075,145.446412027918));
#94992=CARTESIAN_POINT('Ctrl Pts',(-188.289138096809,47.4352589096868,147.277825831555));
#94993=CARTESIAN_POINT('Ctrl Pts',(-179.607362760168,25.9813342957967,143.937538719537));
#94994=CARTESIAN_POINT('Ctrl Pts',(-188.386181827197,34.7187059931883,146.768668767197));
#94995=CARTESIAN_POINT('Ctrl Pts',(-188.06556355209,47.2657487316501,148.733707236845));
#94996=CARTESIAN_POINT('Ctrl Pts',(-178.771977332917,25.1780519636145,145.553513839897));
#94997=CARTESIAN_POINT('Ctrl Pts',(-188.072685289982,33.9724700260299,148.817294700524));
#94998=CARTESIAN_POINT('Ctrl Pts',(-187.659901468284,46.9904063042588,151.019801324971));
#94999=CARTESIAN_POINT('Ctrl Pts',(-178.485447212846,24.909306929138,146.091134114406));
#95000=CARTESIAN_POINT('Ctrl Pts',(-187.960223656828,33.717865232546,149.513668849716));
#95001=CARTESIAN_POINT('Ctrl Pts',(-187.512808021989,46.8950932019447,151.799103801632));
#95002=CARTESIAN_POINT('Ctrl Pts',(-177.89247216804,24.3673914569808,147.163909925698));
#95003=CARTESIAN_POINT('Ctrl Pts',(-187.7158093276,33.1945722270689,150.938584532678));
#95004=CARTESIAN_POINT('Ctrl Pts',(-187.186802763605,46.69618951942,153.40385117349));
#95005=CARTESIAN_POINT('Ctrl Pts',(-177.586052240338,24.0942352060037,147.69906801671));
#95006=CARTESIAN_POINT('Ctrl Pts',(-187.583772753384,32.9257648233002,151.667406988934));
#95007=CARTESIAN_POINT('Ctrl Pts',(-187.008003041589,46.5926072881889,154.229151155406));
#95008=CARTESIAN_POINT('Ctrl Pts',(-176.948143217813,23.5404470288426,148.766384943322));
#95009=CARTESIAN_POINT('Ctrl Pts',(-187.293812193883,32.3688904562231,153.170780717094));
#95010=CARTESIAN_POINT('Ctrl Pts',(-186.605647008022,46.3754949682409,155.944107159623));
#95011=CARTESIAN_POINT('Ctrl Pts',(-176.616706877241,23.2598444410281,149.298549155497));
#95012=CARTESIAN_POINT('Ctrl Pts',(-187.135798229102,32.0806671907642,153.945676070019));
#95013=CARTESIAN_POINT('Ctrl Pts',(-186.382371628933,46.2619825739634,156.833415590026));
#95014=CARTESIAN_POINT('Ctrl Pts',(-175.921123207185,22.68689689322,150.359084407924));
#95015=CARTESIAN_POINT('Ctrl Pts',(-186.78295328971,31.4765317295405,155.56522059985));
#95016=CARTESIAN_POINT('Ctrl Pts',(-185.86783817509,46.0225121039273,158.708068090631));
#95017=CARTESIAN_POINT('Ctrl Pts',(-175.556345307998,22.3940330134238,150.888497532651));
#95018=CARTESIAN_POINT('Ctrl Pts',(-186.58766639389,31.1597913758803,156.411907710318));
#95019=CARTESIAN_POINT('Ctrl Pts',(-185.576751299258,45.8963336811167,159.694503161785));
#95020=CARTESIAN_POINT('Ctrl Pts',(-174.977689406787,21.9427305260402,151.675396018314));
#95021=CARTESIAN_POINT('Ctrl Pts',(-186.252891316275,30.6548993698614,157.762856154212));
#95022=CARTESIAN_POINT('Ctrl Pts',(-185.055116025266,45.6954835717082,161.286489264472));
#95023=CARTESIAN_POINT('Ctrl Pts',(-174.780131262563,21.7907501675503,151.935659078575));
#95024=CARTESIAN_POINT('Ctrl Pts',(-186.134203124744,30.4815764712039,158.226875047));
#95025=CARTESIAN_POINT('Ctrl Pts',(-184.86739764927,45.6268041466984,161.834467135961));
#95026=CARTESIAN_POINT('Ctrl Pts',(-174.373917956148,21.4827711935778,152.451438547147));
#95027=CARTESIAN_POINT('Ctrl Pts',(-185.878705051747,30.122557034981,159.190342309378));
#95028=CARTESIAN_POINT('Ctrl Pts',(-184.453669466243,45.4854241746709,162.977435749436));
#95029=CARTESIAN_POINT('Ctrl Pts',(-174.165275538502,21.3267796903352,152.706959670213));
#95030=CARTESIAN_POINT('Ctrl Pts',(-185.741837597343,29.9367780900454,159.689993905649));
#95031=CARTESIAN_POINT('Ctrl Pts',(-184.227834488115,45.4127279366936,163.57226076685));
#95032=CARTESIAN_POINT('Ctrl Pts',(-173.734439484061,21.0094771153743,153.212317702731));
#95033=CARTESIAN_POINT('Ctrl Pts',(-185.442647757005,29.5479163706511,160.741061501243));
#95034=CARTESIAN_POINT('Ctrl Pts',(-183.720111579081,45.2625191728524,164.828753901589));
#95035=CARTESIAN_POINT('Ctrl Pts',(-173.512272690491,20.8481811116799,153.462164515318));
#95036=CARTESIAN_POINT('Ctrl Pts',(-185.280285255813,29.3447366612225,161.292714722918));
#95037=CARTESIAN_POINT('Ctrl Pts',(-183.438667186176,45.1850157200236,165.490044607484));
#95038=CARTESIAN_POINT('Ctrl Pts',(-173.050663888627,20.5182754311735,153.954763169577));
#95039=CARTESIAN_POINT('Ctrl Pts',(-184.916469656588,28.912060268967,162.477578251216));
#95040=CARTESIAN_POINT('Ctrl Pts',(-182.786281071338,45.0239741908854,166.914420710284));
#95041=CARTESIAN_POINT('Ctrl Pts',(-172.811285296472,20.3497013053525,154.197538421658));
#95042=CARTESIAN_POINT('Ctrl Pts',(-184.715109947839,28.6824943845155,163.111019415201));
#95043=CARTESIAN_POINT('Ctrl Pts',(-182.416611477759,44.9404575123914,167.676642584149));
#95044=CARTESIAN_POINT('Ctrl Pts',(-172.309018538915,20.0018559561541,154.673652378991));
#95045=CARTESIAN_POINT('Ctrl Pts',(-184.243978355941,28.1780553452027,164.520194582625));
#95046=CARTESIAN_POINT('Ctrl Pts',(-181.515829713772,44.7653314719405,169.370362068887));
#95047=CARTESIAN_POINT('Ctrl Pts',(-172.045925480568,19.8224282462785,154.907331215004));
#95048=CARTESIAN_POINT('Ctrl Pts',(-183.974169315528,27.9027184380179,165.298511579777));
#95049=CARTESIAN_POINT('Ctrl Pts',(-180.986839328195,44.6736488797049,170.303040533204));
#95050=CARTESIAN_POINT('Ctrl Pts',(-171.625945202672,19.5411769387697,155.246607689634));
#95051=CARTESIAN_POINT('Ctrl Pts',(-183.465863550883,27.423666236785,166.663047270596));
#95052=CARTESIAN_POINT('Ctrl Pts',(-179.945305056306,44.5275110953375,171.919856198926));
#95053=CARTESIAN_POINT('Ctrl Pts',(-171.482771006779,19.4461136400241,155.356899985026));
#95054=CARTESIAN_POINT('Ctrl Pts',(-183.278745110663,27.2528822960182,167.15099067036));
#95055=CARTESIAN_POINT('Ctrl Pts',(-179.557764749393,44.4777268164602,172.491992949612));
#95056=CARTESIAN_POINT('Ctrl Pts',(-171.188847173927,19.2527442241094,155.570893173036));
#95057=CARTESIAN_POINT('Ctrl Pts',(-182.858413959778,26.8834361487309,168.198730392038));
#95058=CARTESIAN_POINT('Ctrl Pts',(-178.678365949149,44.3756234802552,173.702488528128));
#95059=CARTESIAN_POINT('Ctrl Pts',(-171.038069041094,19.154419880975,155.674573264278));
#95060=CARTESIAN_POINT('Ctrl Pts',(-182.623941443772,26.6839205445033,168.761056756381));
#95061=CARTESIAN_POINT('Ctrl Pts',(-178.184545903382,44.3232947364561,174.342353684468));
#95062=CARTESIAN_POINT('Ctrl Pts',(-170.727951753196,18.9541141206573,155.874480212679));
#95063=CARTESIAN_POINT('Ctrl Pts',(-182.106163264014,26.2568588794142,169.929834066643));
#95064=CARTESIAN_POINT('Ctrl Pts',(-177.102347209724,44.2157955625374,175.639812340165));
#95065=CARTESIAN_POINT('Ctrl Pts',(-170.568582074872,18.8521156515048,155.970683147523));
#95066=CARTESIAN_POINT('Ctrl Pts',(-181.82239246479,26.0290489673764,170.535242403614));
#95067=CARTESIAN_POINT('Ctrl Pts',(-176.51488906461,44.1606146875356,176.294574849227));
#95068=CARTESIAN_POINT('Ctrl Pts',(-170.241606120522,18.6449123730739,156.155713131299));
#95069=CARTESIAN_POINT('Ctrl Pts',(-181.232293959555,25.5638692026676,171.70630221824));
#95070=CARTESIAN_POINT('Ctrl Pts',(-175.330183039519,44.0475587900912,177.520910260544));
#95071=CARTESIAN_POINT('Ctrl Pts',(-170.07403552873,18.5397328103892,156.244564605491));
#95072=CARTESIAN_POINT('Ctrl Pts',(-180.927197004254,25.3273242564655,172.269015371745));
#95073=CARTESIAN_POINT('Ctrl Pts',(-174.736536607708,43.9896960337974,178.090041787821));
#95074=CARTESIAN_POINT('Ctrl Pts',(-169.732361483832,18.3274378186121,156.416018514887));
#95075=CARTESIAN_POINT('Ctrl Pts',(-180.322025264393,24.8627580474761,173.309162198402));
#95076=CARTESIAN_POINT('Ctrl Pts',(-173.607575117574,43.8719040042023,179.109193252876));
#95077=CARTESIAN_POINT('Ctrl Pts',(-169.558289763168,18.2203422570752,156.49864439362));
#95078=CARTESIAN_POINT('Ctrl Pts',(-180.021949930072,24.6347745292575,173.787216467402));
#95079=CARTESIAN_POINT('Ctrl Pts',(-173.071167892211,43.8119858594125,179.561393389303));
#95080=CARTESIAN_POINT('Ctrl Pts',(-169.20537587151,18.0054276813585,156.658881832012));
#95081=CARTESIAN_POINT('Ctrl Pts',(-179.433143561921,24.1912128908626,174.668691448684));
#95082=CARTESIAN_POINT('Ctrl Pts',(-172.061207809833,43.6907330173011,180.372779053295));
#95083=CARTESIAN_POINT('Ctrl Pts',(-169.026537105077,17.8976098204552,156.736496564402));
#95084=CARTESIAN_POINT('Ctrl Pts',(-179.144397687481,23.9756821774116,175.072075935675));
#95085=CARTESIAN_POINT('Ctrl Pts',(-171.586680536841,43.6293995460746,180.732834377098));
#95086=CARTESIAN_POINT('Ctrl Pts',(-168.48479752681,17.5743365828396,156.96321970107));
#95087=CARTESIAN_POINT('Ctrl Pts',(-178.29068744621,23.344281769509,176.201380676567));
#95088=CARTESIAN_POINT('Ctrl Pts',(-170.238369313117,43.4439993478709,181.715166341082));
#95089=CARTESIAN_POINT('Ctrl Pts',(-168.119950530228,17.3610377067902,157.104986914531));
#95090=CARTESIAN_POINT('Ctrl Pts',(-177.749090613288,22.951799353339,176.832994154249));
#95091=CARTESIAN_POINT('Ctrl Pts',(-169.445239878046,43.3196577793825,182.237721038455));
#95092=CARTESIAN_POINT('Ctrl Pts',(-167.391270115551,16.9433709217743,157.374360062321));
#95093=CARTESIAN_POINT('Ctrl Pts',(-176.699191958229,22.206366498613,177.96534356467));
#95094=CARTESIAN_POINT('Ctrl Pts',(-167.986743550946,43.0725588756287,183.147764868599));
#95095=CARTESIAN_POINT('Ctrl Pts',(-167.026606688627,16.7384994826158,157.502198040807));
#95096=CARTESIAN_POINT('Ctrl Pts',(-176.191279038635,21.8538198757381,178.463340366889));
#95097=CARTESIAN_POINT('Ctrl Pts',(-167.320397138975,42.9495163323862,183.534097905677));
#95098=CARTESIAN_POINT('Ctrl Pts',(-166.298120791151,16.3369438280935,157.747661911419));
#95099=CARTESIAN_POINT('Ctrl Pts',(-175.195015680742,21.1770552515635,179.377764246932));
#95100=CARTESIAN_POINT('Ctrl Pts',(-166.064733590356,42.7050918843688,184.228282962997));
#95101=CARTESIAN_POINT('Ctrl Pts',(-165.934275361887,16.1402438203051,157.865253806892));
#95102=CARTESIAN_POINT('Ctrl Pts',(-174.707713182136,20.8536655692418,179.792126024603));
#95103=CARTESIAN_POINT('Ctrl Pts',(-165.475999358049,42.5837015136963,184.535227655678));
#95104=CARTESIAN_POINT('Ctrl Pts',(-165.208022298475,15.7547762879034,158.092246123888));
#95105=CARTESIAN_POINT('Ctrl Pts',(-173.746828237938,20.229692948097,180.563630707583));
#95106=CARTESIAN_POINT('Ctrl Pts',(-164.350718159951,42.3428835648365,185.097515905741));
#95107=CARTESIAN_POINT('Ctrl Pts',(-164.845605266082,15.5660026353619,158.201632183931));
#95108=CARTESIAN_POINT('Ctrl Pts',(-173.273911339772,19.9296328625437,180.919710822024));
#95109=CARTESIAN_POINT('Ctrl Pts',(-163.81441996652,42.2234523785788,185.352529880529));
#95110=CARTESIAN_POINT('Ctrl Pts',(-163.760868033552,15.0109620114243,158.519528866614));
#95111=CARTESIAN_POINT('Ctrl Pts',(-171.867024170727,19.0559076974448,181.926432993042));
#95112=CARTESIAN_POINT('Ctrl Pts',(-162.261759601125,41.8683318500525,186.062918065107));
#95113=CARTESIAN_POINT('Ctrl Pts',(-163.041094616692,14.6559663241023,158.717878535442));
#95114=CARTESIAN_POINT('Ctrl Pts',(-170.954197690537,18.5147147268493,182.508909839269));
#95115=CARTESIAN_POINT('Ctrl Pts',(-161.300437601311,41.6358321593886,186.464837080218));
#95116=CARTESIAN_POINT('Ctrl Pts',(-161.608449841267,13.9724013655304,159.09418397859));
#95117=CARTESIAN_POINT('Ctrl Pts',(-169.153718088121,17.4887166685363,183.570253534368));
#95118=CARTESIAN_POINT('Ctrl Pts',(-159.461971844518,41.1797152854594,187.187814858497));
#95119=CARTESIAN_POINT('Ctrl Pts',(-160.895540391279,13.6438160922004,159.272068429678));
#95120=CARTESIAN_POINT('Ctrl Pts',(-168.268459650413,17.0057013714701,184.04599417238));
#95121=CARTESIAN_POINT('Ctrl Pts',(-158.585843562126,40.9560813261876,187.507754562274));
#95122=CARTESIAN_POINT('Ctrl Pts',(-159.475832904077,13.009713555937,159.61133763757));
#95123=CARTESIAN_POINT('Ctrl Pts',(-166.517450272312,16.0855401228304,184.923294929289));
#95124=CARTESIAN_POINT('Ctrl Pts',(-156.888768072043,40.5175628988981,188.093656406087));
#95125=CARTESIAN_POINT('Ctrl Pts',(-158.768161459745,12.7038561024453,159.772867963314));
#95126=CARTESIAN_POINT('Ctrl Pts',(-165.652176896289,15.6489979847093,185.323724854997));
#95127=CARTESIAN_POINT('Ctrl Pts',(-156.067224181849,40.30242287474,188.359519533784));
#95128=CARTESIAN_POINT('Ctrl Pts',(-157.366637414052,12.1159235889831,160.080243562044));
#95129=CARTESIAN_POINT('Ctrl Pts',(-163.948110086599,14.8191886550039,186.064138967974));
#95130=CARTESIAN_POINT('Ctrl Pts',(-154.472181220503,39.8831463972658,188.849648065907));
#95131=CARTESIAN_POINT('Ctrl Pts',(-156.671806181714,11.8333912668499,160.226325665881));
#95132=CARTESIAN_POINT('Ctrl Pts',(-163.109179654483,14.4259531767049,186.40392320471));
#95133=CARTESIAN_POINT('Ctrl Pts',(-153.697617035838,39.6786970852446,189.074223406174));
#95134=CARTESIAN_POINT('Ctrl Pts',(-154.602353948334,11.0153977851208,160.645385145478));
#95135=CARTESIAN_POINT('Ctrl Pts',(-160.617480990202,13.2962599683315,187.356762363426));
#95136=CARTESIAN_POINT('Ctrl Pts',(-151.424212839044,39.079703876623,189.702420218299));
#95137=CARTESIAN_POINT('Ctrl Pts',(-153.242645750871,10.5093218873485,160.899346226424));
#95138=CARTESIAN_POINT('Ctrl Pts',(-159.004438990581,12.616621750998,187.897831581203));
#95139=CARTESIAN_POINT('Ctrl Pts',(-149.974679379033,38.6994698247911,190.061332929028));
#95140=CARTESIAN_POINT('Ctrl Pts',(-150.552367945823,9.55775821321174,161.369122024951));
#95141=CARTESIAN_POINT('Ctrl Pts',(-155.83710947237,11.3572417479211,188.864442741271));
#95142=CARTESIAN_POINT('Ctrl Pts',(-147.153418928472,37.9718709822992,190.705208506625));
#95143=CARTESIAN_POINT('Ctrl Pts',(-149.221854956537,9.11237711894784,161.584828734122));
#95144=CARTESIAN_POINT('Ctrl Pts',(-154.286803188465,10.7798696037116,189.287290737056));
#95145=CARTESIAN_POINT('Ctrl Pts',(-145.782463563151,37.6245184723861,190.989493670861));
#95146=CARTESIAN_POINT('Ctrl Pts',(-146.582857115906,8.27040425016005,161.985922311379));
#95147=CARTESIAN_POINT('Ctrl Pts',(-151.233794084843,9.7025332564364,190.050527735751));
#95148=CARTESIAN_POINT('Ctrl Pts',(-143.091958400352,36.9585685878482,191.506211581955));
#95149=CARTESIAN_POINT('Ctrl Pts',(-145.274405011894,7.87386890592969,162.171263429212));
#95150=CARTESIAN_POINT('Ctrl Pts',(-149.733537694999,9.2038575210509,190.389647349539));
#95151=CARTESIAN_POINT('Ctrl Pts',(-141.77268701756,36.6399800572188,191.738407898794));
#95152=CARTESIAN_POINT('Ctrl Pts',(-142.67454674327,7.12121869547241,162.517120670501));
#95153=CARTESIAN_POINT('Ctrl Pts',(-146.772252351223,8.26827178830752,191.00646086707));
#95154=CARTESIAN_POINT('Ctrl Pts',(-139.169890034152,36.0282859548994,192.16423420799));
#95155=CARTESIAN_POINT('Ctrl Pts',(-141.383159986701,6.76513568801358,162.677614078792));
#95156=CARTESIAN_POINT('Ctrl Pts',(-145.312838364958,7.83212105280727,191.283481494081));
#95157=CARTESIAN_POINT('Ctrl Pts',(-137.886484698437,35.7351864115571,192.357764299665));
#95158=CARTESIAN_POINT('Ctrl Pts',(-137.52916857534,5.74824757347732,163.127966083129));
#95159=CARTESIAN_POINT('Ctrl Pts',(-140.977953290624,6.59772745373911,192.044692926872));
#95160=CARTESIAN_POINT('Ctrl Pts',(-134.074948396479,34.8901222694588,192.893480588533));
#95161=CARTESIAN_POINT('Ctrl Pts',(-134.986444518518,5.1383515380875,163.386981976694));
#95162=CARTESIAN_POINT('Ctrl Pts',(-138.162497251024,5.87806901503397,192.456640771667));
#95163=CARTESIAN_POINT('Ctrl Pts',(-131.584657294362,34.3722288222929,193.191471577095));
#95164=CARTESIAN_POINT('Ctrl Pts',(-129.935383900544,4.02085867614368,163.845181682642));
#95165=CARTESIAN_POINT('Ctrl Pts',(-132.620396885526,4.57771828187325,193.164571707407));
#95166=CARTESIAN_POINT('Ctrl Pts',(-126.659823795758,33.4111402621432,193.710740918262));
#95167=CARTESIAN_POINT('Ctrl Pts',(-127.424374444051,3.51309267049032,164.044346664358));
#95168=CARTESIAN_POINT('Ctrl Pts',(-129.895918979684,3.99874755408819,193.458855240834));
#95169=CARTESIAN_POINT('Ctrl Pts',(-124.223164579543,32.9676271892553,193.931671784718));
#95170=CARTESIAN_POINT('Ctrl Pts',(-122.457511674559,2.58424517009923,164.395361452057));
#95171=CARTESIAN_POINT('Ctrl Pts',(-124.546807846014,2.95145956830643,193.965517338237));
#95172=CARTESIAN_POINT('Ctrl Pts',(-119.413835209996,32.1484825663496,194.31696041224));
#95173=CARTESIAN_POINT('Ctrl Pts',(-119.997764986607,2.16231324461259,164.547549718778));
#95174=CARTESIAN_POINT('Ctrl Pts',(-121.920684619804,2.48302644750518,194.177754122744));
#95175=CARTESIAN_POINT('Ctrl Pts',(-117.037520550194,31.7720605896045,194.481596153228));
#95176=CARTESIAN_POINT('Ctrl Pts',(-115.113796886312,1.38623409901235,164.816743346736));
#95177=CARTESIAN_POINT('Ctrl Pts',(-116.737508908147,1.62907241709631,194.546134226495));
#95178=CARTESIAN_POINT('Ctrl Pts',(-112.323537492297,31.07452765352,194.770608310854));
#95179=CARTESIAN_POINT('Ctrl Pts',(-112.689642445873,1.03217190481425,164.933695702807));
#95180=CARTESIAN_POINT('Ctrl Pts',(-114.182223627302,1.24409699109422,194.701890597857));
#95181=CARTESIAN_POINT('Ctrl Pts',(-109.986006545736,30.7534547062723,194.89488035781));
#95182=CARTESIAN_POINT('Ctrl Pts',(-105.458748863613,0.0537109949632699,
165.243789332008));
#95183=CARTESIAN_POINT('Ctrl Pts',(-106.593713186433,0.187356491350593,
195.108680154073));
#95184=CARTESIAN_POINT('Ctrl Pts',(-103.014954688006,29.8608768518165,195.222527902486));
#95185=CARTESIAN_POINT('Ctrl Pts',(-100.692926996796,-0.487837340122015,
165.396788055826));
#95186=CARTESIAN_POINT('Ctrl Pts',(-101.648242750641,-0.385696025224757,
195.2997496196));
#95187=CARTESIAN_POINT('Ctrl Pts',(-98.4220441742718,29.3594587157306,195.381539694843));
#95188=CARTESIAN_POINT('Ctrl Pts',(-91.2328687780407,-1.41275722738798,
165.637152647262));
#95189=CARTESIAN_POINT('Ctrl Pts',(-91.8896160224937,-1.35729231567298,
195.595521040211));
#95190=CARTESIAN_POINT('Ctrl Pts',(-89.2957519395693,28.4971764608672,195.630229860082));
#95191=CARTESIAN_POINT('Ctrl Pts',(-86.5390573445431,-1.79556727823837,
165.724146017721));
#95192=CARTESIAN_POINT('Ctrl Pts',(-87.0809543903837,-1.7543127179252,195.699017410214));
#95193=CARTESIAN_POINT('Ctrl Pts',(-84.7630722941598,28.1366238331763,195.719348296838));
#95194=CARTESIAN_POINT('Ctrl Pts',(-77.2034000845379,-2.44180831978024,
165.856868653474));
#95195=CARTESIAN_POINT('Ctrl Pts',(-77.5561948922658,-2.42113102767928,
195.855280888841));
#95196=CARTESIAN_POINT('Ctrl Pts',(-75.7339440753839,27.524859474872,195.854930954148));
#95197=CARTESIAN_POINT('Ctrl Pts',(-72.5617270997191,-2.70499078515223,
165.902429251621));
#95198=CARTESIAN_POINT('Ctrl Pts',(-72.8420539091534,-2.69036081274705,
195.90761787253));
#95199=CARTESIAN_POINT('Ctrl Pts',(-71.2377602240549,27.2738023676749,195.901170564023));
#95200=CARTESIAN_POINT('Ctrl Pts',(-63.3192368021652,-3.13951331323087,
165.968086174843));
#95201=CARTESIAN_POINT('Ctrl Pts',(-63.4824566004367,-3.13329077685642,
195.982573684347));
#95202=CARTESIAN_POINT('Ctrl Pts',(-62.2685467898851,26.8576621150016,195.967694278259));
#95203=CARTESIAN_POINT('Ctrl Pts',(-58.7184924969416,-3.31072222891366,
165.988096029799));
#95204=CARTESIAN_POINT('Ctrl Pts',(-58.8378802767016,-3.30674675640559,
196.005013040848));
#95205=CARTESIAN_POINT('Ctrl Pts',(-57.7956329921226,26.6926696350143,195.987872556486));
#95206=CARTESIAN_POINT('Ctrl Pts',(-44.9687962503876,-3.71864843947255,
166.025958285563));
#95207=CARTESIAN_POINT('Ctrl Pts',(-44.9856197745133,-3.71901632940911,
196.04750598918));
#95208=CARTESIAN_POINT('Ctrl Pts',(-44.4000239059869,26.2982864331341,196.026023260468));
#95209=CARTESIAN_POINT('Ctrl Pts',(-35.8704264307398,-3.84988321153493,
166.022565415402));
#95210=CARTESIAN_POINT('Ctrl Pts',(-35.8586554592819,-3.85007352565092,
196.043873063051));
#95211=CARTESIAN_POINT('Ctrl Pts',(-35.4996912577566,26.1694752614148,196.022557099425));
#95212=CARTESIAN_POINT('Ctrl Pts',(-17.7576320506981,-3.97366628546334,
166.00984699518));
#95213=CARTESIAN_POINT('Ctrl Pts',(-17.7264703415601,-3.97376872241134,
196.031052872576));
#95214=CARTESIAN_POINT('Ctrl Pts',(-17.6760420909501,26.0478005878471,196.009824900738));
#95215=CARTESIAN_POINT('Ctrl Pts',(-8.74333296613901,-3.96249962263878,
165.999882631878));
#95216=CARTESIAN_POINT('Ctrl Pts',(-8.72284852848699,-3.96249840284406,
196.020999546301));
#95217=CARTESIAN_POINT('Ctrl Pts',(-8.75350004691697,26.0586067043184,195.999875379291));
#95218=CARTESIAN_POINT('Ctrl Pts',(0.15743830809244,-3.96262988886149,166.00000104579));
#95219=CARTESIAN_POINT('Ctrl Pts',(0.157070562002837,-3.96262989972655,
196.021119017258));
#95220=CARTESIAN_POINT('Ctrl Pts',(0.157610541791236,26.0584806777796,195.999993616651));
#95221=CARTESIAN_POINT('',(1.578508351368E-14,26.0373712544753,196.));
#95222=CARTESIAN_POINT('Origin',(4.15733729152917E-15,26.0373712544753,
166.));
#95223=CARTESIAN_POINT('Ctrl Pts',(-190.499797482064,51.8013867006572,102.335336081498));
#95224=CARTESIAN_POINT('Ctrl Pts',(-190.499797482064,51.7796732650764,102.335336081498));
#95225=CARTESIAN_POINT('Ctrl Pts',(-190.499735682025,51.7624009619146,102.352155239618));
#95226=CARTESIAN_POINT('Ctrl Pts',(-190.499673388249,51.7493947125939,102.369009004064));
#95227=CARTESIAN_POINT('Ctrl Pts',(-190.499611094472,51.7363884632733,102.38586276851));
#95228=CARTESIAN_POINT('Ctrl Pts',(-190.499541046104,51.7261944008059,102.404734768362));
#95229=CARTESIAN_POINT('Ctrl Pts',(-190.499469961948,51.7170974306138,102.423784057877));
#95230=CARTESIAN_POINT('Ctrl Pts',(-190.499327793636,51.6989034902297,102.461882636908));
#95231=CARTESIAN_POINT('Ctrl Pts',(-190.499176806309,51.684877084871,102.50195510353));
#95232=CARTESIAN_POINT('Ctrl Pts',(-190.499023050416,51.6721578498453,102.542322989557));
#95233=CARTESIAN_POINT('Ctrl Pts',(-190.498715538629,51.6467193797941,102.62305876161));
#95234=CARTESIAN_POINT('Ctrl Pts',(-190.498396552736,51.627122398088,102.70511271305));
#95235=CARTESIAN_POINT('Ctrl Pts',(-190.498069248062,51.6091555610353,102.78753449951));
#95236=CARTESIAN_POINT('Ctrl Pts',(-190.497414638714,51.5732218869298,102.95237807243));
#95237=CARTESIAN_POINT('Ctrl Pts',(-190.496725517573,51.5447751841326,103.119010291625));
#95238=CARTESIAN_POINT('Ctrl Pts',(-190.496006633022,51.5184793922393,103.285777971499));
#95239=CARTESIAN_POINT('Ctrl Pts',(-190.49456886392,51.4658878084526,103.619313331245));
#95240=CARTESIAN_POINT('Ctrl Pts',(-190.493009667524,51.4229821624655,103.954070779999));
#95241=CARTESIAN_POINT('Ctrl Pts',(-190.491322220494,51.3825621856073,104.2891413603));
#95242=CARTESIAN_POINT('Ctrl Pts',(-190.488159741497,51.30681028015,104.917103989015));
#95243=CARTESIAN_POINT('Ctrl Pts',(-190.484546269356,51.2411823737622,105.546379733642));
#95244=CARTESIAN_POINT('Ctrl Pts',(-190.480418712091,51.178146335177,106.175836802634));
#95245=CARTESIAN_POINT('Ctrl Pts',(-190.480141475362,51.1739123769095,106.218115711987));
#95246=CARTESIAN_POINT('Ctrl Pts',(-190.479861919642,51.1696901117017,106.260395458915));
#95247=CARTESIAN_POINT('Ctrl Pts',(-190.479580025962,51.1654772571583,106.302675708929));
#95248=CARTESIAN_POINT('Ctrl Pts',(-190.47255445146,51.0604812053327,107.356417127231));
#95249=CARTESIAN_POINT('Ctrl Pts',(-190.46407790808,50.9625995955066,108.41079436899));
#95250=CARTESIAN_POINT('Ctrl Pts',(-190.453802680175,50.8668358069772,109.465349178475));
#95251=CARTESIAN_POINT('Ctrl Pts',(-190.450977048573,50.8405012877136,109.755345996389));
#95252=CARTESIAN_POINT('Ctrl Pts',(-190.44801515712,50.8143269223293,110.045356058084));
#95253=CARTESIAN_POINT('Ctrl Pts',(-190.444909217821,50.7882088029142,110.335369415777));
#95254=CARTESIAN_POINT('Ctrl Pts',(-190.435051162092,50.7053115367744,111.255853548446));
#95255=CARTESIAN_POINT('Ctrl Pts',(-190.423743516833,50.6233182006791,112.176446285769));
#95256=CARTESIAN_POINT('Ctrl Pts',(-190.410714850994,50.5421480526697,113.097071442683));
#95257=CARTESIAN_POINT('Ctrl Pts',(-190.397868218425,50.4621119937211,114.004833854546));
#95258=CARTESIAN_POINT('Ctrl Pts',(-190.383348467128,50.3828762807955,114.912627713187));
#95259=CARTESIAN_POINT('Ctrl Pts',(-190.366864774591,50.304363509189,115.820340176612));
#95260=CARTESIAN_POINT('Ctrl Pts',(-190.351225118062,50.2298709294274,116.681573854888));
#95261=CARTESIAN_POINT('Ctrl Pts',(-190.333817436516,50.1560291510364,117.542733975473));
#95262=CARTESIAN_POINT('Ctrl Pts',(-190.314365284359,50.0827720612279,118.403691037767));
#95263=CARTESIAN_POINT('Ctrl Pts',(-190.295448100247,50.0115296689136,119.240970282112));
#95264=CARTESIAN_POINT('Ctrl Pts',(-190.274596728903,49.9411985013373,120.078097715621));
#95265=CARTESIAN_POINT('Ctrl Pts',(-190.251524715879,49.8714851641544,120.91505355053));
#95266=CARTESIAN_POINT('Ctrl Pts',(-190.228651418363,49.8023722566437,121.744800820508));
#95267=CARTESIAN_POINT('Ctrl Pts',(-190.203595741332,49.7338665828117,122.574379401192));
#95268=CARTESIAN_POINT('Ctrl Pts',(-190.176046929657,49.665682264082,123.403729980441));
#95269=CARTESIAN_POINT('Ctrl Pts',(-190.148846990024,49.598361416445,124.222577847862));
#95270=CARTESIAN_POINT('Ctrl Pts',(-190.119216815711,49.5313538363069,125.041203389024));
#95271=CARTESIAN_POINT('Ctrl Pts',(-190.086823927838,49.4643843690408,125.859511081624));
#95272=CARTESIAN_POINT('Ctrl Pts',(-190.078849634445,49.4478982137334,126.060957326609));
#95273=CARTESIAN_POINT('Ctrl Pts',(-190.070707749289,49.4314143681323,126.262384127506));
#95274=CARTESIAN_POINT('Ctrl Pts',(-190.062392979207,49.4149287273199,126.463789702368));
#95275=CARTESIAN_POINT('Ctrl Pts',(-190.030547811375,49.3517895192197,127.235163326751));
#95276=CARTESIAN_POINT('Ctrl Pts',(-189.996170659515,49.2883645194752,128.006194734142));
#95277=CARTESIAN_POINT('Ctrl Pts',(-189.958940677373,49.2243050437096,128.776856652747));
#95278=CARTESIAN_POINT('Ctrl Pts',(-189.922052547442,49.1608337732603,129.540442218756));
#95279=CARTESIAN_POINT('Ctrl Pts',(-189.882363909103,49.0967396250354,130.303665012026));
#95280=CARTESIAN_POINT('Ctrl Pts',(-189.839528747592,49.031683431776,131.066460714902));
#95281=CARTESIAN_POINT('Ctrl Pts',(-189.797307015648,48.9675588888477,131.818332648131));
#95282=CARTESIAN_POINT('Ctrl Pts',(-189.752028378616,48.902499657906,132.569789563874));
#95283=CARTESIAN_POINT('Ctrl Pts',(-189.703326084319,48.8361809353554,133.320733846737));
#95284=CARTESIAN_POINT('Ctrl Pts',(-189.677789514313,48.8014073640976,133.714484111013));
#95285=CARTESIAN_POINT('Ctrl Pts',(-189.651311065098,48.7662875174997,134.108092840235));
#95286=CARTESIAN_POINT('Ctrl Pts',(-189.623833678354,48.7307745724516,134.50154201427));
#95287=CARTESIAN_POINT('Ctrl Pts',(-189.575579238559,48.6684084790239,135.19249816881));
#95288=CARTESIAN_POINT('Ctrl Pts',(-189.524246833971,48.6048542762143,135.882953961284));
#95289=CARTESIAN_POINT('Ctrl Pts',(-189.46949371259,48.540048518188,136.572913023358));
#95290=CARTESIAN_POINT('Ctrl Pts',(-189.415263393029,48.4758615480475,137.256284116672));
#95291=CARTESIAN_POINT('Ctrl Pts',(-189.357677536326,48.4104468091526,137.939167882345));
#95292=CARTESIAN_POINT('Ctrl Pts',(-189.2963680754,48.3437426557793,138.62153151236));
#95293=CARTESIAN_POINT('Ctrl Pts',(-189.236051587727,48.2781188485588,139.29284352287));
#95294=CARTESIAN_POINT('Ctrl Pts',(-189.172131261117,48.211247055563,139.963652031237));
#95295=CARTESIAN_POINT('Ctrl Pts',(-189.104220443876,48.1430685780765,140.633891378944));
#95296=CARTESIAN_POINT('Ctrl Pts',(-189.041196215209,48.0797959489164,141.255903005771));
#95297=CARTESIAN_POINT('Ctrl Pts',(-188.974734906569,48.01539791719,141.877424101301));
#95298=CARTESIAN_POINT('Ctrl Pts',(-188.90449721651,47.9498275654531,142.498375722798));
#95299=CARTESIAN_POINT('Ctrl Pts',(-188.834812474735,47.8847734182416,143.114438884366));
#95300=CARTESIAN_POINT('Ctrl Pts',(-188.761413027888,47.8185580207201,143.729925662549));
#95301=CARTESIAN_POINT('Ctrl Pts',(-188.683920571469,47.7512472696655,144.344853949472));
#95302=CARTESIAN_POINT('Ctrl Pts',(-188.607758227294,47.6850918678956,144.949227355559));
#95303=CARTESIAN_POINT('Ctrl Pts',(-188.527642294694,47.6178783920758,145.553061198004));
#95304=CARTESIAN_POINT('Ctrl Pts',(-188.443176958487,47.5496694036548,146.156338077234));
#95305=CARTESIAN_POINT('Ctrl Pts',(-188.359576961453,47.4821592097015,146.753434443376));
#95306=CARTESIAN_POINT('Ctrl Pts',(-188.271716386634,47.41367379652,147.349985158678));
#95307=CARTESIAN_POINT('Ctrl Pts',(-188.179173084183,47.3442738223829,147.945940209406));
#95308=CARTESIAN_POINT('Ctrl Pts',(-188.088056539572,47.275943800955,148.532707306839));
#95309=CARTESIAN_POINT('Ctrl Pts',(-187.992400672799,47.206727201113,149.118896894521));
#95310=CARTESIAN_POINT('Ctrl Pts',(-187.891763054282,47.1366819186201,149.704429809714));
#95311=CARTESIAN_POINT('Ctrl Pts',(-187.849814782888,47.1074852964908,149.948494544136));
#95312=CARTESIAN_POINT('Ctrl Pts',(-187.807000477934,47.078144696512,150.192444812282));
#95313=CARTESIAN_POINT('Ctrl Pts',(-187.763285937964,47.0486643115202,150.436273275158));
#95314=CARTESIAN_POINT('Ctrl Pts',(-187.667271248349,46.9839135440019,150.971818523922));
#95315=CARTESIAN_POINT('Ctrl Pts',(-187.566920476803,46.9184686150377,151.506755633221));
#95316=CARTESIAN_POINT('Ctrl Pts',(-187.461823165435,46.8524910947455,152.041113281851));
#95317=CARTESIAN_POINT('Ctrl Pts',(-187.358729974763,46.7877717123848,152.565281162455));
#95318=CARTESIAN_POINT('Ctrl Pts',(-187.251069644819,46.7225398571991,153.08889138662));
#95319=CARTESIAN_POINT('Ctrl Pts',(-187.138416624462,46.6569480314088,153.611939038436));
#95320=CARTESIAN_POINT('Ctrl Pts',(-187.026967315194,46.5920570621758,154.129397863105));
#95321=CARTESIAN_POINT('Ctrl Pts',(-186.910631597444,46.5268137738982,154.646306033395));
#95322=CARTESIAN_POINT('Ctrl Pts',(-186.788957749885,46.4613658323308,155.162628032045));
#95323=CARTESIAN_POINT('Ctrl Pts',(-186.665654696768,46.3950415467317,155.685863551444));
#95324=CARTESIAN_POINT('Ctrl Pts',(-186.536869956916,46.3285070905597,156.208497179867));
#95325=CARTESIAN_POINT('Ctrl Pts',(-186.402088378624,46.2619161410564,156.730459690725));
#95326=CARTESIAN_POINT('Ctrl Pts',(-186.267306800331,46.1953251915531,157.252422201583));
#95327=CARTESIAN_POINT('Ctrl Pts',(-186.126528666188,46.1286777487184,157.773713602935));
#95328=CARTESIAN_POINT('Ctrl Pts',(-185.979189427949,46.0621274897938,158.294232035195));
#95329=CARTESIAN_POINT('Ctrl Pts',(-185.8628900334,46.0095973225925,158.705093250761));
#95330=CARTESIAN_POINT('Ctrl Pts',(-185.742356438997,45.957106091155,159.115969231144));
#95331=CARTESIAN_POINT('Ctrl Pts',(-185.617482356425,45.9048666497495,159.526097415001));
#95332=CARTESIAN_POINT('Ctrl Pts',(-185.493615974712,45.8530487668366,159.932915972755));
#95333=CARTESIAN_POINT('Ctrl Pts',(-185.365478696385,45.8014786265943,160.338998741735));
#95334=CARTESIAN_POINT('Ctrl Pts',(-185.232986637722,45.7503639717296,160.743648602471));
#95335=CARTESIAN_POINT('Ctrl Pts',(-185.101749884476,45.6997336062917,161.14446457937));
#95336=CARTESIAN_POINT('Ctrl Pts',(-184.966240317941,45.649550136062,161.54387469968));
#95337=CARTESIAN_POINT('Ctrl Pts',(-184.826398490639,45.6000154546973,161.941247763602));
#95338=CARTESIAN_POINT('Ctrl Pts',(-184.79886466275,45.5902624400408,162.019487599001));
#95339=CARTESIAN_POINT('Ctrl Pts',(-184.771162960822,45.5805345767976,162.097648608569));
#95340=CARTESIAN_POINT('Ctrl Pts',(-184.743293041545,45.5708334059981,162.175726186804));
#95341=CARTESIAN_POINT('Ctrl Pts',(-184.536768932763,45.4989449432585,162.754303472959));
#95342=CARTESIAN_POINT('Ctrl Pts',(-184.320853286713,45.4284747155974,163.32874495722));
#95343=CARTESIAN_POINT('Ctrl Pts',(-184.094786606929,45.3598039129179,163.898733974326));
#95344=CARTESIAN_POINT('Ctrl Pts',(-183.872083263143,45.2921547689052,164.460242906788));
#95345=CARTESIAN_POINT('Ctrl Pts',(-183.639528757453,45.2262519058143,165.017430797686));
#95346=CARTESIAN_POINT('Ctrl Pts',(-183.39634647974,45.1624597518103,165.569990148998));
#95347=CARTESIAN_POINT('Ctrl Pts',(-183.340871979055,45.1479075487293,165.696039441739));
#95348=CARTESIAN_POINT('Ctrl Pts',(-183.28484421427,45.1334651833255,165.821847855984));
#95349=CARTESIAN_POINT('Ctrl Pts',(-183.228253584138,45.119136981697,165.947411712232));
#95350=CARTESIAN_POINT('Ctrl Pts',(-182.974553425451,45.0549025489239,166.510324162243));
#95351=CARTESIAN_POINT('Ctrl Pts',(-182.709541404531,44.9930065159401,167.068328533397));
#95352=CARTESIAN_POINT('Ctrl Pts',(-182.432350626818,44.9336063856646,167.621026623286));
#95353=CARTESIAN_POINT('Ctrl Pts',(-182.158590221301,44.8749413612142,168.166884802498));
#95354=CARTESIAN_POINT('Ctrl Pts',(-181.872950676918,44.8187108456795,168.707567162311));
#95355=CARTESIAN_POINT('Ctrl Pts',(-181.57454641481,44.7650665665191,169.242697316412));
#95356=CARTESIAN_POINT('Ctrl Pts',(-181.512347374015,44.7538850147397,169.354239229556));
#95357=CARTESIAN_POINT('Ctrl Pts',(-181.449593569415,44.7428158265347,169.465539944495));
#95358=CARTESIAN_POINT('Ctrl Pts',(-181.386276697259,44.7318603759468,169.576596096675));
#95359=CARTESIAN_POINT('Ctrl Pts',(-181.227234179103,44.7043419217072,169.855552550111));
#95360=CARTESIAN_POINT('Ctrl Pts',(-181.064463358344,44.6775394846246,170.133265862419));
#95361=CARTESIAN_POINT('Ctrl Pts',(-180.898096995233,44.6514228089558,170.409215846077));
#95362=CARTESIAN_POINT('Ctrl Pts',(-180.733096332856,44.6255205249614,170.682900557546));
#95363=CARTESIAN_POINT('Ctrl Pts',(-180.56455880916,44.6002927897678,170.954850835475));
#95364=CARTESIAN_POINT('Ctrl Pts',(-180.392647465491,44.5757100866394,171.224598059603));
#95365=CARTESIAN_POINT('Ctrl Pts',(-180.221339873901,44.5512137178845,171.493397932356));
#95366=CARTESIAN_POINT('Ctrl Pts',(-180.046682003667,44.5273578584496,171.760010253265));
#95367=CARTESIAN_POINT('Ctrl Pts',(-179.868870312727,44.5041133014966,172.024009230221));
#95368=CARTESIAN_POINT('Ctrl Pts',(-179.691626830169,44.4809430239796,172.287164581929));
#95369=CARTESIAN_POINT('Ctrl Pts',(-179.511249554796,44.4583801482762,172.547723337867));
#95370=CARTESIAN_POINT('Ctrl Pts',(-179.327969613584,44.4363957466509,172.805300555097));
#95371=CARTESIAN_POINT('Ctrl Pts',(-179.276482988262,44.4302199336191,172.877658618873));
#95372=CARTESIAN_POINT('Ctrl Pts',(-179.224767526064,44.4240897708081,172.949781614421));
#95373=CARTESIAN_POINT('Ctrl Pts',(-179.172828887012,44.4180046169303,173.021661519505));
#95374=CARTESIAN_POINT('Ctrl Pts',(-178.870046992592,44.3825305565271,173.440693173579));
#95375=CARTESIAN_POINT('Ctrl Pts',(-178.559161603634,44.3484774483554,173.852176021675));
#95376=CARTESIAN_POINT('Ctrl Pts',(-178.240147844902,44.315127964356,174.256013723285));
#95377=CARTESIAN_POINT('Ctrl Pts',(-177.922397125579,44.2819105176478,174.658252550493));
#95378=CARTESIAN_POINT('Ctrl Pts',(-177.596582140635,44.249391134563,175.052906781522));
#95379=CARTESIAN_POINT('Ctrl Pts',(-177.262717453059,44.2168609734906,175.439914913192));
#95380=CARTESIAN_POINT('Ctrl Pts',(-177.050436010064,44.1961772959701,175.685986593424));
#95381=CARTESIAN_POINT('Ctrl Pts',(-176.83490101927,44.1754892611164,175.928967772909));
#95382=CARTESIAN_POINT('Ctrl Pts',(-176.616124869558,44.154614658246,176.168849396935));
#95383=CARTESIAN_POINT('Ctrl Pts',(-176.272384001883,44.1218165030885,176.545751164748));
#95384=CARTESIAN_POINT('Ctrl Pts',(-175.920645070288,44.0884963485789,176.914993814555));
#95385=CARTESIAN_POINT('Ctrl Pts',(-175.560988485832,44.0537660832848,177.276571067712));
#95386=CARTESIAN_POINT('Ctrl Pts',(-175.202561092196,44.0191545148952,177.636912565821));
#95387=CARTESIAN_POINT('Ctrl Pts',(-174.836269971456,43.9831424578628,177.98964110849));
#95388=CARTESIAN_POINT('Ctrl Pts',(-174.462238176354,43.9448508755096,178.334778513058));
#95389=CARTESIAN_POINT('Ctrl Pts',(-174.219851918052,43.9200365322034,178.558440151425));
#95390=CARTESIAN_POINT('Ctrl Pts',(-173.97421583996,43.8942648992402,178.778914445244));
#95391=CARTESIAN_POINT('Ctrl Pts',(-173.725373524941,43.8672967522522,178.996213246504));
#95392=CARTESIAN_POINT('Ctrl Pts',(-173.33157436528,43.8246189881401,179.340094010213));
#95393=CARTESIAN_POINT('Ctrl Pts',(-172.929740164485,43.77893904078,179.676023922631));
#95394=CARTESIAN_POINT('Ctrl Pts',(-172.520054883594,43.7294367759111,180.004094210126));
#95395=CARTESIAN_POINT('Ctrl Pts',(-172.400129907369,43.7149462432647,180.100128466817));
#95396=CARTESIAN_POINT('Ctrl Pts',(-172.279532495907,43.7001281849663,180.195489398804));
#95397=CARTESIAN_POINT('Ctrl Pts',(-172.158268028556,43.6849620296658,180.290179656169));
#95398=CARTESIAN_POINT('Ctrl Pts',(-171.937519087759,43.6573536725623,180.462553101367));
#95399=CARTESIAN_POINT('Ctrl Pts',(-171.714272716709,43.6285444230998,180.632922956221));
#95400=CARTESIAN_POINT('Ctrl Pts',(-171.48897075388,43.5985086299391,180.800987948655));
#95401=CARTESIAN_POINT('Ctrl Pts',(-171.263429988966,43.5684410012367,180.969231076556));
#95402=CARTESIAN_POINT('Ctrl Pts',(-171.035829220323,43.5371442273815,181.135164528807));
#95403=CARTESIAN_POINT('Ctrl Pts',(-170.806655279466,43.5045925753827,181.29851498135));
#95404=CARTESIAN_POINT('Ctrl Pts',(-170.709384854195,43.4907763752452,181.367847331824));
#95405=CARTESIAN_POINT('Ctrl Pts',(-170.611831564477,43.4767341104252,181.436714707051));
#95406=CARTESIAN_POINT('Ctrl Pts',(-170.514035031329,43.462463813322,181.505097724209));
#95407=CARTESIAN_POINT('Ctrl Pts',(-170.078760309056,43.3989492959011,181.809458194294));
#95408=CARTESIAN_POINT('Ctrl Pts',(-169.639517762154,43.3309925285366,182.103636987488));
#95409=CARTESIAN_POINT('Ctrl Pts',(-169.196641938417,43.2586019347472,182.388337219161));
#95410=CARTESIAN_POINT('Ctrl Pts',(-168.747439482107,43.1851772165732,182.677104490991));
#95411=CARTESIAN_POINT('Ctrl Pts',(-168.294499348488,43.1071910897059,182.956120347362));
#95412=CARTESIAN_POINT('Ctrl Pts',(-167.838152191216,43.024652343844,183.226067938466));
#95413=CARTESIAN_POINT('Ctrl Pts',(-167.590085918936,42.9797850127379,183.372809057742));
#95414=CARTESIAN_POINT('Ctrl Pts',(-167.341012569015,42.9335724221927,183.51686972133));
#95415=CARTESIAN_POINT('Ctrl Pts',(-167.090982792996,42.8860159840665,183.658353716968));
#95416=CARTESIAN_POINT('Ctrl Pts',(-166.642612966349,42.8007346537463,183.912072116462));
#95417=CARTESIAN_POINT('Ctrl Pts',(-166.191155107318,42.7111080633194,184.157515138959));
#95418=CARTESIAN_POINT('Ctrl Pts',(-165.736825918976,42.6175507757671,184.39527710363));
#95419=CARTESIAN_POINT('Ctrl Pts',(-165.260941198057,42.5195546865456,184.644319624132));
#95420=CARTESIAN_POINT('Ctrl Pts',(-164.781906536675,42.4172460703372,184.884935082214));
#95421=CARTESIAN_POINT('Ctrl Pts',(-164.299938036989,42.3111013404516,185.117755861939));
#95422=CARTESIAN_POINT('Ctrl Pts',(-163.829408878122,42.207475915753,185.345050728144));
#95423=CARTESIAN_POINT('Ctrl Pts',(-163.356083415661,42.1001943137969,185.564916129514));
#95424=CARTESIAN_POINT('Ctrl Pts',(-162.880130934807,41.9896998241888,185.777896291562));
#95425=CARTESIAN_POINT('Ctrl Pts',(-162.386821667856,41.8751758793343,185.998643302748));
#95426=CARTESIAN_POINT('Ctrl Pts',(-161.890690542258,41.7572004422704,186.211993785727));
#95427=CARTESIAN_POINT('Ctrl Pts',(-161.391889708809,41.6362670896229,186.418507804901));
#95428=CARTESIAN_POINT('Ctrl Pts',(-160.893088875361,41.5153337369753,186.625021824075));
#95429=CARTESIAN_POINT('Ctrl Pts',(-160.391618367242,41.3914424687442,186.824699157984));
#95430=CARTESIAN_POINT('Ctrl Pts',(-159.887592775519,41.2650868615552,187.018056568477));
#95431=CARTESIAN_POINT('Ctrl Pts',(-159.229965927336,41.1002245191058,187.270339441655));
#95432=CARTESIAN_POINT('Ctrl Pts',(-158.567639773076,40.9312012789215,187.511993851814));
#95433=CARTESIAN_POINT('Ctrl Pts',(-157.901479365142,40.7592717923683,187.743807501735));
#95434=CARTESIAN_POINT('Ctrl Pts',(-157.317622400269,40.6085840195801,187.946980810216));
#95435=CARTESIAN_POINT('Ctrl Pts',(-156.730820322625,40.4556637660405,188.142593890958));
#95436=CARTESIAN_POINT('Ctrl Pts',(-156.141659320346,40.3013557385819,188.331144415625));
#95437=CARTESIAN_POINT('Ctrl Pts',(-155.654196713949,40.173683688052,188.487148173234));
#95438=CARTESIAN_POINT('Ctrl Pts',(-155.165963645099,40.0452972553808,188.638049161514));
#95439=CARTESIAN_POINT('Ctrl Pts',(-154.676990185282,39.9164969873809,188.784249754084));
#95440=CARTESIAN_POINT('Ctrl Pts',(-154.183078283921,39.7863958868276,188.93192691571));
#95441=CARTESIAN_POINT('Ctrl Pts',(-153.68841100885,39.6558725495822,189.074808137655));
#95442=CARTESIAN_POINT('Ctrl Pts',(-153.192977621197,39.5252367209535,189.213274927384));
#95443=CARTESIAN_POINT('Ctrl Pts',(-152.909710400687,39.4505448471376,189.29244420349));
#95444=CARTESIAN_POINT('Ctrl Pts',(-152.626191966415,39.3758161992806,189.370169781213));
#95445=CARTESIAN_POINT('Ctrl Pts',(-152.342414195266,39.3011086719599,189.446518398969));
#95446=CARTESIAN_POINT('Ctrl Pts',(-151.795151060383,39.1570358101738,189.593756090377));
#95447=CARTESIAN_POINT('Ctrl Pts',(-151.246876778824,39.0130961115111,189.735887647354));
#95448=CARTESIAN_POINT('Ctrl Pts',(-150.697673775629,38.8695161945702,189.873312967304));
#95449=CARTESIAN_POINT('Ctrl Pts',(-150.142368814188,38.7243410229547,190.012265160849));
#95450=CARTESIAN_POINT('Ctrl Pts',(-149.58611444304,38.5795336722339,190.146405843213));
#95451=CARTESIAN_POINT('Ctrl Pts',(-149.028954080029,38.4353283988271,190.276115113943));
#95452=CARTESIAN_POINT('Ctrl Pts',(-148.4684247408,38.290251160778,190.406608696474));
#95453=CARTESIAN_POINT('Ctrl Pts',(-147.906978444276,38.1457833032065,190.532616977839));
#95454=CARTESIAN_POINT('Ctrl Pts',(-147.344616727764,38.0021633577065,190.654495450789));
#95455=CARTESIAN_POINT('Ctrl Pts',(-146.777274095274,37.8572713503638,190.777453418333));
#95456=CARTESIAN_POINT('Ctrl Pts',(-146.208999795835,37.713242341761,190.896207979983));
#95457=CARTESIAN_POINT('Ctrl Pts',(-145.639751585534,37.5703212579178,191.011094050046));
#95458=CARTESIAN_POINT('Ctrl Pts',(-145.311331144991,37.4878647750177,191.077376091973));
#95459=CARTESIAN_POINT('Ctrl Pts',(-144.982585719152,37.4057770720487,191.142369935152));
#95460=CARTESIAN_POINT('Ctrl Pts',(-144.653500579793,37.3241051839344,191.206135628088));
#95461=CARTESIAN_POINT('Ctrl Pts',(-144.007827757714,37.1638630089583,191.331245424873));
#95462=CARTESIAN_POINT('Ctrl Pts',(-143.360891396152,37.0051772754077,191.451621044132));
#95463=CARTESIAN_POINT('Ctrl Pts',(-142.712787463218,36.8481764161634,191.567642104075));
#95464=CARTESIAN_POINT('Ctrl Pts',(-142.066595888332,36.6916388188152,191.683320821074));
#95465=CARTESIAN_POINT('Ctrl Pts',(-141.419243589998,36.5367761673373,191.79467045464));
#95466=CARTESIAN_POINT('Ctrl Pts',(-140.770782326781,36.3837157610625,191.902036140484));
#95467=CARTESIAN_POINT('Ctrl Pts',(-140.116576423578,36.2292994111407,192.010352965966));
#95468=CARTESIAN_POINT('Ctrl Pts',(-139.461241868626,36.0767173796067,192.114614827941));
#95469=CARTESIAN_POINT('Ctrl Pts',(-138.804787361359,35.9261003790415,192.215146561305));
#95470=CARTESIAN_POINT('Ctrl Pts',(-138.154084610909,35.7768030622473,192.314797450565));
#95471=CARTESIAN_POINT('Ctrl Pts',(-137.502281364437,35.6294364926588,192.410783106841));
#95472=CARTESIAN_POINT('Ctrl Pts',(-136.849343077584,35.4841279770207,192.50339336493));
#95473=CARTESIAN_POINT('Ctrl Pts',(-136.122601282649,35.3223948184655,192.606471629062));
#95474=CARTESIAN_POINT('Ctrl Pts',(-135.394479734399,35.1631836595734,192.705364347868));
#95475=CARTESIAN_POINT('Ctrl Pts',(-134.665082037698,35.0065278137277,192.800411184564));
#95476=CARTESIAN_POINT('Ctrl Pts',(-133.932046814869,34.8490907209231,192.895932022416));
#95477=CARTESIAN_POINT('Ctrl Pts',(-133.197722710275,34.6942344915477,192.987568389549));
#95478=CARTESIAN_POINT('Ctrl Pts',(-132.462170600657,34.5419929398785,193.075636120954));
#95479=CARTESIAN_POINT('Ctrl Pts',(-131.721209520432,34.3886318617104,193.164351468979));
#95480=CARTESIAN_POINT('Ctrl Pts',(-130.979002347912,34.2379240573311,193.249445386225));
#95481=CARTESIAN_POINT('Ctrl Pts',(-130.235565957058,34.0899040924884,193.331213319885));
#95482=CARTESIAN_POINT('Ctrl Pts',(-129.804514902801,34.0040807958603,193.378623097564));
#95483=CARTESIAN_POINT('Ctrl Pts',(-129.373049766394,33.9191610927974,193.424914252193));
#95484=CARTESIAN_POINT('Ctrl Pts',(-128.941166863061,33.8351517208289,193.470140433642));
#95485=CARTESIAN_POINT('Ctrl Pts',(-127.87729664587,33.6282088941676,193.581547454177));
#95486=CARTESIAN_POINT('Ctrl Pts',(-126.81071701587,33.4267339205888,193.686513206178));
#95487=CARTESIAN_POINT('Ctrl Pts',(-125.74260208096,33.2307969580634,193.785653161339));
#95488=CARTESIAN_POINT('Ctrl Pts',(-124.660791933785,33.0323477206837,193.886064274393));
#95489=CARTESIAN_POINT('Ctrl Pts',(-123.577407119073,32.8395794199289,193.980499117476));
#95490=CARTESIAN_POINT('Ctrl Pts',(-122.493654425769,32.652564947185,194.069545230172));
#95491=CARTESIAN_POINT('Ctrl Pts',(-121.980126210895,32.5639495195721,194.111739073451));
#95492=CARTESIAN_POINT('Ctrl Pts',(-121.466515184603,32.4766259807107,194.152722265915));
#95493=CARTESIAN_POINT('Ctrl Pts',(-120.952948478995,32.390602085543,194.192553446946));
#95494=CARTESIAN_POINT('Ctrl Pts',(-120.11885150105,32.250888451059,194.257244298909));
#95495=CARTESIAN_POINT('Ctrl Pts',(-119.284476123138,32.1145190215308,194.318928831136));
#95496=CARTESIAN_POINT('Ctrl Pts',(-118.449883143624,31.9813930461442,194.377867732749));
#95497=CARTESIAN_POINT('Ctrl Pts',(-117.611441106354,31.847653107328,194.437078454568));
#95498=CARTESIAN_POINT('Ctrl Pts',(-116.772779462249,31.7171866086003,194.493518045015));
#95499=CARTESIAN_POINT('Ctrl Pts',(-115.933912635633,31.5898913987512,194.54742738932));
#95500=CARTESIAN_POINT('Ctrl Pts',(-115.089760445711,31.461794152858,194.601676394775));
#95501=CARTESIAN_POINT('Ctrl Pts',(-114.245400495456,31.3369082837734,194.653363064254));
#95502=CARTESIAN_POINT('Ctrl Pts',(-113.40079958965,31.2151296972551,194.702710866655));
#95503=CARTESIAN_POINT('Ctrl Pts',(-113.248301152461,31.193141745313,194.711620947964));
#95504=CARTESIAN_POINT('Ctrl Pts',(-113.095794734474,31.1712550931384,194.720454725358));
#95505=CARTESIAN_POINT('Ctrl Pts',(-112.943279974745,31.1494691280026,194.729213442506));
#95506=CARTESIAN_POINT('Ctrl Pts',(-112.012917484241,31.0165715329257,194.782642906736));
#95507=CARTESIAN_POINT('Ctrl Pts',(-111.082171549081,30.8874107776426,194.833285574614));
#95508=CARTESIAN_POINT('Ctrl Pts',(-110.151163017163,30.7618507587285,194.881394610227));
#95509=CARTESIAN_POINT('Ctrl Pts',(-109.215546186852,30.6356692438631,194.929741775549));
#95510=CARTESIAN_POINT('Ctrl Pts',(-108.279664169512,30.513124199377,194.975530049119));
#95511=CARTESIAN_POINT('Ctrl Pts',(-107.343592216217,30.394077490774,195.018993347157));
#95512=CARTESIAN_POINT('Ctrl Pts',(-106.400548423923,30.2741441254533,195.062780358682));
#95513=CARTESIAN_POINT('Ctrl Pts',(-105.457311886688,30.1577614011017,195.104207531364));
#95514=CARTESIAN_POINT('Ctrl Pts',(-104.513911178532,30.0447880737119,195.143492362419));
#95515=CARTESIAN_POINT('Ctrl Pts',(-103.56665038208,29.9313524962783,195.182937934203));
#95516=CARTESIAN_POINT('Ctrl Pts',(-102.619224068339,29.8213542731688,195.220223489191));
#95517=CARTESIAN_POINT('Ctrl Pts',(-101.67161238576,29.7146504194992,195.255549022673));
#95518=CARTESIAN_POINT('Ctrl Pts',(-100.718092149116,29.6072812453192,195.291094818134));
#95519=CARTESIAN_POINT('Ctrl Pts',(-99.7643842389313,29.5032476508013,195.324655977918));
#95520=CARTESIAN_POINT('Ctrl Pts',(-98.8104190123668,29.4024039597289,195.356417394037));
#95521=CARTESIAN_POINT('Ctrl Pts',(-98.1692983922634,29.3346310808509,195.377762929734));
#95522=CARTESIAN_POINT('Ctrl Pts',(-97.5280605291925,29.2682989629573,195.398295200154));
#95523=CARTESIAN_POINT('Ctrl Pts',(-96.8866718339058,29.2033633869119,195.418065909768));
#95524=CARTESIAN_POINT('Ctrl Pts',(-95.8194851598921,29.0953191043508,195.450961777735));
#95525=CARTESIAN_POINT('Ctrl Pts',(-94.7519462915874,28.9911386886706,195.481748272047));
#95526=CARTESIAN_POINT('Ctrl Pts',(-93.6841635390857,28.8906537330632,195.51063659134));
#95527=CARTESIAN_POINT('Ctrl Pts',(-92.6091431308992,28.7894876693292,195.539720721727));
#95528=CARTESIAN_POINT('Ctrl Pts',(-91.5338755508916,28.6920673326612,195.566880757599));
#95529=CARTESIAN_POINT('Ctrl Pts',(-90.4584222720733,28.5982208684964,195.592312201723));
#95530=CARTESIAN_POINT('Ctrl Pts',(-89.3790508310761,28.5040324967158,195.617836299358));
#95531=CARTESIAN_POINT('Ctrl Pts',(-88.299492335566,28.413444086011,195.641619082449));
#95532=CARTESIAN_POINT('Ctrl Pts',(-87.2197595020423,28.3262818966322,195.663839656897));
#95533=CARTESIAN_POINT('Ctrl Pts',(-86.1335962252375,28.2386006052147,195.68619256792));
#95534=CARTESIAN_POINT('Ctrl Pts',(-85.0472565430152,28.1543864669692,195.70696451454));
#95535=CARTESIAN_POINT('Ctrl Pts',(-83.9607033276884,28.0734626194551,195.726320569441));
#95536=CARTESIAN_POINT('Ctrl Pts',(-82.9042804153475,27.9947828038117,195.745139877692));
#95537=CARTESIAN_POINT('Ctrl Pts',(-81.8476554011058,27.9192133283808,195.762620570897));
#95538=CARTESIAN_POINT('Ctrl Pts',(-80.7907491207154,27.8465916397671,195.778900114941));
#95539=CARTESIAN_POINT('Ctrl Pts',(-79.5927899892482,27.7642779884704,195.797352298267));
#95540=CARTESIAN_POINT('Ctrl Pts',(-78.3945110935997,27.6857558821897,195.814260762512));
#95541=CARTESIAN_POINT('Ctrl Pts',(-77.1960106267694,27.6108328461224,195.829803207285));
#95542=CARTESIAN_POINT('Ctrl Pts',(-75.9906334010089,27.5354799164742,195.845434831536));
#95543=CARTESIAN_POINT('Ctrl Pts',(-74.7850320750889,27.4637674770372,195.859684620514));
#95544=CARTESIAN_POINT('Ctrl Pts',(-73.5792566986783,27.3954997208146,195.872716012439));
#95545=CARTESIAN_POINT('Ctrl Pts',(-72.3695516951773,27.3270094796836,195.885789873725));
#95546=CARTESIAN_POINT('Ctrl Pts',(-71.1596715013674,27.2619864108281,195.89763728701));
#95547=CARTESIAN_POINT('Ctrl Pts',(-69.9496165320275,27.200232786598,195.90840734607));
#95548=CARTESIAN_POINT('Ctrl Pts',(-68.7337633573345,27.1381832582945,195.919229011888));
#95549=CARTESIAN_POINT('Ctrl Pts',(-67.5177337342398,27.0794345819982,195.928962886438));
#95550=CARTESIAN_POINT('Ctrl Pts',(-66.301477520774,27.0237861740703,195.937745524306));
#95551=CARTESIAN_POINT('Ctrl Pts',(-65.756109234319,26.9988334736939,195.941683651907));
#95552=CARTESIAN_POINT('Ctrl Pts',(-65.2106947138561,26.9745041189272,195.945430334053));
#95553=CARTESIAN_POINT('Ctrl Pts',(-64.6652261582808,26.9507800259604,195.948996999556));
#95554=CARTESIAN_POINT('Ctrl Pts',(-63.2921914866837,26.8910625557916,195.957974887188));
#95555=CARTESIAN_POINT('Ctrl Pts',(-61.9186754281437,26.8351713374488,195.965814281803));
#95556=CARTESIAN_POINT('Ctrl Pts',(-60.5448604722267,26.7828678234138,195.972681482714));
#95557=CARTESIAN_POINT('Ctrl Pts',(-59.1665103016465,26.7303916459041,195.979571353513));
#95558=CARTESIAN_POINT('Ctrl Pts',(-57.7878592656561,26.6815268991377,195.98548249961));
#95559=CARTESIAN_POINT('Ctrl Pts',(-56.4090416718605,26.6360326653217,195.990566152296));
#95560=CARTESIAN_POINT('Ctrl Pts',(-55.0256419341819,26.5903872431786,195.995666699189));
#95561=CARTESIAN_POINT('Ctrl Pts',(-53.6420745337509,26.5481347732668,195.999934147721));
#95562=CARTESIAN_POINT('Ctrl Pts',(-52.2584247821025,26.5090319279185,196.00350592515));
#95563=CARTESIAN_POINT('Ctrl Pts',(-50.8701549846142,26.4697985170583,196.007089628846));
#95564=CARTESIAN_POINT('Ctrl Pts',(-49.4818022848805,26.4337357992488,196.009972917482));
#95565=CARTESIAN_POINT('Ctrl Pts',(-48.0934022317709,26.4005980012406,196.012280609137));
#95566=CARTESIAN_POINT('Ctrl Pts',(-46.6978527766565,26.3672895640575,196.014600183977));
#95567=CARTESIAN_POINT('Ctrl Pts',(-45.3022554908575,26.3369362472909,196.016338136559));
#95568=CARTESIAN_POINT('Ctrl Pts',(-43.906595309167,26.3092884613659,196.017608406848));
#95569=CARTESIAN_POINT('Ctrl Pts',(-42.5069578153343,26.2815618855778,196.018882297116));
#95570=CARTESIAN_POINT('Ctrl Pts',(-41.1072570559494,26.256556282891,196.019685753621));
#95571=CARTESIAN_POINT('Ctrl Pts',(-39.7074265331523,26.2340199238245,196.020122080962));
#95572=CARTESIAN_POINT('Ctrl Pts',(-38.3013563474903,26.2113831102526,196.020560353207));
#95573=CARTESIAN_POINT('Ctrl Pts',(-36.8951552400075,26.1912376023804,196.020628141197));
#95574=CARTESIAN_POINT('Ctrl Pts',(-35.4887041846105,26.1733282894916,196.020419616074));
#95575=CARTESIAN_POINT('Ctrl Pts',(-34.4438796836606,26.1600238173384,196.02026470691));
#95576=CARTESIAN_POINT('Ctrl Pts',(-33.3989161740766,26.1479534359963,196.019957085882));
#95577=CARTESIAN_POINT('Ctrl Pts',(-32.3537465564776,26.1370125567383,196.019531990655));
#95578=CARTESIAN_POINT('Ctrl Pts',(-30.7854770717214,26.1205958461988,196.018894138328));
#95579=CARTESIAN_POINT('Ctrl Pts',(-29.2170110079495,26.1067517878668,196.017992423837));
#95580=CARTESIAN_POINT('Ctrl Pts',(-27.6484330828428,26.095104898452,196.016935586552));
#95581=CARTESIAN_POINT('Ctrl Pts',(-26.0759263950899,26.0834288374779,196.015876102243));
#95582=CARTESIAN_POINT('Ctrl Pts',(-24.5033072786384,26.0739609655501,196.014660632531));
#95583=CARTESIAN_POINT('Ctrl Pts',(-22.9306098968377,26.0663229709262,196.013387146679));
#95584=CARTESIAN_POINT('Ctrl Pts',(-21.352039330109,26.0586564524708,196.012108905038));
#95585=CARTESIAN_POINT('Ctrl Pts',(-19.7733899133043,26.0528335040686,196.01077213539));
#95586=CARTESIAN_POINT('Ctrl Pts',(-18.1946447084382,26.0484715597521,196.009465466002));
#95587=CARTESIAN_POINT('Ctrl Pts',(-17.5228889540512,26.0466155533579,196.00890947845));
#95588=CARTESIAN_POINT('Ctrl Pts',(-16.8511152226401,26.0450240618587,196.008358818673));
#95589=CARTESIAN_POINT('Ctrl Pts',(-16.1793193989419,26.0436676136088,196.007819795871));
#95590=CARTESIAN_POINT('Ctrl Pts',(-14.4910806772245,26.0402588272205,196.00646521888));
#95591=CARTESIAN_POINT('Ctrl Pts',(-12.8027179439815,26.0383672764135,196.005184901619));
#95592=CARTESIAN_POINT('Ctrl Pts',(-11.1143235409627,26.037377069714,196.004071270348));
#95593=CARTESIAN_POINT('Ctrl Pts',(-9.42199598084912,26.0363845563031,196.002955044845));
#95594=CARTESIAN_POINT('Ctrl Pts',(-7.72963659586614,26.0362975912985,196.002006202154));
#95595=CARTESIAN_POINT('Ctrl Pts',(-6.03728696792206,26.0364959689877,196.001307542158));
#95596=CARTESIAN_POINT('Ctrl Pts',(-4.33934640493638,26.0366950020479,196.000606574032));
#95597=CARTESIAN_POINT('Ctrl Pts',(-2.6414156613371,26.0371812662625,196.000157369753));
#95598=CARTESIAN_POINT('Ctrl Pts',(-0.94348510617516,26.0373283887573,196.000034389117));
#95599=CARTESIAN_POINT('Ctrl Pts',(-0.628990291197994,26.0373556391426,
196.000011610345));
#95600=CARTESIAN_POINT('Ctrl Pts',(-0.314495340669711,26.0373712544753,
196.));
#95601=CARTESIAN_POINT('Ctrl Pts',(2.8421709430404E-14,26.0373712544753,
196.));
#95602=CARTESIAN_POINT('Ctrl Pts',(-175.744237881275,22.546886555333,150.608265410388));
#95603=CARTESIAN_POINT('Ctrl Pts',(-175.908702878622,22.6788155043369,150.370416902681));
#95604=CARTESIAN_POINT('Ctrl Pts',(-176.070305087181,22.8100740741211,150.130584015011));
#95605=CARTESIAN_POINT('Ctrl Pts',(-176.229190935516,22.9406832143353,149.889269308473));
#95606=CARTESIAN_POINT('Ctrl Pts',(-176.242451717849,22.9515839924555,149.869128925734));
#95607=CARTESIAN_POINT('Ctrl Pts',(-176.255693602711,22.9624802562284,149.848978236114));
#95608=CARTESIAN_POINT('Ctrl Pts',(-176.268916688211,22.9733720229219,149.828817539881));
#95609=CARTESIAN_POINT('Ctrl Pts',(-176.44103106749,23.1151414808645,149.566401803559));
#95610=CARTESIAN_POINT('Ctrl Pts',(-176.610110587624,23.2562741012296,149.302035066109));
#95611=CARTESIAN_POINT('Ctrl Pts',(-176.776388927648,23.3968919164516,149.035943859508));
#95612=CARTESIAN_POINT('Ctrl Pts',(-176.942667267672,23.5375097316736,148.769852652907));
#95613=CARTESIAN_POINT('Ctrl Pts',(-177.106144812233,23.6776129639275,148.502037017761));
#95614=CARTESIAN_POINT('Ctrl Pts',(-177.267103401469,23.817346041801,148.232728813506));
#95615=CARTESIAN_POINT('Ctrl Pts',(-177.363999318881,23.9014643534589,148.070607204205));
#95616=CARTESIAN_POINT('Ctrl Pts',(-177.459978494646,23.9854462723562,147.907944307097));
#95617=CARTESIAN_POINT('Ctrl Pts',(-177.555073691723,24.0693089296899,147.744787763983));
#95618=CARTESIAN_POINT('Ctrl Pts',(-177.742739096476,24.2348075039171,147.422806847571));
#95619=CARTESIAN_POINT('Ctrl Pts',(-177.926980239791,24.3998589145364,147.098876637803));
#95620=CARTESIAN_POINT('Ctrl Pts',(-178.108158130897,24.5646751337556,146.773242494141));
#95621=CARTESIAN_POINT('Ctrl Pts',(-178.135162221033,24.5892405595513,146.724707577914));
#95622=CARTESIAN_POINT('Ctrl Pts',(-178.162098345943,24.6138007991985,146.676134818599));
#95623=CARTESIAN_POINT('Ctrl Pts',(-178.188967788788,24.6383565940794,146.627525038914));
#95624=CARTESIAN_POINT('Ctrl Pts',(-178.387133584952,24.819458921767,146.269021301122));
#95625=CARTESIAN_POINT('Ctrl Pts',(-178.581657096816,25.0003113926081,145.90850229487));
#95626=CARTESIAN_POINT('Ctrl Pts',(-178.772869825489,25.1811314130801,145.546279049829));
#95627=CARTESIAN_POINT('Ctrl Pts',(-178.86617158637,25.2693620786306,145.369533145784));
#95628=CARTESIAN_POINT('Ctrl Pts',(-178.958685835325,25.3575853437931,145.192381566129));
#95629=CARTESIAN_POINT('Ctrl Pts',(-179.050455154588,25.4458281382592,145.014860934436));
#95630=CARTESIAN_POINT('Ctrl Pts',(-179.092385660168,25.4861473322497,144.933749622971));
#95631=CARTESIAN_POINT('Ctrl Pts',(-179.134162006972,25.5264707409745,144.852561419544));
#95632=CARTESIAN_POINT('Ctrl Pts',(-179.17578644388,25.5668003915238,144.771299621934));
#95633=CARTESIAN_POINT('Ctrl Pts',(-179.39260672159,25.7768761710768,144.34800967897));
#95634=CARTESIAN_POINT('Ctrl Pts',(-179.605309522255,25.9871277930927,143.922719571555));
#95635=CARTESIAN_POINT('Ctrl Pts',(-179.814294542222,26.1979040977535,143.495807476513));
#95636=CARTESIAN_POINT('Ctrl Pts',(-180.037734528063,26.4232592669264,143.03936695036));
#95637=CARTESIAN_POINT('Ctrl Pts',(-180.256924825074,26.6492146536794,142.581072304569));
#95638=CARTESIAN_POINT('Ctrl Pts',(-180.47241005792,26.8762157659472,142.121392484689));
#95639=CARTESIAN_POINT('Ctrl Pts',(-180.527030915697,26.9337556507213,142.004873567206));
#95640=CARTESIAN_POINT('Ctrl Pts',(-180.581413973102,26.9913627943564,141.888265681818));
#95641=CARTESIAN_POINT('Ctrl Pts',(-180.635568590654,27.0490445708111,141.771576526924));
#95642=CARTESIAN_POINT('Ctrl Pts',(-180.886093230566,27.3158861981584,141.231760905778));
#95643=CARTESIAN_POINT('Ctrl Pts',(-181.131684690975,27.5842894890372,140.690201281687));
#95644=CARTESIAN_POINT('Ctrl Pts',(-181.372929297185,27.8550313552204,140.147621216792));
#95645=CARTESIAN_POINT('Ctrl Pts',(-181.594737305059,28.1039600874706,139.648755749095));
#95646=CARTESIAN_POINT('Ctrl Pts',(-181.812872298084,28.3548669042706,139.149027826144));
#95647=CARTESIAN_POINT('Ctrl Pts',(-182.02782728574,28.6083467745418,138.649005217546));
#95648=CARTESIAN_POINT('Ctrl Pts',(-182.04782703148,28.631930935164,138.602482337826));
#95649=CARTESIAN_POINT('Ctrl Pts',(-182.067799817512,28.6555380045141,138.555955681339));
#95650=CARTESIAN_POINT('Ctrl Pts',(-182.087745982222,28.6791683785366,138.509425856118));
#95651=CARTESIAN_POINT('Ctrl Pts',(-182.299276287944,28.9297699510136,138.015974192752));
#95652=CARTESIAN_POINT('Ctrl Pts',(-182.507800014602,29.182970670716,137.522164174549));
#95653=CARTESIAN_POINT('Ctrl Pts',(-182.713589982161,29.4394358963928,137.028706746927));
#95654=CARTESIAN_POINT('Ctrl Pts',(-182.901130257844,29.6731574898079,136.579009693605));
#95655=CARTESIAN_POINT('Ctrl Pts',(-183.086401030652,29.9095908775968,136.129605579487));
#95656=CARTESIAN_POINT('Ctrl Pts',(-183.269620366698,30.1491974649295,135.681035410223));
#95657=CARTESIAN_POINT('Ctrl Pts',(-183.330707454486,30.2290846043046,135.531477804022));
#95658=CARTESIAN_POINT('Ctrl Pts',(-183.391566549221,30.3093240737019,135.382012919852));
#95659=CARTESIAN_POINT('Ctrl Pts',(-183.452205819528,30.3899316377764,135.232660860471));
#95660=CARTESIAN_POINT('Ctrl Pts',(-183.614088692094,30.605121958454,134.833949921601));
#95661=CARTESIAN_POINT('Ctrl Pts',(-183.774414717316,30.822931855176,134.436042377523));
#95662=CARTESIAN_POINT('Ctrl Pts',(-183.933260187282,31.0438149196179,134.039316900741));
#95663=CARTESIAN_POINT('Ctrl Pts',(-184.083805069754,31.2531555761914,133.663322607113));
#95664=CARTESIAN_POINT('Ctrl Pts',(-184.233020269242,31.4652568189183,133.288390095977));
#95665=CARTESIAN_POINT('Ctrl Pts',(-184.380969182443,31.6804576051001,132.914842397316));
#95666=CARTESIAN_POINT('Ctrl Pts',(-184.435603688472,31.7599268515842,132.776898876452));
#95667=CARTESIAN_POINT('Ctrl Pts',(-184.49006548564,31.8398182782547,132.639144203768));
#95668=CARTESIAN_POINT('Ctrl Pts',(-184.544357638816,31.9201471237056,132.501594660764));
#95669=CARTESIAN_POINT('Ctrl Pts',(-184.617819762747,32.0288392137119,132.315477865177));
#95670=CARTESIAN_POINT('Ctrl Pts',(-184.690974787393,32.1383373743561,132.12972991714));
#95671=CARTESIAN_POINT('Ctrl Pts',(-184.763835795633,32.2486855326466,131.944376242217));
#95672=CARTESIAN_POINT('Ctrl Pts',(-184.908108059022,32.4671861949611,131.577356970119));
#95673=CARTESIAN_POINT('Ctrl Pts',(-185.051273897465,32.6890839232354,131.211883205961));
#95674=CARTESIAN_POINT('Ctrl Pts',(-185.193246738383,32.9147242786968,130.848150885959));
#95675=CARTESIAN_POINT('Ctrl Pts',(-185.332338778526,33.1357861182467,130.491799134966));
#95676=CARTESIAN_POINT('Ctrl Pts',(-185.470285743725,33.3604403311696,130.137118880231));
#95677=CARTESIAN_POINT('Ctrl Pts',(-185.607009479458,33.5889617133876,129.784294086801));
#95678=CARTESIAN_POINT('Ctrl Pts',(-185.643105683007,33.6492932592125,129.691145406418));
#95679=CARTESIAN_POINT('Ctrl Pts',(-185.679116644919,33.7098940684669,129.598126050538));
#95680=CARTESIAN_POINT('Ctrl Pts',(-185.715040966049,33.770768586648,129.505239400064));
#95681=CARTESIAN_POINT('Ctrl Pts',(-185.826219135776,33.9591623349881,129.21777487835));
#95682=CARTESIAN_POINT('Ctrl Pts',(-185.936515312922,34.15009092431,128.931710214066));
#95683=CARTESIAN_POINT('Ctrl Pts',(-186.045906297122,34.3436896511963,128.647105949505));
#95684=CARTESIAN_POINT('Ctrl Pts',(-186.187963906724,34.5951013426148,128.277512405741));
#95685=CARTESIAN_POINT('Ctrl Pts',(-186.328581615584,34.8513141937532,127.910381712665));
#95686=CARTESIAN_POINT('Ctrl Pts',(-186.467167928252,35.1117711144459,127.545845380182));
#95687=CARTESIAN_POINT('Ctrl Pts',(-186.587608752915,35.3381256924236,127.22903879475));
#95688=CARTESIAN_POINT('Ctrl Pts',(-186.706516042193,35.5676857771387,126.914191656203));
#95689=CARTESIAN_POINT('Ctrl Pts',(-186.823533306774,35.8000896127479,126.601389596021));
#95690=CARTESIAN_POINT('Ctrl Pts',(-186.935264325339,36.0219946227828,126.302718345085));
#95691=CARTESIAN_POINT('Ctrl Pts',(-187.045298175341,36.2465364855314,126.005843786788));
#95692=CARTESIAN_POINT('Ctrl Pts',(-187.153519980204,36.4737898819313,125.710359064098));
#95693=CARTESIAN_POINT('Ctrl Pts',(-187.198434955774,36.5681061868602,125.587724913636));
#95694=CARTESIAN_POINT('Ctrl Pts',(-187.243037899464,36.6628901737859,125.465330144598));
#95695=CARTESIAN_POINT('Ctrl Pts',(-187.287320824454,36.7581497766535,125.343145615419));
#95696=CARTESIAN_POINT('Ctrl Pts',(-187.38529512183,36.9689080466076,125.072816963927));
#95697=CARTESIAN_POINT('Ctrl Pts',(-187.481592779837,37.1819935292495,124.80351797177));
#95698=CARTESIAN_POINT('Ctrl Pts',(-187.575959132587,37.3967240017217,124.53493166223));
#95699=CARTESIAN_POINT('Ctrl Pts',(-187.663018946538,37.5948284577938,124.287141285079));
#95700=CARTESIAN_POINT('Ctrl Pts',(-187.748435398913,37.7943346717978,124.039957489253));
#95701=CARTESIAN_POINT('Ctrl Pts',(-187.832006518938,37.9947459637195,123.793130970979));
#95702=CARTESIAN_POINT('Ctrl Pts',(-187.931222863557,38.2326759543536,123.500096428773));
#95703=CARTESIAN_POINT('Ctrl Pts',(-188.027871329892,38.4719542366046,123.207477462073));
#95704=CARTESIAN_POINT('Ctrl Pts',(-188.121669748411,38.71200239098,122.914628621077));
#95705=CARTESIAN_POINT('Ctrl Pts',(-188.206651476469,38.9294869424027,122.649306444432));
#95706=CARTESIAN_POINT('Ctrl Pts',(-188.289294089793,39.1476058176956,122.383795546001));
#95707=CARTESIAN_POINT('Ctrl Pts',(-188.369345374146,39.3659272509012,122.117615059027));
#95708=CARTESIAN_POINT('Ctrl Pts',(-188.377650540578,39.3885776787255,122.089999346635));
#95709=CARTESIAN_POINT('Ctrl Pts',(-188.385927771447,39.4112302682003,122.062376426411));
#95710=CARTESIAN_POINT('Ctrl Pts',(-188.394176753812,39.4338845216231,122.034745760962));
#95711=CARTESIAN_POINT('Ctrl Pts',(-188.467578797548,39.6354692052961,121.78887939537));
#95712=CARTESIAN_POINT('Ctrl Pts',(-188.538661405825,39.8368471399804,121.542399924329));
#95713=CARTESIAN_POINT('Ctrl Pts',(-188.607469504649,40.037770592676,121.294926617));
#95714=CARTESIAN_POINT('Ctrl Pts',(-188.634278299083,40.1160537545741,121.198506847565));
#95715=CARTESIAN_POINT('Ctrl Pts',(-188.660741457239,40.1942675384835,121.101936207836));
#95716=CARTESIAN_POINT('Ctrl Pts',(-188.686860236094,40.2723955794952,121.005192162795));
#95717=CARTESIAN_POINT('Ctrl Pts',(-188.747793540263,40.4546628942767,120.779494998471));
#95718=CARTESIAN_POINT('Ctrl Pts',(-188.806812883497,40.6363432015775,120.552805785747));
#95719=CARTESIAN_POINT('Ctrl Pts',(-188.863919259891,40.8171855501551,120.32493878908));
#95720=CARTESIAN_POINT('Ctrl Pts',(-188.9195764212,40.9934385783092,120.10285447921));
#95721=CARTESIAN_POINT('Ctrl Pts',(-188.973416356601,41.1688959671253,119.87965139287));
#95722=CARTESIAN_POINT('Ctrl Pts',(-189.025418324791,41.3432817233448,119.655156510801));
#95723=CARTESIAN_POINT('Ctrl Pts',(-189.075659196967,41.5117617404008,119.438264361006));
#95724=CARTESIAN_POINT('Ctrl Pts',(-189.124184353139,41.6792416727984,119.220166418816));
#95725=CARTESIAN_POINT('Ctrl Pts',(-189.170956450069,41.8454277028942,119.000705813639));
#95726=CARTESIAN_POINT('Ctrl Pts',(-189.190583026184,41.9151629293015,118.90861543167));
#95727=CARTESIAN_POINT('Ctrl Pts',(-189.209900700109,41.9846697503341,118.816285099538));
#95728=CARTESIAN_POINT('Ctrl Pts',(-189.228905765118,42.0539238525625,118.723703186652));
#95729=CARTESIAN_POINT('Ctrl Pts',(-189.269701749122,42.2025836569575,118.524968258072));
#95730=CARTESIAN_POINT('Ctrl Pts',(-189.309122104735,42.3501377294883,118.325073829805));
#95731=CARTESIAN_POINT('Ctrl Pts',(-189.347227030635,42.496617577999,118.123903895185));
#95732=CARTESIAN_POINT('Ctrl Pts',(-189.41133846046,42.7430695079501,117.785436050364));
#95733=CARTESIAN_POINT('Ctrl Pts',(-189.471642745778,42.9861722585085,117.443390482533));
#95734=CARTESIAN_POINT('Ctrl Pts',(-189.528369432274,43.2256914913882,117.097684460107));
#95735=CARTESIAN_POINT('Ctrl Pts',(-189.583560824824,43.4587281945992,116.761334886931));
#95736=CARTESIAN_POINT('Ctrl Pts',(-189.635365277565,43.6883725336104,116.421520292599));
#95737=CARTESIAN_POINT('Ctrl Pts',(-189.684025408118,43.9143710383731,116.078162647865));
#95738=CARTESIAN_POINT('Ctrl Pts',(-189.71533602662,44.0597909721935,115.857227354393));
#95739=CARTESIAN_POINT('Ctrl Pts',(-189.745345430984,44.2037006513986,115.634825079113));
#95740=CARTESIAN_POINT('Ctrl Pts',(-189.774126467365,44.3460245195935,115.410934680711));
#95741=CARTESIAN_POINT('Ctrl Pts',(-189.788646208236,44.4178254672295,115.297984246074));
#95742=CARTESIAN_POINT('Ctrl Pts',(-189.80285892525,44.4892404437514,115.184655369196));
#95743=CARTESIAN_POINT('Ctrl Pts',(-189.816771882395,44.5602764703106,115.070945604173));
#95744=CARTESIAN_POINT('Ctrl Pts',(-189.845878495638,44.7088874470996,114.833058998333));
#95745=CARTESIAN_POINT('Ctrl Pts',(-189.873666771693,44.8558147467008,114.593508547228));
#95746=CARTESIAN_POINT('Ctrl Pts',(-189.900169411116,45.0008888701078,114.352652858109));
#95747=CARTESIAN_POINT('Ctrl Pts',(-189.927395037922,45.1499205903126,114.105226667775));
#95748=CARTESIAN_POINT('Ctrl Pts',(-189.953264055466,45.2969967153742,113.856423060368));
#95749=CARTESIAN_POINT('Ctrl Pts',(-189.977840198345,45.4419804406038,113.606631315635));
#95750=CARTESIAN_POINT('Ctrl Pts',(-189.982109404138,45.4671660591443,113.563239137737));
#95751=CARTESIAN_POINT('Ctrl Pts',(-189.986339659915,45.4922886464614,113.51981714256));
#95752=CARTESIAN_POINT('Ctrl Pts',(-189.990531378616,45.5173476214414,113.476367372042));
#95753=CARTESIAN_POINT('Ctrl Pts',(-190.024309750992,45.7192818275872,113.126233540803));
#95754=CARTESIAN_POINT('Ctrl Pts',(-190.055618148429,45.9172926050588,112.773946819036));
#95755=CARTESIAN_POINT('Ctrl Pts',(-190.084773825985,46.1116429059189,112.419679369385));
#95756=CARTESIAN_POINT('Ctrl Pts',(-190.093605530925,46.1705146131193,112.312366288447));
#95757=CARTESIAN_POINT('Ctrl Pts',(-190.102239941155,46.2290507217143,112.204871457883));
#95758=CARTESIAN_POINT('Ctrl Pts',(-190.110686478729,46.2872592582712,112.097199656883));
#95759=CARTESIAN_POINT('Ctrl Pts',(-190.117126005374,46.3316366636664,112.015112123932));
#95760=CARTESIAN_POINT('Ctrl Pts',(-190.123455889712,46.3758232353185,111.932921222337));
#95761=CARTESIAN_POINT('Ctrl Pts',(-190.129678414464,46.419824581143,111.850629008613));
#95762=CARTESIAN_POINT('Ctrl Pts',(-190.155150488636,46.5999452860367,111.513763595398));
#95763=CARTESIAN_POINT('Ctrl Pts',(-190.178819063545,46.7769386360979,111.175174863812));
#95764=CARTESIAN_POINT('Ctrl Pts',(-190.200847352509,46.9511673688017,110.835089165966));
#95765=CARTESIAN_POINT('Ctrl Pts',(-190.223891565535,47.1334313675208,110.479319034172));
#95766=CARTESIAN_POINT('Ctrl Pts',(-190.245140712285,47.31266995987,110.121910676907));
#95767=CARTESIAN_POINT('Ctrl Pts',(-190.264805352682,47.4893524414545,109.763123230192));
#95768=CARTESIAN_POINT('Ctrl Pts',(-190.282639426873,47.6495876871243,109.437735030117));
#95769=CARTESIAN_POINT('Ctrl Pts',(-190.299170675221,47.8077215438186,109.11121254813));
#95770=CARTESIAN_POINT('Ctrl Pts',(-190.31457133704,47.9641377788197,108.783749054156));
#95771=CARTESIAN_POINT('Ctrl Pts',(-190.3186324918,48.0053847424114,108.697396925725));
#95772=CARTESIAN_POINT('Ctrl Pts',(-190.322613497865,48.0465130238487,108.610979412536));
#95773=CARTESIAN_POINT('Ctrl Pts',(-190.326516429816,48.0875360219424,108.524500248369));
#95774=CARTESIAN_POINT('Ctrl Pts',(-190.347470973244,48.3077853641662,108.060200223779));
#95775=CARTESIAN_POINT('Ctrl Pts',(-190.366165850257,48.5249327446489,107.594151454416));
#95776=CARTESIAN_POINT('Ctrl Pts',(-190.382938268006,48.7409820320843,107.127459866807));
#95777=CARTESIAN_POINT('Ctrl Pts',(-190.386425985993,48.7859081123401,107.030414308507));
#95778=CARTESIAN_POINT('Ctrl Pts',(-190.389830635255,48.8307748699332,106.933340624158));
#95779=CARTESIAN_POINT('Ctrl Pts',(-190.3931546158,48.875624857867,106.836249384426));
#95780=CARTESIAN_POINT('Ctrl Pts',(-190.401482760198,48.9879953036755,106.592989878786));
#95781=CARTESIAN_POINT('Ctrl Pts',(-190.409300674852,49.1002112103535,106.349587462763));
#95782=CARTESIAN_POINT('Ctrl Pts',(-190.416648501021,49.2129329835915,106.106403549491));
#95783=CARTESIAN_POINT('Ctrl Pts',(-190.423045207733,49.3110637921878,105.894697919234));
#95784=CARTESIAN_POINT('Ctrl Pts',(-190.429085626652,49.4095780398654,105.683157832093));
#95785=CARTESIAN_POINT('Ctrl Pts',(-190.434796191365,49.5088790511891,105.472019538342));
#95786=CARTESIAN_POINT('Ctrl Pts',(-190.437734685736,49.5599765305866,105.363373770578));
#95787=CARTESIAN_POINT('Ctrl Pts',(-190.440585807973,49.611162274679,105.254832348517));
#95788=CARTESIAN_POINT('Ctrl Pts',(-190.443352111172,49.6626721329211,105.146434935855));
#95789=CARTESIAN_POINT('Ctrl Pts',(-190.447571428625,49.7412377955184,104.981101253329));
#95790=CARTESIAN_POINT('Ctrl Pts',(-190.451593258618,49.8205686724301,104.816139230826));
#95791=CARTESIAN_POINT('Ctrl Pts',(-190.455414205516,49.9011704353188,104.651848944708));
#95792=CARTESIAN_POINT('Ctrl Pts',(-190.458076115421,49.9573226501258,104.537394085334));
#95793=CARTESIAN_POINT('Ctrl Pts',(-190.460640829764,50.0140930954728,104.423265371995));
#95794=CARTESIAN_POINT('Ctrl Pts',(-190.463110495386,50.0716668432943,104.309565487542));
#95795=CARTESIAN_POINT('Ctrl Pts',(-190.465509387058,50.1275906829144,104.199123934862));
#95796=CARTESIAN_POINT('Ctrl Pts',(-190.46782537944,50.184430059915,104.089064186709));
#95797=CARTESIAN_POINT('Ctrl Pts',(-190.470059472272,50.242337358968,103.979614063443));
#95798=CARTESIAN_POINT('Ctrl Pts',(-190.471153763902,50.2707012084011,103.926003778254));
#95799=CARTESIAN_POINT('Ctrl Pts',(-190.472228401696,50.2993205360378,103.872539719887));
#95800=CARTESIAN_POINT('Ctrl Pts',(-190.473283481554,50.3282085918218,103.819248459061));
#95801=CARTESIAN_POINT('Ctrl Pts',(-190.474860709149,50.3713930374174,103.739583923273));
#95802=CARTESIAN_POINT('Ctrl Pts',(-190.476394184613,50.4150658005626,103.660301066565));
#95803=CARTESIAN_POINT('Ctrl Pts',(-190.47788357534,50.4597519396773,103.58150526024));
#95804=CARTESIAN_POINT('Ctrl Pts',(-190.478463762675,50.4771592804534,103.550810609066));
#95805=CARTESIAN_POINT('Ctrl Pts',(-190.479037260371,50.4947198656172,103.520189846983));
#95806=CARTESIAN_POINT('Ctrl Pts',(-190.479604049555,50.5124625282476,103.489649124445));
#95807=CARTESIAN_POINT('Ctrl Pts',(-190.480619357872,50.54424554994,103.434940512376));
#95808=CARTESIAN_POINT('Ctrl Pts',(-190.481609405472,50.5764981037343,103.38048925242));
#95809=CARTESIAN_POINT('Ctrl Pts',(-190.482573587812,50.6093230551895,103.326508708962));
#95810=CARTESIAN_POINT('Ctrl Pts',(-190.483480289518,50.6401911164417,103.275746266125));
#95811=CARTESIAN_POINT('Ctrl Pts',(-190.484364110455,50.67156559899,103.225400089796));
#95812=CARTESIAN_POINT('Ctrl Pts',(-190.485224213747,50.7034859716933,103.175645783279));
#95813=CARTESIAN_POINT('Ctrl Pts',(-190.485693564421,50.7209046336072,103.148495303176));
#95814=CARTESIAN_POINT('Ctrl Pts',(-190.486155847173,50.738485007477,103.121521036496));
#95815=CARTESIAN_POINT('Ctrl Pts',(-190.486610891693,50.7562268616243,103.094751266519));
#95816=CARTESIAN_POINT('Ctrl Pts',(-190.487171560686,50.7780869369309,103.061767724732));
#95817=CARTESIAN_POINT('Ctrl Pts',(-190.487724180922,50.8003067802776,103.028929310287));
#95818=CARTESIAN_POINT('Ctrl Pts',(-190.488268410957,50.8228991405886,102.996250130195));
#95819=CARTESIAN_POINT('Ctrl Pts',(-190.489052241381,50.8554379168998,102.949183753932));
#95820=CARTESIAN_POINT('Ctrl Pts',(-190.489818400132,50.8886218581293,102.902459464589));
#95821=CARTESIAN_POINT('Ctrl Pts',(-190.490565574978,50.9230915750538,102.856163776289));
#95822=CARTESIAN_POINT('Ctrl Pts',(-190.491265949113,50.9554022160489,102.812767906007));
#95823=CARTESIAN_POINT('Ctrl Pts',(-190.491949650515,50.9888425049264,102.76974862589));
#95824=CARTESIAN_POINT('Ctrl Pts',(-190.492616032225,51.0238897102706,102.727173554288));
#95825=CARTESIAN_POINT('Ctrl Pts',(-190.492660561478,51.0262316501122,102.724328584041));
#95826=CARTESIAN_POINT('Ctrl Pts',(-190.492705013542,51.0285807458312,102.721485595865));
#95827=CARTESIAN_POINT('Ctrl Pts',(-190.492749388285,51.0309371314078,102.718644609311));
#95828=CARTESIAN_POINT('Ctrl Pts',(-190.493173137558,51.0534390456138,102.691515078253));
#95829=CARTESIAN_POINT('Ctrl Pts',(-190.493585842178,51.0763984440354,102.664839908867));
#95830=CARTESIAN_POINT('Ctrl Pts',(-190.493986293241,51.0997856641685,102.638721920427));
#95831=CARTESIAN_POINT('Ctrl Pts',(-190.494246786517,51.1149990426479,102.621732178124));
#95832=CARTESIAN_POINT('Ctrl Pts',(-190.494502098002,51.1303924656902,102.604978141484));
#95833=CARTESIAN_POINT('Ctrl Pts',(-190.49475193048,51.1459458605707,102.588487321706));
#95834=CARTESIAN_POINT('Ctrl Pts',(-190.495025958524,51.1630055574701,102.570399412976));
#95835=CARTESIAN_POINT('Ctrl Pts',(-190.495293609111,51.1802133663293,102.552613124357));
#95836=CARTESIAN_POINT('Ctrl Pts',(-190.495554183348,51.1977393721181,102.535187035469));
#95837=CARTESIAN_POINT('Ctrl Pts',(-190.495800955596,51.214337067625,102.518683964506));
#95838=CARTESIAN_POINT('Ctrl Pts',(-190.496041381906,51.2312198938965,102.502503925468));
#95839=CARTESIAN_POINT('Ctrl Pts',(-190.49627495862,51.2484810562372,102.486691839988));
#95840=CARTESIAN_POINT('Ctrl Pts',(-190.496507440142,51.2656612846284,102.470953894041));
#95841=CARTESIAN_POINT('Ctrl Pts',(-190.4967331362,51.2832163684952,102.455580467278));
#95842=CARTESIAN_POINT('Ctrl Pts',(-190.496951637893,51.3011868238247,102.440610966142));
#95843=CARTESIAN_POINT('Ctrl Pts',(-190.497170421921,51.319180499469,102.42562212234));
#95844=CARTESIAN_POINT('Ctrl Pts',(-190.49738199311,51.3375906224577,102.411038251086));
#95845=CARTESIAN_POINT('Ctrl Pts',(-190.497586027925,51.3564056935099,102.396893915589));
#95846=CARTESIAN_POINT('Ctrl Pts',(-190.497622036443,51.3597262191685,102.394397691748));
#95847=CARTESIAN_POINT('Ctrl Pts',(-190.497657810449,51.3630592267632,102.391915145125));
#95848=CARTESIAN_POINT('Ctrl Pts',(-190.497693348437,51.3664044859326,102.389446449618));
#95849=CARTESIAN_POINT('Ctrl Pts',(-190.497698185796,51.3668598358445,102.389110415779));
#95850=CARTESIAN_POINT('Ctrl Pts',(-190.497703018127,51.3673153510038,102.388774686009));
#95851=CARTESIAN_POINT('Ctrl Pts',(-190.497707845407,51.3677710284501,102.388439262075));
#95852=CARTESIAN_POINT('Ctrl Pts',(-190.497829956126,51.3792978295723,102.379954389689));
#95853=CARTESIAN_POINT('Ctrl Pts',(-190.49794870553,51.3908794562608,102.371673743334));
#95854=CARTESIAN_POINT('Ctrl Pts',(-190.49806353266,51.4025952328269,102.363640762749));
#95855=CARTESIAN_POINT('Ctrl Pts',(-190.498176084254,51.4140788371052,102.35576697225));
#95856=CARTESIAN_POINT('Ctrl Pts',(-190.49828486745,51.4256914109588,102.348131139072));
#95857=CARTESIAN_POINT('Ctrl Pts',(-190.498389448386,51.4374575098775,102.340767949979));
#95858=CARTESIAN_POINT('Ctrl Pts',(-190.498493937874,51.4492133202251,102.333411199444));
#95859=CARTESIAN_POINT('Ctrl Pts',(-190.498594232461,51.4611224309089,102.326326621791));
#95860=CARTESIAN_POINT('Ctrl Pts',(-190.498689995252,51.473157593797,102.31954239481));
#95861=CARTESIAN_POINT('Ctrl Pts',(-190.498787203883,51.4853744653403,102.312655738574));
#95862=CARTESIAN_POINT('Ctrl Pts',(-190.498879742976,51.4977211980772,102.306078567821));
#95863=CARTESIAN_POINT('Ctrl Pts',(-190.498967358278,51.5101155779645,102.299833692461));
#95864=CARTESIAN_POINT('Ctrl Pts',(-190.499000191867,51.5147603370296,102.297493442952));
#95865=CARTESIAN_POINT('Ctrl Pts',(-190.499032334942,51.5194112573811,102.295199793732));
#95866=CARTESIAN_POINT('Ctrl Pts',(-190.499063777468,51.5240621615258,102.292953715569));
#95867=CARTESIAN_POINT('Ctrl Pts',(-190.499127550844,51.5334953684055,102.288398102442));
#95868=CARTESIAN_POINT('Ctrl Pts',(-190.499188701791,51.5429635346423,102.284018903747));
#95869=CARTESIAN_POINT('Ctrl Pts',(-190.49924660439,51.5524660168867,102.279864143773));
#95870=CARTESIAN_POINT('Ctrl Pts',(-190.499275923368,51.5572775982511,102.277760381287));
#95871=CARTESIAN_POINT('Ctrl Pts',(-190.499304413945,51.5620971811844,102.27571383855));
#95872=CARTESIAN_POINT('Ctrl Pts',(-190.49933202114,51.5669200122158,102.273728831663));
#95873=CARTESIAN_POINT('Ctrl Pts',(-190.499401179922,51.5790016855048,102.26875619121));
#95874=CARTESIAN_POINT('Ctrl Pts',(-190.499466261876,51.5913660796301,102.264061108971));
#95875=CARTESIAN_POINT('Ctrl Pts',(-190.499526819669,51.6040357712666,102.259679993778));
#95876=CARTESIAN_POINT('Ctrl Pts',(-190.499575160619,51.6141494972118,102.256182718575));
#95877=CARTESIAN_POINT('Ctrl Pts',(-190.499620626327,51.6244565361271,102.252884943998));
#95878=CARTESIAN_POINT('Ctrl Pts',(-190.499663124803,51.6349470309206,102.249795087218));
#95879=CARTESIAN_POINT('Ctrl Pts',(-190.499707459708,51.6458908374787,102.246571712576));
#95880=CARTESIAN_POINT('Ctrl Pts',(-190.499749250184,51.6572266217615,102.243522398947));
#95881=CARTESIAN_POINT('Ctrl Pts',(-190.499786904165,51.6688350796959,102.24076878861));
#95882=CARTESIAN_POINT('Ctrl Pts',(-190.499797766025,51.6721837149382,102.239974468066));
#95883=CARTESIAN_POINT('Ctrl Pts',(-190.499808288085,51.6755550949733,102.239204421804));
#95884=CARTESIAN_POINT('Ctrl Pts',(-190.499818442416,51.6789464892751,102.238460794519));
#95885=CARTESIAN_POINT('Ctrl Pts',(-190.49985255672,51.6903401557494,102.235962517845));
#95886=CARTESIAN_POINT('Ctrl Pts',(-190.4998824689,51.7019610574954,102.23376631126));
#95887=CARTESIAN_POINT('Ctrl Pts',(-190.499907362821,51.7136418981571,102.231935917858));
#95888=CARTESIAN_POINT('Ctrl Pts',(-190.499932499582,51.7254366852798,102.230087668989));
#95889=CARTESIAN_POINT('Ctrl Pts',(-190.499952519172,51.7372923374136,102.228612429663));
#95890=CARTESIAN_POINT('Ctrl Pts',(-190.499967274851,51.7490230427039,102.227523777426));
#95891=CARTESIAN_POINT('Ctrl Pts',(-190.499982652175,51.7612479527539,102.226389261185));
#95892=CARTESIAN_POINT('Ctrl Pts',(-190.499992312906,51.7733368621914,102.225674559321));
#95893=CARTESIAN_POINT('Ctrl Pts',(-190.499996850844,51.7850689572221,102.225338275583));
#95894=CARTESIAN_POINT('Ctrl Pts',(-190.499998988428,51.7905953287186,102.225179870041));
#95895=CARTESIAN_POINT('Ctrl Pts',(-190.5,51.7960424097962,102.225104635364));
#95896=CARTESIAN_POINT('Ctrl Pts',(-190.5,51.8013867006572,102.225104347682));
#95897=CARTESIAN_POINT('Ctrl Pts',(190.469429429736,54.1262777440014,110.636021302185));
#95898=CARTESIAN_POINT('Ctrl Pts',(190.470286237567,57.114886044131,110.505619326269));
#95899=CARTESIAN_POINT('Ctrl Pts',(190.390488824897,60.0974355462687,110.365455132863));
#95900=CARTESIAN_POINT('Ctrl Pts',(190.500739017087,52.1710967193735,102.073694012035));
#95901=CARTESIAN_POINT('Ctrl Pts',(190.500921335563,52.6730706221047,102.021024092992));
#95902=CARTESIAN_POINT('Ctrl Pts',(190.503306943774,53.175064208621,101.968360125277));
#95903=CARTESIAN_POINT('Ctrl Pts',(190.500187664912,51.8514724777866,102.229958216589));
#95904=CARTESIAN_POINT('Ctrl Pts',(190.500381911772,51.9211334344651,102.175808890008));
#95905=CARTESIAN_POINT('Ctrl Pts',(190.501435020995,51.9907954565713,102.121657812393));
#95906=CARTESIAN_POINT('Ctrl Pts',(190.499591926775,51.7334252320839,102.391035770384));
#95907=CARTESIAN_POINT('Ctrl Pts',(190.499799430221,51.6407334755141,102.335323750815));
#95908=CARTESIAN_POINT('Ctrl Pts',(190.499250292471,51.5480440363441,102.279610270829));
#95909=CARTESIAN_POINT('Ctrl Pts',(190.499515970613,51.7229179106605,102.411478309401));
#95910=CARTESIAN_POINT('Ctrl Pts',(190.49972516959,51.6156442577851,102.355567759317));
#95911=CARTESIAN_POINT('Ctrl Pts',(190.498970307289,51.5083740319849,102.299655341424));
#95912=CARTESIAN_POINT('Ctrl Pts',(190.499284059707,51.6946440831874,102.473535673214));
#95913=CARTESIAN_POINT('Ctrl Pts',(190.499498450219,51.5479726767401,102.417020913844));
#95914=CARTESIAN_POINT('Ctrl Pts',(190.498111784629,51.4013090294031,102.360502853894));
#95915=CARTESIAN_POINT('Ctrl Pts',(190.499119727676,51.6800791470945,102.517049663537));
#95916=CARTESIAN_POINT('Ctrl Pts',(190.499337816664,51.5128530332642,102.460109100771));
#95917=CARTESIAN_POINT('Ctrl Pts',(190.497498869166,51.345638318955,102.403164303197));
#95918=CARTESIAN_POINT('Ctrl Pts',(190.498618713093,51.6405359775216,102.648172265196));
#95919=CARTESIAN_POINT('Ctrl Pts',(190.498848143968,51.4171792202356,102.589942012296));
#95920=CARTESIAN_POINT('Ctrl Pts',(190.495619236823,51.1938479864711,102.531703725));
#95921=CARTESIAN_POINT('Ctrl Pts',(190.498271656209,51.6201726452936,102.737019270818));
#95922=CARTESIAN_POINT('Ctrl Pts',(190.498509029016,51.367385337178,102.677905732386));
#95923=CARTESIAN_POINT('Ctrl Pts',(190.49430319548,51.1146352450511,102.618781959713));
#95924=CARTESIAN_POINT('Ctrl Pts',(190.497201308041,51.5641115179798,103.004804782485));
#95925=CARTESIAN_POINT('Ctrl Pts',(190.497463445055,51.2295980868092,102.943002008983));
#95926=CARTESIAN_POINT('Ctrl Pts',(190.49021003554,50.8951677024927,102.881177837155));
#95927=CARTESIAN_POINT('Ctrl Pts',(190.496447643867,51.5344336039414,103.185292559695));
#95928=CARTESIAN_POINT('Ctrl Pts',(190.496727574125,51.1555210265605,103.121637703458));
#95929=CARTESIAN_POINT('Ctrl Pts',(190.487283349245,50.7767304584846,103.057955343393));
#95930=CARTESIAN_POINT('Ctrl Pts',(190.494081221756,51.4520056115398,103.727228609739));
#95931=CARTESIAN_POINT('Ctrl Pts',(190.494418228543,50.9480361132095,103.657900955732));
#95932=CARTESIAN_POINT('Ctrl Pts',(190.477971438738,50.444345763347,103.588507032427));
#95933=CARTESIAN_POINT('Ctrl Pts',(190.49235932922,51.4069351392841,104.090155717021));
#95934=CARTESIAN_POINT('Ctrl Pts',(190.492739427804,50.8318828452958,104.016865737875));
#95935=CARTESIAN_POINT('Ctrl Pts',(190.471040957409,50.2572502899628,103.943486936546));
#95936=CARTESIAN_POINT('Ctrl Pts',(190.486730141455,51.2791586543925,105.180968843957));
#95937=CARTESIAN_POINT('Ctrl Pts',(190.487257204149,50.4975091671849,105.095304416781));
#95938=CARTESIAN_POINT('Ctrl Pts',(190.447858717668,49.7168874252647,105.009386390733));
#95939=CARTESIAN_POINT('Ctrl Pts',(190.482359180188,51.2055248140897,105.911119065978));
#95940=CARTESIAN_POINT('Ctrl Pts',(190.483007695422,50.2972530200621,105.816498140453));
#95941=CARTESIAN_POINT('Ctrl Pts',(190.429230323806,49.3906083817691,105.721494395297));
#95942=CARTESIAN_POINT('Ctrl Pts',(190.472162308371,51.0626181516781,107.374691782782));
#95943=CARTESIAN_POINT('Ctrl Pts',(190.473121121834,49.8957928625997,107.260560352614));
#95944=CARTESIAN_POINT('Ctrl Pts',(190.383701752993,48.7324581795214,107.145873015116));
#95945=CARTESIAN_POINT('Ctrl Pts',(190.466335782918,50.9942518830845,108.108322244973));
#95946=CARTESIAN_POINT('Ctrl Pts',(190.467482361322,49.6966919813105,107.983721772173));
#95947=CARTESIAN_POINT('Ctrl Pts',(190.356804914099,48.4039286397594,107.858347999142));
#95948=CARTESIAN_POINT('Ctrl Pts',(190.452970899325,50.8595431134232,109.579204958687));
#95949=CARTESIAN_POINT('Ctrl Pts',(190.454586628089,49.2890216722974,109.431896793475));
#95950=CARTESIAN_POINT('Ctrl Pts',(190.292017249808,47.727047424533,109.283470480434));
#95951=CARTESIAN_POINT('Ctrl Pts',(190.445432703546,50.7933151759563,110.316467760936));
#95952=CARTESIAN_POINT('Ctrl Pts',(190.447327931139,49.0806876989918,110.15703956062));
#95953=CARTESIAN_POINT('Ctrl Pts',(190.254138221714,47.3791214038583,109.996128900898));
#95954=CARTESIAN_POINT('Ctrl Pts',(190.419816456401,50.5959796189513,112.534099894033));
#95955=CARTESIAN_POINT('Ctrl Pts',(190.422734650417,48.4315676710545,112.3360534236));
#95956=CARTESIAN_POINT('Ctrl Pts',(190.118372626102,46.2890691893423,112.134196728001));
#95957=CARTESIAN_POINT('Ctrl Pts',(190.398759656664,50.4661184136419,114.020346541584));
#95958=CARTESIAN_POINT('Ctrl Pts',(190.402589209194,47.966636367364,113.793361990212));
#95959=CARTESIAN_POINT('Ctrl Pts',(189.999306492312,45.5003667299309,113.559765336211));
#95960=CARTESIAN_POINT('Ctrl Pts',(190.359096412405,50.2726331003764,116.263830002808));
#95961=CARTESIAN_POINT('Ctrl Pts',(190.365014333285,47.1893016369557,115.984297698539));
#95962=CARTESIAN_POINT('Ctrl Pts',(189.741113284684,44.1704053032068,115.697893892108));
#95963=CARTESIAN_POINT('Ctrl Pts',(190.34452459809,50.2084149184493,117.013959238553));
#95964=CARTESIAN_POINT('Ctrl Pts',(190.351237949028,46.9164429231363,116.71648393922));
#95965=CARTESIAN_POINT('Ctrl Pts',(189.641525718368,43.7026480635995,116.410512021392));
#95966=CARTESIAN_POINT('Ctrl Pts',(190.31224902198,50.0806483650631,118.519403304998));
#95967=CARTESIAN_POINT('Ctrl Pts',(190.320859208328,46.3399940246239,118.183416722279));
#95968=CARTESIAN_POINT('Ctrl Pts',(189.406807784642,42.7138690255277,117.835543719062));
#95969=CARTESIAN_POINT('Ctrl Pts',(190.294545716396,50.0171081032886,119.274717542161));
#95970=CARTESIAN_POINT('Ctrl Pts',(190.304243560584,46.0360189897018,118.918579936746));
#95971=CARTESIAN_POINT('Ctrl Pts',(189.271522379414,42.1925277014723,118.547958266628));
#95972=CARTESIAN_POINT('Ctrl Pts',(190.255510033889,49.8907533419771,120.791203382157));
#95973=CARTESIAN_POINT('Ctrl Pts',(190.267779575357,45.3981681971246,120.391919060921));
#95974=CARTESIAN_POINT('Ctrl Pts',(188.957866276243,41.1027212910509,119.972550354973));
#95975=CARTESIAN_POINT('Ctrl Pts',(190.234178228885,49.8279470556339,121.552374076106));
#95976=CARTESIAN_POINT('Ctrl Pts',(190.247911663905,45.0638991441457,121.130595534004));
#95977=CARTESIAN_POINT('Ctrl Pts',(188.779250264425,40.5341155190546,120.684728907705));
#95978=CARTESIAN_POINT('Ctrl Pts',(190.187306873929,49.7027878508555,123.081327471884));
#95979=CARTESIAN_POINT('Ctrl Pts',(190.204468021955,44.3763011076148,122.611515499938));
#95980=CARTESIAN_POINT('Ctrl Pts',(188.378856035911,39.3756582923654,122.108773106394));
#95981=CARTESIAN_POINT('Ctrl Pts',(190.161768087685,49.6404349854971,123.84910806775));
#95982=CARTESIAN_POINT('Ctrl Pts',(190.180866911108,44.023010216783,123.3542529677));
#95983=CARTESIAN_POINT('Ctrl Pts',(188.157139850915,38.7864955565338,122.820638866055));
#95984=CARTESIAN_POINT('Ctrl Pts',(190.105804470716,49.5154258447559,125.392126822043));
#95985=CARTESIAN_POINT('Ctrl Pts',(190.129396822592,43.3164757243997,124.843934539981));
#95986=CARTESIAN_POINT('Ctrl Pts',(187.682431381576,37.6261436339848,124.243917236916));
#95987=CARTESIAN_POINT('Ctrl Pts',(190.075380715705,49.4527600253111,126.167361462351));
#95988=CARTESIAN_POINT('Ctrl Pts',(190.101500176494,42.9634678383499,125.591245111377));
#95989=CARTESIAN_POINT('Ctrl Pts',(187.429845353543,37.0556750039611,124.955328797435));
#95990=CARTESIAN_POINT('Ctrl Pts',(190.008843987008,49.3260415780364,127.726281125232));
#95991=CARTESIAN_POINT('Ctrl Pts',(190.040788198983,42.2719768330555,127.090804150198));
#95992=CARTESIAN_POINT('Ctrl Pts',(186.909282058273,35.9593595880391,126.377509295516));
#95993=CARTESIAN_POINT('Ctrl Pts',(189.972732501654,49.2619815486278,128.509962500036));
#95994=CARTESIAN_POINT('Ctrl Pts',(190.007946445721,41.9334210799763,127.84325017495));
#95995=CARTESIAN_POINT('Ctrl Pts',(186.64145632905,35.4333468604082,127.08827735133));
#95996=CARTESIAN_POINT('Ctrl Pts',(189.854418466984,49.0660570573506,130.875521988522));
#95997=CARTESIAN_POINT('Ctrl Pts',(189.900690411698,40.9424772204947,130.114102894018));
#95998=CARTESIAN_POINT('Ctrl Pts',(185.829257275597,33.9285810406561,129.219310893706));
#95999=CARTESIAN_POINT('Ctrl Pts',(189.762383383776,48.9303940639483,132.471700290503));
#96000=CARTESIAN_POINT('Ctrl Pts',(189.817923043442,40.3196344184964,131.636603424624));
#96001=CARTESIAN_POINT('Ctrl Pts',(185.277674642686,33.0230795598244,130.638306254556));
#96002=CARTESIAN_POINT('Ctrl Pts',(189.541450758005,48.6413779255017,135.716703876259));
#96003=CARTESIAN_POINT('Ctrl Pts',(189.622302528065,39.1154704613994,134.713814310541));
#96004=CARTESIAN_POINT('Ctrl Pts',(184.16314166873,31.343059040108,133.471278688383));
#96005=CARTESIAN_POINT('Ctrl Pts',(189.412696565286,48.4880858492789,137.365316901128));
#96006=CARTESIAN_POINT('Ctrl Pts',(189.509253756171,38.5332826287984,136.268745748172));
#96007=CARTESIAN_POINT('Ctrl Pts',(183.598718362169,30.5665275759884,134.885267769976));
#96008=CARTESIAN_POINT('Ctrl Pts',(189.101617591595,48.15693255634,140.73916716681));
#96009=CARTESIAN_POINT('Ctrl Pts',(189.241776478868,37.3725240109737,139.426916956348));
#96010=CARTESIAN_POINT('Ctrl Pts',(182.436006440891,29.0794895646531,137.706412840331));
#96011=CARTESIAN_POINT('Ctrl Pts',(188.91966300801,47.9791445996723,142.463861098625));
#96012=CARTESIAN_POINT('Ctrl Pts',(189.087110147823,36.7940512823183,141.030628638056));
#96013=CARTESIAN_POINT('Ctrl Pts',(181.837626822499,28.3693117365578,139.113588019648));
#96014=CARTESIAN_POINT('Ctrl Pts',(188.47229553167,47.5907621638428,146.033790251501));
#96015=CARTESIAN_POINT('Ctrl Pts',(188.717853953436,35.6098041142205,144.31641474328));
#96016=CARTESIAN_POINT('Ctrl Pts',(180.578988811759,26.9735714770137,141.918640354836));
#96017=CARTESIAN_POINT('Ctrl Pts',(188.208103854505,47.3803127607776,147.87729610845));
#96018=CARTESIAN_POINT('Ctrl Pts',(188.503079327534,35.0038658683449,145.999240295164));
#96019=CARTESIAN_POINT('Ctrl Pts',(179.919133224523,26.2884818917448,143.316561676331));
#96020=CARTESIAN_POINT('Ctrl Pts',(187.701708797589,47.0306444895355,150.802754104872));
#96021=CARTESIAN_POINT('Ctrl Pts',(188.110337479306,34.0490845545101,148.624600476526));
#96022=CARTESIAN_POINT('Ctrl Pts',(178.852766970947,25.2531568776001,145.403494991665));
#96023=CARTESIAN_POINT('Ctrl Pts',(187.5142585255,46.9083821641599,151.805049241076));
#96024=CARTESIAN_POINT('Ctrl Pts',(187.966748913229,33.721575883887,149.521043140327));
#96025=CARTESIAN_POINT('Ctrl Pts',(178.484425597357,24.9067806771726,146.097467019026));
#96026=CARTESIAN_POINT('Ctrl Pts',(187.084961282489,46.6498692416155,153.888493688112));
#96027=CARTESIAN_POINT('Ctrl Pts',(187.646445162211,33.0425327417734,151.368871051823));
#96028=CARTESIAN_POINT('Ctrl Pts',(177.713935688162,24.2062418677873,147.481240380467));
#96029=CARTESIAN_POINT('Ctrl Pts',(186.84356384104,46.5136513094283,154.969065472559));
#96030=CARTESIAN_POINT('Ctrl Pts',(187.469619298187,32.6907847434722,152.320710176512));
#96031=CARTESIAN_POINT('Ctrl Pts',(177.311884861241,23.8521344999142,148.171051695706));
#96032=CARTESIAN_POINT('Ctrl Pts',(186.274665703984,46.2233074742099,157.253389244316));
#96033=CARTESIAN_POINT('Ctrl Pts',(187.067385185671,31.9509244222017,154.312403060988));
#96034=CARTESIAN_POINT('Ctrl Pts',(176.461891719931,23.1291070452778,149.545249180182));
#96035=CARTESIAN_POINT('Ctrl Pts',(185.948755193325,46.0692730647339,158.455223543716));
#96036=CARTESIAN_POINT('Ctrl Pts',(186.842064169064,31.5626244001255,155.352420003862));
#96037=CARTESIAN_POINT('Ctrl Pts',(176.014221907291,22.7603385409926,150.229663071457));
#96038=CARTESIAN_POINT('Ctrl Pts',(185.341105577039,45.8195993055715,160.422578369751));
#96039=CARTESIAN_POINT('Ctrl Pts',(186.443675283611,30.9354856298111,157.030413584589));
#96040=CARTESIAN_POINT('Ctrl Pts',(175.292466123159,22.1873888600896,151.25057226375));
#96041=CARTESIAN_POINT('Ctrl Pts',(185.11820009744,45.7332168496864,161.106542537928));
#96042=CARTESIAN_POINT('Ctrl Pts',(186.29997071828,30.7179737283957,157.612199178184));
#96043=CARTESIAN_POINT('Ctrl Pts',(175.043347033158,21.9930297124899,151.589912581918));
#96044=CARTESIAN_POINT('Ctrl Pts',(184.616759767744,45.5544782741863,162.541567503122));
#96045=CARTESIAN_POINT('Ctrl Pts',(185.986027899374,30.2653381771069,158.825495053442));
#96046=CARTESIAN_POINT('Ctrl Pts',(174.528782445827,21.5990339634757,152.259669539456));
#96047=CARTESIAN_POINT('Ctrl Pts',(184.338298824303,45.4619607004085,163.293528615471));
#96048=CARTESIAN_POINT('Ctrl Pts',(185.815468705345,30.0296558164555,159.45843675178));
#96049=CARTESIAN_POINT('Ctrl Pts',(174.262870297413,21.3990136510515,152.590829373774));
#96050=CARTESIAN_POINT('Ctrl Pts',(183.690939071064,45.2690280167149,164.905619500582));
#96051=CARTESIAN_POINT('Ctrl Pts',(185.433213803636,29.5303219098013,160.807765819904));
#96052=CARTESIAN_POINT('Ctrl Pts',(173.708825716552,20.9902993513571,153.24381452559));
#96053=CARTESIAN_POINT('Ctrl Pts',(183.323597110923,45.1686445967153,165.764429148084));
#96054=CARTESIAN_POINT('Ctrl Pts',(185.22166924195,29.2666120232491,161.524194287642));
#96055=CARTESIAN_POINT('Ctrl Pts',(173.420787378789,20.7816581703162,153.565674560105));
#96056=CARTESIAN_POINT('Ctrl Pts',(182.647456403272,45.0101079286491,167.193151066404));
#96057=CARTESIAN_POINT('Ctrl Pts',(184.850837725503,28.8354472440965,162.71011232814));
#96058=CARTESIAN_POINT('Ctrl Pts',(172.965820078663,20.4588438804909,154.039099832331));
#96059=CARTESIAN_POINT('Ctrl Pts',(182.4008106133,44.9559247402993,167.693223955363));
#96060=CARTESIAN_POINT('Ctrl Pts',(184.717658151634,28.6851618676557,163.125789683885));
#96061=CARTESIAN_POINT('Ctrl Pts',(172.810312765267,20.3495787812123,154.195335097582));
#96062=CARTESIAN_POINT('Ctrl Pts',(181.844224354564,44.8443052620572,168.760246115741));
#96063=CARTESIAN_POINT('Ctrl Pts',(184.424357870275,28.3667030054888,164.013312964699));
#96064=CARTESIAN_POINT('Ctrl Pts',(172.489839921108,20.1267742123925,154.504000559469));
#96065=CARTESIAN_POINT('Ctrl Pts',(181.534618839301,44.7868741449486,169.327084815468));
#96066=CARTESIAN_POINT('Ctrl Pts',(184.26415365177,28.1984160514982,164.485572835663));
#96067=CARTESIAN_POINT('Ctrl Pts',(172.324889664599,20.0132431244623,154.656436448801));
#96068=CARTESIAN_POINT('Ctrl Pts',(180.816015283947,44.6679012328639,170.557089813402));
#96069=CARTESIAN_POINT('Ctrl Pts',(183.901791939756,27.8344037889279,165.514854559176));
#96070=CARTESIAN_POINT('Ctrl Pts',(171.982933620113,19.7804856361125,154.956532274931));
#96071=CARTESIAN_POINT('Ctrl Pts',(180.404978491179,44.606095409884,171.22402034852));
#96072=CARTESIAN_POINT('Ctrl Pts',(183.698284469547,27.6374346411265,166.075913204549));
#96073=CARTESIAN_POINT('Ctrl Pts',(171.805167736614,19.660753182185,155.104786004147));
#96074=CARTESIAN_POINT('Ctrl Pts',(179.676788347291,44.5104783181643,172.310866493804));
#96075=CARTESIAN_POINT('Ctrl Pts',(183.346182791328,27.3133423187831,166.999982185387));
#96076=CARTESIAN_POINT('Ctrl Pts',(171.529838730185,19.4774729604571,155.319896659783));
#96077=CARTESIAN_POINT('Ctrl Pts',(179.41543002632,44.4781344195113,172.68732829295));
#96078=CARTESIAN_POINT('Ctrl Pts',(183.220557062346,27.2001673966544,167.322714587353));
#96079=CARTESIAN_POINT('Ctrl Pts',(171.436652942884,19.4157890822098,155.390365310602));
#96080=CARTESIAN_POINT('Ctrl Pts',(178.849564583556,44.4123980422603,173.467349740303));
#96081=CARTESIAN_POINT('Ctrl Pts',(182.950138463494,26.9622256484572,167.997886625965));
#96082=CARTESIAN_POINT('Ctrl Pts',(171.247132785599,19.291074681691,155.528562264384));
#96083=CARTESIAN_POINT('Ctrl Pts',(178.544828026528,44.379004547457,173.871097732987));
#96084=CARTESIAN_POINT('Ctrl Pts',(182.805119762423,26.8373005774686,168.350789186519));
#96085=CARTESIAN_POINT('Ctrl Pts',(171.150795263472,19.228042132856,155.596288273887));
#96086=CARTESIAN_POINT('Ctrl Pts',(177.891978896762,44.311076287452,174.695871921722));
#96087=CARTESIAN_POINT('Ctrl Pts',(182.494224696965,26.5751718520979,169.081599863043));
#96088=CARTESIAN_POINT('Ctrl Pts',(170.954677195547,19.1004973565966,155.728748553708));
#96089=CARTESIAN_POINT('Ctrl Pts',(177.54370604816,44.2765399816905,175.116859637631));
#96090=CARTESIAN_POINT('Ctrl Pts',(182.328105345844,26.4378064245884,169.459826151321));
#96091=CARTESIAN_POINT('Ctrl Pts',(170.854891970795,19.0359822946474,155.793479304452));
#96092=CARTESIAN_POINT('Ctrl Pts',(176.816454914454,44.2062878499871,175.953808795454));
#96093=CARTESIAN_POINT('Ctrl Pts',(181.977837333457,26.1530991582133,170.225223838092));
#96094=CARTESIAN_POINT('Ctrl Pts',(170.651744296242,18.9054504576405,155.919809151524));
#96095=CARTESIAN_POINT('Ctrl Pts',(176.437805815838,44.1705713626272,176.369252899516));
#96096=CARTESIAN_POINT('Ctrl Pts',(181.79364300311,26.0057327649136,170.612157232357));
#96097=CARTESIAN_POINT('Ctrl Pts',(170.548379957486,18.8394328302813,155.981406632915));
#96098=CARTESIAN_POINT('Ctrl Pts',(175.67416196717,44.0980156569334,177.168406531664));
#96099=CARTESIAN_POINT('Ctrl Pts',(181.415109475414,25.7064830072658,171.371918912357));
#96100=CARTESIAN_POINT('Ctrl Pts',(170.338218421151,18.7060526535118,156.101533098092));
#96101=CARTESIAN_POINT('Ctrl Pts',(175.289646799165,44.0611777276179,177.551758007294));
#96102=CARTESIAN_POINT('Ctrl Pts',(181.220896603426,25.5546901009831,171.744319900801));
#96103=CARTESIAN_POINT('Ctrl Pts',(170.231425117911,18.6386929030414,156.160064719042));
#96104=CARTESIAN_POINT('Ctrl Pts',(174.535877481548,43.9865237830416,178.271798574629));
#96105=CARTESIAN_POINT('Ctrl Pts',(180.830591057864,25.2520703105088,172.458763603975));
#96106=CARTESIAN_POINT('Ctrl Pts',(170.014802174258,18.5029361223571,156.274313806325));
#96107=CARTESIAN_POINT('Ctrl Pts',(174.166661263537,43.9487095499583,178.608658923048));
#96108=CARTESIAN_POINT('Ctrl Pts',(180.634570310566,25.1013021558804,172.800659261218));
#96109=CARTESIAN_POINT('Ctrl Pts',(169.904977694101,18.4345424558401,156.330034996734));
#96110=CARTESIAN_POINT('Ctrl Pts',(173.096395080678,43.8340694277073,179.549104938071));
#96111=CARTESIAN_POINT('Ctrl Pts',(180.049380177025,24.6539596786527,173.776866319289));
#96112=CARTESIAN_POINT('Ctrl Pts',(169.571687500788,18.2283337795665,156.493479970059));
#96113=CARTESIAN_POINT('Ctrl Pts',(172.433943023058,43.7560611973564,180.082861701901));
#96114=CARTESIAN_POINT('Ctrl Pts',(179.666916997985,24.3652485690659,174.355239609894));
#96115=CARTESIAN_POINT('Ctrl Pts',(169.344451316501,18.089526387521,156.597515025505));
#96116=CARTESIAN_POINT('Ctrl Pts',(171.205786180245,43.5981266073985,181.019825600731));
#96117=CARTESIAN_POINT('Ctrl Pts',(178.920970523949,23.8083509956536,175.403059117497));
#96118=CARTESIAN_POINT('Ctrl Pts',(168.883249062146,17.8115169098302,156.798103910025));
#96119=CARTESIAN_POINT('Ctrl Pts',(170.637157103811,43.518029497162,181.424897130365));
#96120=CARTESIAN_POINT('Ctrl Pts',(178.556708868383,23.5397308935891,175.873065324021));
#96121=CARTESIAN_POINT('Ctrl Pts',(168.648778846346,17.6720218607262,156.89483965041));
#96122=CARTESIAN_POINT('Ctrl Pts',(169.577125502554,43.3582879379689,182.146828667796));
#96123=CARTESIAN_POINT('Ctrl Pts',(177.848422670943,23.0239393013448,176.731949074881));
#96124=CARTESIAN_POINT('Ctrl Pts',(168.179817243338,17.3966478726328,157.080712120593));
#96125=CARTESIAN_POINT('Ctrl Pts',(169.084091674877,43.2784719370058,182.46462633532));
#96126=CARTESIAN_POINT('Ctrl Pts',(177.503993626021,22.776498051728,177.121003860235));
#96127=CARTESIAN_POINT('Ctrl Pts',(167.944828417653,17.2604584461382,157.170067976753));
#96128=CARTESIAN_POINT('Ctrl Pts',(168.149706837097,43.11926457637,183.044103788451));
#96129=CARTESIAN_POINT('Ctrl Pts',(176.828250555667,22.2975347205762,177.844722410507));
#96130=CARTESIAN_POINT('Ctrl Pts',(167.474607120963,16.9913843688579,157.343134967837));
#96131=CARTESIAN_POINT('Ctrl Pts',(167.708474202632,43.0398707539592,183.305509411467));
#96132=CARTESIAN_POINT('Ctrl Pts',(176.497339532542,22.0663379064465,178.178536418142));
#96133=CARTESIAN_POINT('Ctrl Pts',(167.239368096194,16.8584950715248,157.426836570331));
#96134=CARTESIAN_POINT('Ctrl Pts',(166.441269532885,42.8026077754189,184.030870841384));
#96135=CARTESIAN_POINT('Ctrl Pts',(175.516740453347,21.3907448714663,179.122298645269));
#96136=CARTESIAN_POINT('Ctrl Pts',(166.533930460771,16.4649162452889,157.6709545235));
#96137=CARTESIAN_POINT('Ctrl Pts',(165.67057063508,42.645672122449,184.437373448117));
#96138=CARTESIAN_POINT('Ctrl Pts',(174.88514165464,20.9686022770523,179.668954321226));
#96139=CARTESIAN_POINT('Ctrl Pts',(166.064053906251,16.2093368164217,157.824459871347));
#96140=CARTESIAN_POINT('Ctrl Pts',(164.215189634904,42.3350660712107,185.165802042391));
#96141=CARTESIAN_POINT('Ctrl Pts',(173.644088953391,20.1618031972738,180.668647973063));
#96142=CARTESIAN_POINT('Ctrl Pts',(165.126741222935,15.7114345690758,158.117870390187));
#96143=CARTESIAN_POINT('Ctrl Pts',(163.531436677291,42.1813820193468,185.486483517213));
#96144=CARTESIAN_POINT('Ctrl Pts',(173.03620986103,19.7783760162525,181.118882320385));
#96145=CARTESIAN_POINT('Ctrl Pts',(164.659269936658,15.469088732046,158.257721966292));
#96146=CARTESIAN_POINT('Ctrl Pts',(162.220881816397,41.8775725051339,186.072809112622));
#96147=CARTESIAN_POINT('Ctrl Pts',(171.836140271617,19.0417666288641,181.953923628036));
#96148=CARTESIAN_POINT('Ctrl Pts',(163.727189231406,14.9967277807032,158.526558693323));
#96149=CARTESIAN_POINT('Ctrl Pts',(161.594416787495,41.7274416157552,186.338050141004));
#96150=CARTESIAN_POINT('Ctrl Pts',(171.244906300323,18.6893215198367,182.337382834772));
#96151=CARTESIAN_POINT('Ctrl Pts',(163.262566911235,14.7667051884807,158.65552280578));
#96152=CARTESIAN_POINT('Ctrl Pts',(160.381684956782,41.4308406296666,186.829865947347));
#96153=CARTESIAN_POINT('Ctrl Pts',(170.074501642088,18.0098120898375,183.055472768792));
#96154=CARTESIAN_POINT('Ctrl Pts',(162.336204079231,14.3179948881814,158.904394050565));
#96155=CARTESIAN_POINT('Ctrl Pts',(159.795558975426,41.2843680069152,187.056283248367));
#96156=CARTESIAN_POINT('Ctrl Pts',(169.495983674241,17.6832380393579,183.389338243258));
#96157=CARTESIAN_POINT('Ctrl Pts',(161.874458194339,14.0993047060754,159.024291458785));
#96158=CARTESIAN_POINT('Ctrl Pts',(158.081766525943,40.850451543292,187.692431197991));
#96159=CARTESIAN_POINT('Ctrl Pts',(167.771142741458,16.734066698008,184.335884123339));
#96160=CARTESIAN_POINT('Ctrl Pts',(160.493316742373,13.4588151165262,159.372323641613));
#96161=CARTESIAN_POINT('Ctrl Pts',(156.996151795608,40.5680775459283,188.060383044538));
#96162=CARTESIAN_POINT('Ctrl Pts',(166.644152309164,16.1471188061287,184.888549532335));
#96163=CARTESIAN_POINT('Ctrl Pts',(159.576564432943,13.0519322694405,159.589213106444));
#96164=CARTESIAN_POINT('Ctrl Pts',(154.902062387963,40.0195872766128,188.724538486421));
#96165=CARTESIAN_POINT('Ctrl Pts',(164.425531251345,15.0434942821473,185.891220463642));
#96166=CARTESIAN_POINT('Ctrl Pts',(157.758927004785,12.2759631210897,159.997426329598));
#96167=CARTESIAN_POINT('Ctrl Pts',(153.896877076874,39.7541702385511,189.019386070661));
#96168=CARTESIAN_POINT('Ctrl Pts',(163.339462148368,14.5299347015406,186.337660838382));
#96169=CARTESIAN_POINT('Ctrl Pts',(156.860464559164,11.9078480940796,160.188200885041));
#96170=CARTESIAN_POINT('Ctrl Pts',(151.941670484102,39.2392317495092,189.559159111861));
#96171=CARTESIAN_POINT('Ctrl Pts',(161.20045577941,13.560445138601,187.1554296739));
#96172=CARTESIAN_POINT('Ctrl Pts',(155.080186035148,11.2043865044206,160.548546057543));
#96173=CARTESIAN_POINT('Ctrl Pts',(150.992079329702,38.9897469154245,189.803781241461));
#96174=CARTESIAN_POINT('Ctrl Pts',(160.149374965747,13.1056749038428,187.525391586376));
#96175=CARTESIAN_POINT('Ctrl Pts',(154.198401648731,10.8690713312607,160.71807822485));
#96176=CARTESIAN_POINT('Ctrl Pts',(150.061838982486,38.7473935021229,190.030202679682));
#96177=CARTESIAN_POINT('Ctrl Pts',(159.114345837254,12.6753117645545,187.866263775242));
#96178=CARTESIAN_POINT('Ctrl Pts',(153.323364948845,10.5475610359161,160.878837531617));
#96179=CARTESIAN_POINT('',(190.499797482064,51.8013867006573,102.335336081514));
#96180=CARTESIAN_POINT('Ctrl Pts',(151.26536469753,39.0180386085743,189.729482705023));
#96181=CARTESIAN_POINT('Ctrl Pts',(152.311979458206,39.2925615430878,189.460998195749));
#96182=CARTESIAN_POINT('Ctrl Pts',(153.355186189874,39.5681010168028,189.174926079119));
#96183=CARTESIAN_POINT('Ctrl Pts',(155.434778870331,40.1162070651496,188.561125057896));
#96184=CARTESIAN_POINT('Ctrl Pts',(156.473210242748,40.3893067764282,188.232684087622));
#96185=CARTESIAN_POINT('Ctrl Pts',(159.560122787503,41.1893291647367,187.178921311955));
#96186=CARTESIAN_POINT('Ctrl Pts',(161.580064916327,41.6970588940589,186.386530151768));
#96187=CARTESIAN_POINT('Ctrl Pts',(165.526821722319,42.5922403987276,184.555727820473));
#96188=CARTESIAN_POINT('Ctrl Pts',(167.454218150135,42.9769238346723,183.517277705224));
#96189=CARTESIAN_POINT('Ctrl Pts',(170.249726424738,43.4291995534616,181.706506578626));
#96190=CARTESIAN_POINT('Ctrl Pts',(171.170073214828,43.5601865679599,181.056506878982));
#96191=CARTESIAN_POINT('Ctrl Pts',(172.935023625514,43.7831597459461,179.688354836545));
#96192=CARTESIAN_POINT('Ctrl Pts',(173.782417537072,43.8759288508816,178.968977104368));
#96193=CARTESIAN_POINT('Ctrl Pts',(176.214153740203,44.1226926454971,176.702601166982));
#96194=CARTESIAN_POINT('Ctrl Pts',(177.687043857519,44.247660840443,175.046670319815));
#96195=CARTESIAN_POINT('Ctrl Pts',(179.337557075668,44.4366493823772,172.799184311615));
#96196=CARTESIAN_POINT('Ctrl Pts',(179.658204132338,44.4759149514855,172.340861046938));
#96197=CARTESIAN_POINT('Ctrl Pts',(180.280752658175,44.5585643046451,171.406844757758));
#96198=CARTESIAN_POINT('Ctrl Pts',(180.582966807554,44.602014713882,170.930523914811));
#96199=CARTESIAN_POINT('Ctrl Pts',(181.45383672706,44.7382868762494,169.49003443454));
#96200=CARTESIAN_POINT('Ctrl Pts',(181.989702502981,44.8375345369766,168.51017247428));
#96201=CARTESIAN_POINT('Ctrl Pts',(183.479269028008,45.160389197305,165.519349529815));
#96202=CARTESIAN_POINT('Ctrl Pts',(184.315468338622,45.4093716649899,163.457423617314));
#96203=CARTESIAN_POINT('Ctrl Pts',(185.391987364775,45.807605610716,160.285891280647));
#96204=CARTESIAN_POINT('Ctrl Pts',(185.720583246987,45.9442010673929,159.21642893812));
#96205=CARTESIAN_POINT('Ctrl Pts',(186.320700873814,46.2176663718146,157.077876486429));
#96206=CARTESIAN_POINT('Ctrl Pts',(186.593330143435,46.3549283352379,156.005610616448));
#96207=CARTESIAN_POINT('Ctrl Pts',(187.34307110056,46.763277222671,152.78090583539));
#96208=CARTESIAN_POINT('Ctrl Pts',(187.752691172238,47.0305111914563,150.620590465638));
#96209=CARTESIAN_POINT('Ctrl Pts',(188.446157287329,47.5399101689615,146.283476114733));
#96210=CARTESIAN_POINT('Ctrl Pts',(188.729706086305,47.7822397640886,144.106660767897));
#96211=CARTESIAN_POINT('Ctrl Pts',(189.207183080785,48.2381611353919,139.74018708407));
#96212=CARTESIAN_POINT('Ctrl Pts',(189.400945395645,48.4517916420194,137.550514252977));
#96213=CARTESIAN_POINT('Ctrl Pts',(189.724147979183,48.8542816387485,133.161532602988));
#96214=CARTESIAN_POINT('Ctrl Pts',(189.853490061688,49.0429920619039,130.962197846555));
#96215=CARTESIAN_POINT('Ctrl Pts',(190.066046457663,49.40875100006,126.557233882612));
#96216=CARTESIAN_POINT('Ctrl Pts',(190.149197206518,49.5864981643842,124.35166813467));
#96217=CARTESIAN_POINT('Ctrl Pts',(190.282774616374,49.9515269587546,119.937868461153));
#96218=CARTESIAN_POINT('Ctrl Pts',(190.333166891757,50.1388961726539,117.729639560238));
#96219=CARTESIAN_POINT('Ctrl Pts',(190.411306967085,50.5223284935433,113.311546989386));
#96220=CARTESIAN_POINT('Ctrl Pts',(190.439016042554,50.7163027287905,111.102262196733));
#96221=CARTESIAN_POINT('Ctrl Pts',(190.469287350292,51.0207096976079,107.789673661224));
#96222=CARTESIAN_POINT('Ctrl Pts',(190.477479042423,51.1237807501464,106.685603953041));
#96223=CARTESIAN_POINT('Ctrl Pts',(190.487498953076,51.2962699272586,105.031116633254));
#96224=CARTESIAN_POINT('Ctrl Pts',(190.4904598684,51.3562576700685,104.47989406235));
#96225=CARTESIAN_POINT('Ctrl Pts',(190.494393761014,51.4628762247885,103.65518540443));
#96226=CARTESIAN_POINT('Ctrl Pts',(190.495620626626,51.5008184630458,103.380585399644));
#96227=CARTESIAN_POINT('Ctrl Pts',(190.497338199613,51.5713767347022,102.970407234778));
#96228=CARTESIAN_POINT('Ctrl Pts',(190.497889660856,51.5968666250794,102.834097086841));
#96229=CARTESIAN_POINT('Ctrl Pts',(190.498680294458,51.6455604475564,102.63201300199));
#96230=CARTESIAN_POINT('Ctrl Pts',(190.498938602068,51.6633593134969,102.564820245953));
#96231=CARTESIAN_POINT('Ctrl Pts',(190.499310561813,51.6980708668151,102.466436119011));
#96232=CARTESIAN_POINT('Ctrl Pts',(190.499431569571,51.7107691530297,102.434144296921));
#96233=CARTESIAN_POINT('Ctrl Pts',(190.499602005233,51.7356544621898,102.388309768035));
#96234=CARTESIAN_POINT('Ctrl Pts',(190.499657802637,51.7450073320729,102.373238940239));
#96235=CARTESIAN_POINT('Ctrl Pts',(190.499753774817,51.7683402146372,102.34723353356));
#96236=CARTESIAN_POINT('Ctrl Pts',(190.499797482064,51.7835531522669,102.3353360815));
#96237=CARTESIAN_POINT('Ctrl Pts',(190.499797482064,51.8013867006573,102.335336081514));
#96238=CARTESIAN_POINT('Ctrl Pts',(154.442742286491,25.4284918940193,185.219477651462));
#96239=CARTESIAN_POINT('Ctrl Pts',(155.25456339184,25.4219089188872,184.847447378001));
#96240=CARTESIAN_POINT('Ctrl Pts',(156.059626688009,25.4153258334577,184.457936844013));
#96241=CARTESIAN_POINT('Ctrl Pts',(157.654842582912,25.4021882974927,183.640346053175));
#96242=CARTESIAN_POINT('Ctrl Pts',(158.443529931846,25.3956457653571,183.21290121233));
#96243=CARTESIAN_POINT('Ctrl Pts',(160.764687787038,25.3762759136631,181.879229353496));
#96244=CARTESIAN_POINT('Ctrl Pts',(162.258407229187,25.3636567477705,180.918818281769));
#96245=CARTESIAN_POINT('Ctrl Pts',(165.122650460426,25.3392714587578,178.834487770115));
#96246=CARTESIAN_POINT('Ctrl Pts',(166.493313761037,25.3275024335347,177.710753515211));
#96247=CARTESIAN_POINT('Ctrl Pts',(168.440743116212,25.3107129547371,175.881059878429));
#96248=CARTESIAN_POINT('Ctrl Pts',(169.071734366144,25.3052609475703,175.247070171405));
#96249=CARTESIAN_POINT('Ctrl Pts',(170.293644774771,25.2946997332868,173.92590533392));
#96250=CARTESIAN_POINT('Ctrl Pts',(170.880307363561,25.2896272886514,173.242999300009));
#96251=CARTESIAN_POINT('Ctrl Pts',(172.548007721856,25.2752507069752,171.142925705269));
#96252=CARTESIAN_POINT('Ctrl Pts',(173.54407194752,25.2667550967002,169.667567264653));
#96253=CARTESIAN_POINT('Ctrl Pts',(174.844336948799,25.2558838450969,167.328403359915));
#96254=CARTESIAN_POINT('Ctrl Pts',(175.24527787866,25.2525778363154,166.527546788028));
#96255=CARTESIAN_POINT('Ctrl Pts',(175.794514753496,25.2478415600948,165.29231347852));
#96256=CARTESIAN_POINT('Ctrl Pts',(175.968732185778,25.2462958959865,164.87510964052));
#96257=CARTESIAN_POINT('Ctrl Pts',(176.296234803807,25.2432032648891,164.037870148976));
#96258=CARTESIAN_POINT('Ctrl Pts',(176.449996680554,25.2416509109389,163.616789191854));
#96259=CARTESIAN_POINT('Ctrl Pts',(177.170688179857,25.2336053720658,161.499530229832));
#96260=CARTESIAN_POINT('Ctrl Pts',(177.591573404014,25.2258451067606,159.767375049538));
#96261=CARTESIAN_POINT('Ctrl Pts',(178.209179105645,25.2074249258181,156.247847451973));
#96262=CARTESIAN_POINT('Ctrl Pts',(178.407949493929,25.1970961265605,154.457387616557));
#96263=CARTESIAN_POINT('Ctrl Pts',(178.535788240059,25.1869009068823,152.663678496546));
#96264=CARTESIAN_POINT('',(190.5,51.8013867006572,102.225104347683));
#96265=CARTESIAN_POINT('Ctrl Pts',(190.5,51.8013867006572,102.225104347683));
#96266=CARTESIAN_POINT('Ctrl Pts',(190.5,51.7819061888801,102.225107030451));
#96267=CARTESIAN_POINT('Ctrl Pts',(190.499987805158,51.7635986709013,102.226005968592));
#96268=CARTESIAN_POINT('Ctrl Pts',(190.499965895733,51.7462663363356,102.227616117064));
#96269=CARTESIAN_POINT('Ctrl Pts',(190.499940589854,51.7262470993417,102.229475874832));
#96270=CARTESIAN_POINT('Ctrl Pts',(190.499902299865,51.7075287120045,102.232286246869));
#96271=CARTESIAN_POINT('Ctrl Pts',(190.49985447553,51.6898704822393,102.235789048991));
#96272=CARTESIAN_POINT('Ctrl Pts',(190.499808728661,51.6729793172492,102.239139691118));
#96273=CARTESIAN_POINT('Ctrl Pts',(190.499754222189,51.6570599065149,102.243126566931));
#96274=CARTESIAN_POINT('Ctrl Pts',(190.499694135448,51.6419407404168,102.247511091656));
#96275=CARTESIAN_POINT('Ctrl Pts',(190.499639836321,51.6282778672001,102.251473294667));
#96276=CARTESIAN_POINT('Ctrl Pts',(190.499580960819,51.6152697582099,102.255761680282));
#96277=CARTESIAN_POINT('Ctrl Pts',(190.49952034789,51.6028024249967,102.260162820708));
#96278=CARTESIAN_POINT('Ctrl Pts',(190.499513887304,51.6014735618565,102.260631927708));
#96279=CARTESIAN_POINT('Ctrl Pts',(190.499507407636,51.6001508455561,102.261102265943));
#96280=CARTESIAN_POINT('Ctrl Pts',(190.499500912834,51.5988341389355,102.2615735385));
#96281=CARTESIAN_POINT('Ctrl Pts',(190.499435796719,51.5856329951794,102.266298461019));
#96282=CARTESIAN_POINT('Ctrl Pts',(190.499367209565,51.5728858133411,102.271265386069));
#96283=CARTESIAN_POINT('Ctrl Pts',(190.499294966487,51.5604980579874,102.276487402146));
#96284=CARTESIAN_POINT('Ctrl Pts',(190.499245073007,51.5519426609412,102.280093900632));
#96285=CARTESIAN_POINT('Ctrl Pts',(190.49919088718,51.5431272533784,102.284000583904));
#96286=CARTESIAN_POINT('Ctrl Pts',(190.499132702827,51.5341865318516,102.288183180012));
#96287=CARTESIAN_POINT('Ctrl Pts',(190.499075807096,51.5254438225133,102.292273143214));
#96288=CARTESIAN_POINT('Ctrl Pts',(190.499015087286,51.5165815564384,102.296626970431));
#96289=CARTESIAN_POINT('Ctrl Pts',(190.498950971254,51.5076773758461,102.301210936651));
#96290=CARTESIAN_POINT('Ctrl Pts',(190.498887080431,51.4988044714745,102.305778801541));
#96291=CARTESIAN_POINT('Ctrl Pts',(190.498819817172,51.489890005652,102.310575180582));
#96292=CARTESIAN_POINT('Ctrl Pts',(190.498749764597,51.4809597062609,102.31555539242));
#96293=CARTESIAN_POINT('Ctrl Pts',(190.498728849729,51.4782934797706,102.317042282405));
#96294=CARTESIAN_POINT('Ctrl Pts',(190.498707687303,51.4756254949432,102.31854548342));
#96295=CARTESIAN_POINT('Ctrl Pts',(190.498686295542,51.472955560573,102.320063617662));
#96296=CARTESIAN_POINT('Ctrl Pts',(190.49858999832,51.4609365752182,102.326897655768));
#96297=CARTESIAN_POINT('Ctrl Pts',(190.498488595803,51.4488755337678,102.334067398576));
#96298=CARTESIAN_POINT('Ctrl Pts',(190.498382995867,51.4369286075406,102.341503710545));
#96299=CARTESIAN_POINT('Ctrl Pts',(190.49827545108,51.4247616529285,102.349076978219));
#96300=CARTESIAN_POINT('Ctrl Pts',(190.498163552905,51.4127129205985,102.356926676939));
#96301=CARTESIAN_POINT('Ctrl Pts',(190.498048409372,51.4008932928763,102.364971649728));
#96302=CARTESIAN_POINT('Ctrl Pts',(190.497920233672,51.387735896961,102.373927168007));
#96303=CARTESIAN_POINT('Ctrl Pts',(190.49778803536,51.3748625721735,102.383124630778));
#96304=CARTESIAN_POINT('Ctrl Pts',(190.49765353826,51.3623579799668,102.392442509208));
#96305=CARTESIAN_POINT('Ctrl Pts',(190.497499626757,51.348048373481,102.403105405798));
#96306=CARTESIAN_POINT('Ctrl Pts',(190.497340595809,51.3340223984724,102.414076149627));
#96307=CARTESIAN_POINT('Ctrl Pts',(190.497177021594,51.3201942330095,102.425308352082));
#96308=CARTESIAN_POINT('Ctrl Pts',(190.497077659119,51.3117943716334,102.432131306568));
#96309=CARTESIAN_POINT('Ctrl Pts',(190.496976622798,51.3034664870513,102.439050563475));
#96310=CARTESIAN_POINT('Ctrl Pts',(190.496874065214,51.2951820979778,102.4460541533));
#96311=CARTESIAN_POINT('Ctrl Pts',(190.496632990611,51.2757085913373,102.462516978955));
#96312=CARTESIAN_POINT('Ctrl Pts',(190.49638320033,51.2565388519805,102.479469354575));
#96313=CARTESIAN_POINT('Ctrl Pts',(190.496125351658,51.2377329006417,102.496851940838));
#96314=CARTESIAN_POINT('Ctrl Pts',(190.495861249209,51.2184708358817,102.51465611869));
#96315=CARTESIAN_POINT('Ctrl Pts',(190.495588692412,51.1995904330682,102.532911629592));
#96316=CARTESIAN_POINT('Ctrl Pts',(190.495308471908,51.1811007324381,102.551551257997));
#96317=CARTESIAN_POINT('Ctrl Pts',(190.49502123726,51.1621482198251,102.570657451197));
#96318=CARTESIAN_POINT('Ctrl Pts',(190.494725950315,51.143606007776,102.590167219544));
#96319=CARTESIAN_POINT('Ctrl Pts',(190.494423553778,51.1254276671506,102.610004672516));
#96320=CARTESIAN_POINT('Ctrl Pts',(190.49410167335,51.1060780671041,102.631120284159));
#96321=CARTESIAN_POINT('Ctrl Pts',(190.493771737142,51.0871405553085,102.652607156205));
#96322=CARTESIAN_POINT('Ctrl Pts',(190.493434990178,51.0684986842281,102.674369990984));
#96323=CARTESIAN_POINT('Ctrl Pts',(190.49327146515,51.0594461527773,102.684938068912));
#96324=CARTESIAN_POINT('Ctrl Pts',(190.493106335701,51.0504624770422,102.69557116779));
#96325=CARTESIAN_POINT('Ctrl Pts',(190.492939753098,51.0415300296156,102.706258106843));
#96326=CARTESIAN_POINT('Ctrl Pts',(190.492873196198,51.037961133462,102.710527997709));
#96327=CARTESIAN_POINT('Ctrl Pts',(190.492806404688,51.0344025574796,102.7148066594));
#96328=CARTESIAN_POINT('Ctrl Pts',(190.492739387011,51.0308546706283,102.719093465428));
#96329=CARTESIAN_POINT('Ctrl Pts',(190.492217277783,51.00321443393,102.752490340321));
#96330=CARTESIAN_POINT('Ctrl Pts',(190.491680105235,50.9761560277177,102.78649716168));
#96331=CARTESIAN_POINT('Ctrl Pts',(190.491128747327,50.9496781884247,102.821001634167));
#96332=CARTESIAN_POINT('Ctrl Pts',(190.490561797783,50.9224515926376,102.856481845178));
#96333=CARTESIAN_POINT('Ctrl Pts',(190.489979853435,50.8958386079739,102.892488229329));
#96334=CARTESIAN_POINT('Ctrl Pts',(190.489383684826,50.8697813267168,102.928894775142));
#96335=CARTESIAN_POINT('Ctrl Pts',(190.488750358062,50.8420999403357,102.96757047778));
#96336=CARTESIAN_POINT('Ctrl Pts',(190.488100985496,50.8150454753715,103.006697754866));
#96337=CARTESIAN_POINT('Ctrl Pts',(190.48743619729,50.7884887641956,103.046121498537));
#96338=CARTESIAN_POINT('Ctrl Pts',(190.487145966101,50.7768947169831,103.063332995186));
#96339=CARTESIAN_POINT('Ctrl Pts',(190.486852792435,50.765394825828,103.080600950831));
#96340=CARTESIAN_POINT('Ctrl Pts',(190.486556707587,50.7539753280591,103.097912264592));
#96341=CARTESIAN_POINT('Ctrl Pts',(190.485781475642,50.724075927493,103.143238067439));
#96342=CARTESIAN_POINT('Ctrl Pts',(190.484990248106,50.6948833065813,103.188902737648));
#96343=CARTESIAN_POINT('Ctrl Pts',(190.484183841959,50.6660948762953,103.23483075695));
#96344=CARTESIAN_POINT('Ctrl Pts',(190.483057216169,50.6258747116616,103.298996551309));
#96345=CARTESIAN_POINT('Ctrl Pts',(190.481900571853,50.5865712041433,103.363708602892));
#96346=CARTESIAN_POINT('Ctrl Pts',(190.480713977185,50.5480908227822,103.428837031643));
#96347=CARTESIAN_POINT('Ctrl Pts',(190.48030288073,50.5347592709413,103.451400815927));
#96348=CARTESIAN_POINT('Ctrl Pts',(190.479888180932,50.5215260489788,103.474014558782));
#96349=CARTESIAN_POINT('Ctrl Pts',(190.479469852368,50.5083858374461,103.496672801637));
#96350=CARTESIAN_POINT('Ctrl Pts',(190.476436358211,50.4131000779096,103.66097821444));
#96351=CARTESIAN_POINT('Ctrl Pts',(190.473188613689,50.3220653991955,103.827547153392));
#96352=CARTESIAN_POINT('Ctrl Pts',(190.46973453625,50.2336378965589,103.995526950525));
#96353=CARTESIAN_POINT('Ctrl Pts',(190.467665095073,50.1806583330469,104.096168674713));
#96354=CARTESIAN_POINT('Ctrl Pts',(190.465522226543,50.128613102748,104.197316875812));
#96355=CARTESIAN_POINT('Ctrl Pts',(190.463314699951,50.0771562760488,104.298790001184));
#96356=CARTESIAN_POINT('Ctrl Pts',(190.463157784645,50.0734986241936,104.306002909346));
#96357=CARTESIAN_POINT('Ctrl Pts',(190.463000546636,50.0698445782581,104.313217483716));
#96358=CARTESIAN_POINT('Ctrl Pts',(190.462842989874,50.0661942109542,104.3204336661));
#96359=CARTESIAN_POINT('Ctrl Pts',(190.460234376599,50.0057563310984,104.439909523633));
#96360=CARTESIAN_POINT('Ctrl Pts',(190.4575319713,49.946177244841,104.559852577398));
#96361=CARTESIAN_POINT('Ctrl Pts',(190.454729245207,49.8872683438416,104.680145857249));
#96362=CARTESIAN_POINT('Ctrl Pts',(190.451857501286,49.82690879648,104.803401389083));
#96363=CARTESIAN_POINT('Ctrl Pts',(190.448880494172,49.7672527304977,104.927024628702));
#96364=CARTESIAN_POINT('Ctrl Pts',(190.445787762928,49.7080428432841,105.050886546628));
#96365=CARTESIAN_POINT('Ctrl Pts',(190.444871046973,49.6904924504486,105.08760043715));
#96366=CARTESIAN_POINT('Ctrl Pts',(190.443944137777,49.6729809089871,105.124335275583));
#96367=CARTESIAN_POINT('Ctrl Pts',(190.443006694391,49.655500653764,105.161087645489));
#96368=CARTESIAN_POINT('Ctrl Pts',(190.437604122775,49.5547603507539,105.372894900784));
#96369=CARTESIAN_POINT('Ctrl Pts',(190.43186467886,49.4553128650949,105.585253901174));
#96370=CARTESIAN_POINT('Ctrl Pts',(190.425767977364,49.3563958270275,105.797898094705));
#96371=CARTESIAN_POINT('Ctrl Pts',(190.419697186698,49.2578991839181,106.009638555689));
#96372=CARTESIAN_POINT('Ctrl Pts',(190.41327196394,49.1599272263073,106.221661693927));
#96373=CARTESIAN_POINT('Ctrl Pts',(190.406482906553,49.0617771372373,106.433708381924));
#96374=CARTESIAN_POINT('Ctrl Pts',(190.401950664083,48.996254049606,106.575266620446));
#96375=CARTESIAN_POINT('Ctrl Pts',(190.3972566273,48.9307847293818,106.716843520304));
#96376=CARTESIAN_POINT('Ctrl Pts',(190.392398235184,48.865383382616,106.858372934206));
#96377=CARTESIAN_POINT('Ctrl Pts',(190.38241104125,48.7309405632426,107.149309044396));
#96378=CARTESIAN_POINT('Ctrl Pts',(190.371691438842,48.5962741276876,107.440080064837));
#96379=CARTESIAN_POINT('Ctrl Pts',(190.360163745888,48.4608401849474,107.730416452946));
#96380=CARTESIAN_POINT('Ctrl Pts',(190.349247469066,48.3325895092942,108.005353718954));
#96381=CARTESIAN_POINT('Ctrl Pts',(190.337606452941,48.203650213339,108.279901220201));
#96382=CARTESIAN_POINT('Ctrl Pts',(190.325186866745,48.0736022962362,108.553832171948));
#96383=CARTESIAN_POINT('Ctrl Pts',(190.324928765199,48.0708996644553,108.559524954366));
#96384=CARTESIAN_POINT('Ctrl Pts',(190.324670326008,48.0681965365245,108.565217466365));
#96385=CARTESIAN_POINT('Ctrl Pts',(190.324411548623,48.0654929077705,108.570909706858));
#96386=CARTESIAN_POINT('Ctrl Pts',(190.30809950033,47.8950695038768,108.929720434545));
#96387=CARTESIAN_POINT('Ctrl Pts',(190.290445173734,47.7227602459063,109.287455099581));
#96388=CARTESIAN_POINT('Ctrl Pts',(190.271252865212,47.5479923029685,109.643858481022));
#96389=CARTESIAN_POINT('Ctrl Pts',(190.252060556691,47.3732243600308,110.000261862464));
#96390=CARTESIAN_POINT('Ctrl Pts',(190.231330066105,47.19599710458,110.355333952089));
#96391=CARTESIAN_POINT('Ctrl Pts',(190.208885317062,47.0157890831752,110.708819911125));
#96392=CARTESIAN_POINT('Ctrl Pts',(190.187535799278,46.8443746311556,111.045056897095));
#96393=CARTESIAN_POINT('Ctrl Pts',(190.164687494095,46.6702470477431,111.379862490087));
#96394=CARTESIAN_POINT('Ctrl Pts',(190.140086540729,46.4931565230915,111.713020121159));
#96395=CARTESIAN_POINT('Ctrl Pts',(190.135640195587,46.4611494060373,111.773234609293));
#96396=CARTESIAN_POINT('Ctrl Pts',(190.131136667723,46.4290456179944,111.833395265089));
#96397=CARTESIAN_POINT('Ctrl Pts',(190.126574553226,46.3968438430142,111.893500810988));
#96398=CARTESIAN_POINT('Ctrl Pts',(190.103520003164,46.234112847576,112.197242928358));
#96399=CARTESIAN_POINT('Ctrl Pts',(190.078949349961,46.0687489493423,112.499768106126));
#96400=CARTESIAN_POINT('Ctrl Pts',(190.05269520814,45.9006448211917,112.800818213231));
#96401=CARTESIAN_POINT('Ctrl Pts',(190.026979163907,45.7359861084927,113.09569808108));
#96402=CARTESIAN_POINT('Ctrl Pts',(189.999647793594,45.5686981823395,113.389162719898));
#96403=CARTESIAN_POINT('Ctrl Pts',(189.970568077575,45.3987230083238,113.6809699866));
#96404=CARTESIAN_POINT('Ctrl Pts',(189.942216363998,45.2330031145719,113.965471941159));
#96405=CARTESIAN_POINT('Ctrl Pts',(189.912202667965,45.0647287721212,114.248398465848));
#96406=CARTESIAN_POINT('Ctrl Pts',(189.880428588463,44.8938888954231,114.52952562181));
#96407=CARTESIAN_POINT('Ctrl Pts',(189.86320062523,44.8012592060418,114.681953272992));
#96408=CARTESIAN_POINT('Ctrl Pts',(189.845455581042,44.7078760453384,114.833851949159));
#96409=CARTESIAN_POINT('Ctrl Pts',(189.827181068214,44.6137431943845,114.98518601914));
#96410=CARTESIAN_POINT('Ctrl Pts',(189.821506870443,44.5845151422847,115.032174929357));
#96411=CARTESIAN_POINT('Ctrl Pts',(189.815780524983,44.5552150513257,115.07910917213));
#96412=CARTESIAN_POINT('Ctrl Pts',(189.810001379507,44.5258437663493,115.125987692428));
#96413=CARTESIAN_POINT('Ctrl Pts',(189.765174624184,44.2980212602981,115.489607533465));
#96414=CARTESIAN_POINT('Ctrl Pts',(189.717207375984,44.0661209111254,115.849506313826));
#96415=CARTESIAN_POINT('Ctrl Pts',(189.665770468423,43.830187225881,116.205776137928));
#96416=CARTESIAN_POINT('Ctrl Pts',(189.621237067927,43.6259189330552,116.514229882798));
#96417=CARTESIAN_POINT('Ctrl Pts',(189.574103889631,43.4186275748335,116.819963409595));
#96418=CARTESIAN_POINT('Ctrl Pts',(189.524188097192,43.2083484666004,117.123036448682));
#96419=CARTESIAN_POINT('Ctrl Pts',(189.471931048151,42.9882064006407,117.440324863695));
#96420=CARTESIAN_POINT('Ctrl Pts',(189.416593974544,42.7647307895591,117.754697553232));
#96421=CARTESIAN_POINT('Ctrl Pts',(189.358051649801,42.5384379229682,118.066222446577));
#96422=CARTESIAN_POINT('Ctrl Pts',(189.34997393449,42.5072138579641,118.109206892648));
#96423=CARTESIAN_POINT('Ctrl Pts',(189.341835231097,42.4759360834058,118.152137120363));
#96424=CARTESIAN_POINT('Ctrl Pts',(189.333635244335,42.4446058864512,118.195013308131));
#96425=CARTESIAN_POINT('Ctrl Pts',(189.281169294919,42.2441459861673,118.469347884994));
#96426=CARTESIAN_POINT('Ctrl Pts',(189.226201434868,42.0415675978545,118.74145480887));
#96427=CARTESIAN_POINT('Ctrl Pts',(189.168605458159,41.837000994173,119.011626542698));
#96428=CARTESIAN_POINT('Ctrl Pts',(189.150898374159,41.7741098298585,119.094687094124));
#96429=CARTESIAN_POINT('Ctrl Pts',(189.132942815417,41.7110303772408,119.177564735845));
#96430=CARTESIAN_POINT('Ctrl Pts',(189.114734900347,41.6477654678563,119.260267962345));
#96431=CARTESIAN_POINT('Ctrl Pts',(189.062359779652,41.4657837718707,119.498164034092));
#96432=CARTESIAN_POINT('Ctrl Pts',(189.007870691134,41.2822558358634,119.734617066258));
#96433=CARTESIAN_POINT('Ctrl Pts',(188.951308014775,41.0975794254857,119.969828354958));
#96434=CARTESIAN_POINT('Ctrl Pts',(188.891670312216,40.9028630941394,120.217826889982));
#96435=CARTESIAN_POINT('Ctrl Pts',(188.829727582339,40.7068697456579,120.464445000665));
#96436=CARTESIAN_POINT('Ctrl Pts',(188.765505290305,40.5100109306358,120.709918499324));
#96437=CARTESIAN_POINT('Ctrl Pts',(188.731311904526,40.4051988911872,120.840614084493));
#96438=CARTESIAN_POINT('Ctrl Pts',(188.696471946879,40.3001406356658,120.97098519985));
#96439=CARTESIAN_POINT('Ctrl Pts',(188.660986721352,40.194892939968,121.101067416233));
#96440=CARTESIAN_POINT('Ctrl Pts',(188.634061070125,40.1150325838717,121.199771830171));
#96441=CARTESIAN_POINT('Ctrl Pts',(188.606759755875,40.0350508878436,121.298330966865));
#96442=CARTESIAN_POINT('Ctrl Pts',(188.579082594393,39.9549720968558,121.396759465166));
#96443=CARTESIAN_POINT('Ctrl Pts',(188.505122801803,39.7409830005985,121.65978323385));
#96444=CARTESIAN_POINT('Ctrl Pts',(188.428490328119,39.5263977759299,121.921874171461));
#96445=CARTESIAN_POINT('Ctrl Pts',(188.349443899174,39.3119399066477,122.183309854839));
#96446=CARTESIAN_POINT('Ctrl Pts',(188.25931230754,39.0674073027749,122.48140825811));
#96447=CARTESIAN_POINT('Ctrl Pts',(188.166042607857,38.8230391186135,122.778654761601));
#96448=CARTESIAN_POINT('Ctrl Pts',(188.06996723637,38.5798577704378,123.075460334885));
#96449=CARTESIAN_POINT('Ctrl Pts',(188.020644387728,38.4550141539823,123.227833374309));
#96450=CARTESIAN_POINT('Ctrl Pts',(187.97058127727,38.3304826937849,123.380090193964));
#96451=CARTESIAN_POINT('Ctrl Pts',(187.919818326087,38.2063995497728,123.532286325396));
#96452=CARTESIAN_POINT('Ctrl Pts',(187.876714762721,38.1010387396561,123.661518283791));
#96453=CARTESIAN_POINT('Ctrl Pts',(187.833119954047,37.9960248692047,123.790706450871));
#96454=CARTESIAN_POINT('Ctrl Pts',(187.789067088822,37.8914036208365,123.91988464976));
#96455=CARTESIAN_POINT('Ctrl Pts',(187.688880417279,37.6534700700169,124.213666534698));
#96456=CARTESIAN_POINT('Ctrl Pts',(187.586266219707,37.4174238641642,124.507604623262));
#96457=CARTESIAN_POINT('Ctrl Pts',(187.481605512553,37.1838645680724,124.8020774362));
#96458=CARTESIAN_POINT('Ctrl Pts',(187.379427626148,36.9558458982757,125.089564597795));
#96459=CARTESIAN_POINT('Ctrl Pts',(187.275298297069,36.7301962684332,125.377561423478));
#96460=CARTESIAN_POINT('Ctrl Pts',(187.169565526471,36.5075211301387,125.666419468782));
#96461=CARTESIAN_POINT('Ctrl Pts',(187.060011656538,36.2767986871335,125.965716617105));
#96462=CARTESIAN_POINT('Ctrl Pts',(186.948763090548,36.0492413463077,126.265938222591));
#96463=CARTESIAN_POINT('Ctrl Pts',(186.835993331848,35.8248118979545,126.567473823342));
#96464=CARTESIAN_POINT('Ctrl Pts',(186.81435442702,35.7817470946811,126.62533419515));
#96465=CARTESIAN_POINT('Ctrl Pts',(186.792659524023,35.7387976140255,126.683242945147));
#96466=CARTESIAN_POINT('Ctrl Pts',(186.770909873261,35.6959634156462,126.741202820671));
#96467=CARTESIAN_POINT('Ctrl Pts',(186.639338192594,35.4368435091902,127.091823541781));
#96468=CARTESIAN_POINT('Ctrl Pts',(186.505773556998,35.1819666145873,127.444279414045));
#96469=CARTESIAN_POINT('Ctrl Pts',(186.370723311232,34.9317582538241,127.798621865455));
#96470=CARTESIAN_POINT('Ctrl Pts',(186.20804502502,34.6303632649153,128.225454281794));
#96471=CARTESIAN_POINT('Ctrl Pts',(186.043351381547,34.335748183931,128.655024244082));
#96472=CARTESIAN_POINT('Ctrl Pts',(185.876684597081,34.0472913013621,129.087419480968));
#96473=CARTESIAN_POINT('Ctrl Pts',(185.806771876844,33.9262905548952,129.26879891614));
#96474=CARTESIAN_POINT('Ctrl Pts',(185.736512055574,33.8063728032299,129.450675459093));
#96475=CARTESIAN_POINT('Ctrl Pts',(185.665908670656,33.6874894197892,129.633055460434));
#96476=CARTESIAN_POINT('Ctrl Pts',(185.527287154577,33.4540757545885,129.991137333107));
#96477=CARTESIAN_POINT('Ctrl Pts',(185.387363065923,33.2246908054913,130.351102371684));
#96478=CARTESIAN_POINT('Ctrl Pts',(185.246262498078,32.999087553421,130.712756874191));
#96479=CARTESIAN_POINT('Ctrl Pts',(185.10220568057,32.7687576050079,131.081988532605));
#96480=CARTESIAN_POINT('Ctrl Pts',(184.956922586553,32.5423693847545,131.452981180414));
#96481=CARTESIAN_POINT('Ctrl Pts',(184.810554291019,32.319606258196,131.825528446831));
#96482=CARTESIAN_POINT('Ctrl Pts',(184.780554568769,32.2739486115059,131.901885929007));
#96483=CARTESIAN_POINT('Ctrl Pts',(184.75050928061,32.2284430769014,131.978308718369));
#96484=CARTESIAN_POINT('Ctrl Pts',(184.720419674804,32.1830866635913,132.054795037419));
#96485=CARTESIAN_POINT('Ctrl Pts',(184.648336307881,32.0744297737673,132.238027461138));
#96486=CARTESIAN_POINT('Ctrl Pts',(184.575973994326,31.9665951990179,132.42162468394));
#96487=CARTESIAN_POINT('Ctrl Pts',(184.503318676827,31.8595431559822,132.605562041294));
#96488=CARTESIAN_POINT('Ctrl Pts',(184.348768662941,31.6318255530998,132.996827568877));
#96489=CARTESIAN_POINT('Ctrl Pts',(184.192900936543,31.4076637868292,133.38959457567));
#96490=CARTESIAN_POINT('Ctrl Pts',(184.035599174924,31.186668157996,133.783560786267));
#96491=CARTESIAN_POINT('Ctrl Pts',(183.868593799099,30.9520397745063,134.201829942223));
#96492=CARTESIAN_POINT('Ctrl Pts',(183.699971816693,30.7209801122015,134.621450788687));
#96493=CARTESIAN_POINT('Ctrl Pts',(183.52958893264,30.4929612354519,135.04206209289));
#96494=CARTESIAN_POINT('Ctrl Pts',(183.36063949118,30.2668606967534,135.459134766077));
#96495=CARTESIAN_POINT('Ctrl Pts',(183.189958389329,30.0437491561647,135.877181275877));
#96496=CARTESIAN_POINT('Ctrl Pts',(183.017403636412,29.823061307358,136.295850324503));
#96497=CARTESIAN_POINT('Ctrl Pts',(182.810366744021,29.5582727365807,136.798183278554));
#96498=CARTESIAN_POINT('Ctrl Pts',(182.600620696084,29.2970147069744,137.301414781572));
#96499=CARTESIAN_POINT('Ctrl Pts',(182.387736218738,29.0386703876795,137.804925385732));
#96500=CARTESIAN_POINT('Ctrl Pts',(182.262081339166,28.8861828755141,138.102122086581));
#96501=CARTESIAN_POINT('Ctrl Pts',(182.135333110065,28.7347093094155,138.399416072433));
#96502=CARTESIAN_POINT('Ctrl Pts',(182.007405205727,28.5841147979743,138.696680511829));
#96503=CARTESIAN_POINT('Ctrl Pts',(181.768065544775,28.3023682978958,139.252831028844));
#96504=CARTESIAN_POINT('Ctrl Pts',(181.524579784592,28.0236833319436,139.80891000626));
#96505=CARTESIAN_POINT('Ctrl Pts',(181.276383640261,27.7471156056873,140.36413417791));
#96506=CARTESIAN_POINT('Ctrl Pts',(181.253733983975,27.7218768415782,140.414802316545));
#96507=CARTESIAN_POINT('Ctrl Pts',(181.231045128986,27.6966556886218,140.465463341053));
#96508=CARTESIAN_POINT('Ctrl Pts',(181.208316664928,27.6714514183718,140.51611665903));
#96509=CARTESIAN_POINT('Ctrl Pts',(180.980534297709,27.4188567719832,141.023759086915));
#96510=CARTESIAN_POINT('Ctrl Pts',(180.748822648448,27.1680200449666,141.530632755925));
#96511=CARTESIAN_POINT('Ctrl Pts',(180.512479092602,26.9183528177257,142.036107824096));
#96512=CARTESIAN_POINT('Ctrl Pts',(180.299672774679,26.6935497206205,142.491243093911));
#96513=CARTESIAN_POINT('Ctrl Pts',(180.083110983336,26.4696940369098,142.945244465906));
#96514=CARTESIAN_POINT('Ctrl Pts',(179.862320517908,26.2463607446773,143.397657233819));
#96515=CARTESIAN_POINT('Ctrl Pts',(179.648388584287,26.0299649734357,143.836016462994));
#96516=CARTESIAN_POINT('Ctrl Pts',(179.430486159255,25.8140590945568,144.27288421347));
#96517=CARTESIAN_POINT('Ctrl Pts',(179.208227260175,25.5982699452165,144.707852190921));
#96518=CARTESIAN_POINT('Ctrl Pts',(179.195518563554,25.585931186928,144.732723528305));
#96519=CARTESIAN_POINT('Ctrl Pts',(179.182795480721,25.5735928331242,144.757588637647));
#96520=CARTESIAN_POINT('Ctrl Pts',(179.170057878368,25.5612547983027,144.78244743594));
#96521=CARTESIAN_POINT('Ctrl Pts',(178.979847025161,25.3770106944807,145.153664333906));
#96522=CARTESIAN_POINT('Ctrl Pts',(178.786394805049,25.1928363963962,145.523476609339));
#96523=CARTESIAN_POINT('Ctrl Pts',(178.589310654333,25.0084853544995,145.891550971731));
#96524=CARTESIAN_POINT('Ctrl Pts',(178.428416829498,24.8579864730049,146.192036281046));
#96525=CARTESIAN_POINT('Ctrl Pts',(178.265103079925,24.7073699745978,146.49136341204));
#96526=CARTESIAN_POINT('Ctrl Pts',(178.099180810728,24.5565114251989,146.789353762951));
#96527=CARTESIAN_POINT('Ctrl Pts',(177.920514420468,24.3940657656058,147.110232091021));
#96528=CARTESIAN_POINT('Ctrl Pts',(177.73884300383,24.2313506353695,147.429562397532));
#96529=CARTESIAN_POINT('Ctrl Pts',(177.553755639537,24.0681325678661,147.747103367846));
#96530=CARTESIAN_POINT('Ctrl Pts',(177.382332626396,23.9169643180119,148.041201401682));
#96531=CARTESIAN_POINT('Ctrl Pts',(177.207966406531,23.7653534854513,148.333785835995));
#96532=CARTESIAN_POINT('Ctrl Pts',(177.030419553461,23.6131761028683,148.624584498751));
#96533=CARTESIAN_POINT('Ctrl Pts',(176.982805614263,23.572365665981,148.702569940949));
#96534=CARTESIAN_POINT('Ctrl Pts',(176.934963189111,23.5315145984672,148.780426981826));
#96535=CARTESIAN_POINT('Ctrl Pts',(176.886888290586,23.490620772596,148.858150437944));
#96536=CARTESIAN_POINT('Ctrl Pts',(176.728507612646,23.3558978285284,149.114207009035));
#96537=CARTESIAN_POINT('Ctrl Pts',(176.56763806299,23.2207301604003,149.368817187247));
#96538=CARTESIAN_POINT('Ctrl Pts',(176.403920824963,23.084931065456,149.621773376208));
#96539=CARTESIAN_POINT('Ctrl Pts',(176.245282158161,22.9533445102802,149.866882767617));
#96540=CARTESIAN_POINT('Ctrl Pts',(176.083969629685,22.8211650153288,150.110439183361));
#96541=CARTESIAN_POINT('Ctrl Pts',(175.919700886915,22.6882438794319,150.35225852202));
#96542=CARTESIAN_POINT('Ctrl Pts',(175.861583564823,22.6412171576257,150.43781279215));
#96543=CARTESIAN_POINT('Ctrl Pts',(175.803096631979,22.5940978076811,150.523149677045));
#96544=CARTESIAN_POINT('Ctrl Pts',(175.744229001408,22.5468799342391,150.608261176452));
#96545=CARTESIAN_POINT('Origin',(160.5,51.8013867006572,102.225104347672));
#96546=CARTESIAN_POINT('Origin',(160.5,51.8013867006572,102.225104347672));
#96547=CARTESIAN_POINT('',(190.5,51.8013867006572,102.225104347672));
#96548=CARTESIAN_POINT('',(190.499797482064,51.8013867006573,102.335336081499));
#96549=CARTESIAN_POINT('Ctrl Pts',(-190.499797482064,25.5156816663762,102.335336081498));
#96550=CARTESIAN_POINT('Ctrl Pts',(-190.499797482064,60.1768636667247,102.335336081498));
#96551=CARTESIAN_POINT('Ctrl Pts',(-190.141509581597,25.5156816663762,199.844139409912));
#96552=CARTESIAN_POINT('Ctrl Pts',(-190.141509581597,60.1768636667247,199.844139409912));
#96553=CARTESIAN_POINT('Ctrl Pts',(-180.969631132311,25.5156816663762,196.));
#96554=CARTESIAN_POINT('Ctrl Pts',(-180.969631132311,60.1768636667247,196.));
#96555=CARTESIAN_POINT('Ctrl Pts',(1.58515917575596E-14,25.5156816663763,
196.));
#96556=CARTESIAN_POINT('Ctrl Pts',(1.58515917575596E-14,60.1768636667247,
196.));
#96557=CARTESIAN_POINT('',(3.34339434094657E-14,-112.4,196.));
#96558=CARTESIAN_POINT('Ctrl Pts',(129.971165261432,38.9257468402258,193.360148302349));
#96559=CARTESIAN_POINT('Ctrl Pts',(129.971165261432,57.4948506319549,193.360148302349));
#96560=CARTESIAN_POINT('Ctrl Pts',(186.116291121746,38.9257468402258,187.246632700069));
#96561=CARTESIAN_POINT('Ctrl Pts',(186.116291121746,57.4948506319549,187.246632700069));
#96562=CARTESIAN_POINT('Ctrl Pts',(190.261265602416,38.9257468402258,167.252287253607));
#96563=CARTESIAN_POINT('Ctrl Pts',(190.261265602416,57.4948506319549,167.252287253607));
#96564=CARTESIAN_POINT('Ctrl Pts',(190.499797482064,38.9257468402258,102.3353360815));
#96565=CARTESIAN_POINT('Ctrl Pts',(190.499797482064,57.4948506319549,102.3353360815));
#96566=CARTESIAN_POINT('Origin',(-122.710817715584,2.64173312008429,40.));
#96567=CARTESIAN_POINT('Origin',(-190.5,59.,211.4));
#96568=CARTESIAN_POINT('',(-190.5,51.8013867006572,211.4));
#96569=CARTESIAN_POINT('Origin',(190.5,59.,211.4));
#96570=CARTESIAN_POINT('',(190.5,51.8013867006572,211.4));
#96571=CARTESIAN_POINT('Ctrl Pts',(148.824154305368,8.98894876016889,150.608250755187));
#96572=CARTESIAN_POINT('Ctrl Pts',(148.824154305368,8.98894876016889,19.0783498489626));
#96573=CARTESIAN_POINT('Ctrl Pts',(173.689807552334,17.1099506086912,150.608250755187));
#96574=CARTESIAN_POINT('Ctrl Pts',(173.689807552334,17.1099506086912,19.0783498489626));
#96575=CARTESIAN_POINT('Ctrl Pts',(190.5,30.3189740729563,150.608250755187));
#96576=CARTESIAN_POINT('Ctrl Pts',(190.5,30.3189740729563,19.0783498489626));
#96577=CARTESIAN_POINT('Ctrl Pts',(190.5,51.8013867006572,150.608250755187));
#96578=CARTESIAN_POINT('Ctrl Pts',(190.5,51.8013867006572,19.0783498489626));
#96579=CARTESIAN_POINT('Ctrl Pts',(-190.5,51.8013867006572,150.608250755187));
#96580=CARTESIAN_POINT('Ctrl Pts',(-190.5,51.8013867006572,19.0783498489627));
#96581=CARTESIAN_POINT('Ctrl Pts',(-190.5,-4.93900225262807,150.608250755187));
#96582=CARTESIAN_POINT('Ctrl Pts',(-190.5,-4.93900225262807,19.0783498489627));
#96583=CARTESIAN_POINT('Ctrl Pts',(-73.2288472415572,-3.96262874552467,
150.608250755187));
#96584=CARTESIAN_POINT('Ctrl Pts',(-73.2288472415572,-3.96262874552467,
19.0783498489627));
#96585=CARTESIAN_POINT('Ctrl Pts',(7.71069817591099E-15,-3.96262874552467,
150.608250755187));
#96586=CARTESIAN_POINT('Ctrl Pts',(7.71069817591099E-15,-3.96262874552467,
19.0783498489627));
#96587=CARTESIAN_POINT('',(7.71069817591099E-15,-3.96262874552467,211.4));
#96588=CARTESIAN_POINT('Ctrl Pts',(153.843438675571,24.8757620423259,184.508710490748));
#96589=CARTESIAN_POINT('Ctrl Pts',(154.097189311659,24.8757620423259,185.073807734126));
#96590=CARTESIAN_POINT('Ctrl Pts',(154.210203413018,25.4303873898659,185.325487722502));
#96591=CARTESIAN_POINT('Ctrl Pts',(155.446182926033,24.8757620423259,183.789015999753));
#96592=CARTESIAN_POINT('Ctrl Pts',(155.704024681242,24.8757620423411,184.341199300067));
#96593=CARTESIAN_POINT('Ctrl Pts',(155.832745509897,25.4172512189876,184.589740299172));
#96594=CARTESIAN_POINT('Ctrl Pts',(157.036128954789,24.8757620423259,182.994575738328));
#96595=CARTESIAN_POINT('Ctrl Pts',(157.306394375555,24.8757620423136,183.529968721434));
#96596=CARTESIAN_POINT('Ctrl Pts',(157.443723445175,25.4039841842481,183.777098085943));
#96597=CARTESIAN_POINT('Ctrl Pts',(160.10416844211,24.8757620423259,181.266959679052));
#96598=CARTESIAN_POINT('Ctrl Pts',(160.398490808051,24.8757620423381,181.765887812577));
#96599=CARTESIAN_POINT('Ctrl Pts',(160.554889697529,25.3780508928129,182.00870277573));
#96600=CARTESIAN_POINT('Ctrl Pts',(161.585909292923,24.8757620423259,180.333133950633));
#96601=CARTESIAN_POINT('Ctrl Pts',(161.893267982881,24.8757620423381,180.813291368863));
#96602=CARTESIAN_POINT('Ctrl Pts',(162.058767051137,25.3653573201704,181.052285081176));
#96603=CARTESIAN_POINT('Ctrl Pts',(164.429011149336,24.8757620423259,178.304256437065));
#96604=CARTESIAN_POINT('Ctrl Pts',(164.76052871889,24.8757620423138,178.743922175154));
#96605=CARTESIAN_POINT('Ctrl Pts',(164.946574599667,25.3407885877743,178.972999501815));
#96606=CARTESIAN_POINT('Ctrl Pts',(165.790512137565,24.8757620423259,177.209392132235));
#96607=CARTESIAN_POINT('Ctrl Pts',(166.135033875418,24.8757620423076,177.627992122806));
#96608=CARTESIAN_POINT('Ctrl Pts',(166.330643962048,25.3289106297604,177.850325403001));
#96609=CARTESIAN_POINT('Ctrl Pts',(167.7262630848,24.8757620423259,175.424458331705));
#96610=CARTESIAN_POINT('Ctrl Pts',(168.091916053128,24.875762042335,175.805683882935));
#96611=CARTESIAN_POINT('Ctrl Pts',(168.299891924294,25.3119382317935,176.018973888766));
#96612=CARTESIAN_POINT('Ctrl Pts',(168.35370579661,24.8757620423259,174.805630477488));
#96613=CARTESIAN_POINT('Ctrl Pts',(168.725280353603,24.8757620423259,175.175178634881));
#96614=CARTESIAN_POINT('Ctrl Pts',(168.938439625813,25.3064219914066,175.38388734878));
#96615=CARTESIAN_POINT('Ctrl Pts',(169.265322202836,24.8757620423259,173.837815186678));
#96616=CARTESIAN_POINT('Ctrl Pts',(169.646212598391,24.8757620423259,174.188387298614));
#96617=CARTESIAN_POINT('Ctrl Pts',(169.866526829743,25.2984005760092,174.390370544029));
#96618=CARTESIAN_POINT('Ctrl Pts',(169.564467812621,24.8757620423259,173.508308943463));
#96619=CARTESIAN_POINT('Ctrl Pts',(169.948201978296,24.875762042322,173.852727851945));
#96620=CARTESIAN_POINT('Ctrl Pts',(170.171135592209,25.295767253308,174.052069713981));
#96621=CARTESIAN_POINT('Ctrl Pts',(170.147287755393,24.8757620423259,172.841326470637));
#96622=CARTESIAN_POINT('Ctrl Pts',(170.536563854742,24.8757620423297,173.173343282725));
#96623=CARTESIAN_POINT('Ctrl Pts',(170.764708940666,25.2906383278187,173.367194177139));
#96624=CARTESIAN_POINT('Ctrl Pts',(170.431610309457,24.8757620423259,172.503187193767));
#96625=CARTESIAN_POINT('Ctrl Pts',(170.823635650814,24.8757620423236,172.828932302436));
#96626=CARTESIAN_POINT('Ctrl Pts',(171.054333341806,25.2881370228471,173.019938913282));
#96627=CARTESIAN_POINT('Ctrl Pts',(171.817076225877,24.8757620423259,170.788785130436));
#96628=CARTESIAN_POINT('Ctrl Pts',(172.219289850269,24.875762042335,171.086871061764));
#96629=CARTESIAN_POINT('Ctrl Pts',(172.465898368354,25.2759637810014,171.259086668886));
#96630=CARTESIAN_POINT('Ctrl Pts',(172.810442504972,24.8757620423259,169.341840426858));
#96631=CARTESIAN_POINT('Ctrl Pts',(173.224067477814,24.8757620423259,169.612833465978));
#96632=CARTESIAN_POINT('Ctrl Pts',(173.478886091858,25.267312726279,169.772183826282));
#96633=CARTESIAN_POINT('Ctrl Pts',(174.107069219023,24.8757620423259,167.044573700205));
#96634=CARTESIAN_POINT('Ctrl Pts',(174.535707663812,24.8757620423259,167.271257953513));
#96635=CARTESIAN_POINT('Ctrl Pts',(174.802046949673,25.2562438193643,167.410304255125));
#96636=CARTESIAN_POINT('Ctrl Pts',(174.506855867878,24.8757620423259,166.257555096081));
#96637=CARTESIAN_POINT('Ctrl Pts',(174.939890357575,24.8757620423321,166.469932193093));
#96638=CARTESIAN_POINT('Ctrl Pts',(175.210198426796,25.2528791783321,166.600945447381));
#96639=CARTESIAN_POINT('Ctrl Pts',(175.054500634198,24.8757620423259,165.042901677538));
#96640=CARTESIAN_POINT('Ctrl Pts',(175.493435316943,24.8757620423228,165.23296575935));
#96641=CARTESIAN_POINT('Ctrl Pts',(175.769094570506,25.2480730731251,165.351948198845));
#96642=CARTESIAN_POINT('Ctrl Pts',(175.228346721299,24.8757620423259,164.632216279467));
#96643=CARTESIAN_POINT('Ctrl Pts',(175.669034332558,24.8757620423282,164.814988071584));
#96644=CARTESIAN_POINT('Ctrl Pts',(175.946466324372,25.2465059135025,164.929681619307));
#96645=CARTESIAN_POINT('Ctrl Pts',(175.555134756084,24.8757620423259,163.807963820627));
#96646=CARTESIAN_POINT('Ctrl Pts',(175.998882222778,24.8757620423236,163.976305634484));
#96647=CARTESIAN_POINT('Ctrl Pts',(176.279628859577,25.2433755556989,164.082445685088));
#96648=CARTESIAN_POINT('Ctrl Pts',(175.708568670929,24.8757620423259,163.393346553788));
#96649=CARTESIAN_POINT('Ctrl Pts',(176.153645063015,24.8757620423251,163.554541064828));
#96650=CARTESIAN_POINT('Ctrl Pts',(176.435919583728,25.2418067111356,163.656398290152));
#96651=CARTESIAN_POINT('Ctrl Pts',(176.427992501896,24.8757620423259,161.308318933633));
#96652=CARTESIAN_POINT('Ctrl Pts',(176.87730024609,24.8757620423289,161.437555001007));
#96653=CARTESIAN_POINT('Ctrl Pts',(177.16765157546,25.2336828542469,161.515194813592));
#96654=CARTESIAN_POINT('Ctrl Pts',(176.849355140085,24.8757620423259,159.601737069089));
#96655=CARTESIAN_POINT('Ctrl Pts',(177.298473156492,24.875762042329,159.707111376069));
#96656=CARTESIAN_POINT('Ctrl Pts',(177.591814447343,25.2258569061289,159.767692273689));
#96657=CARTESIAN_POINT('Ctrl Pts',(177.474201675422,24.8757620423259,156.129938446047));
#96658=CARTESIAN_POINT('Ctrl Pts',(177.915514314354,24.8757620423228,156.194887636441));
#96659=CARTESIAN_POINT('Ctrl Pts',(178.211970156958,25.2073379577766,156.230317176798));
#96660=CARTESIAN_POINT('Ctrl Pts',(177.679073669645,24.8757620423259,154.358973529501));
#96661=CARTESIAN_POINT('Ctrl Pts',(178.114003744645,24.8757620423629,154.40887674537));
#96662=CARTESIAN_POINT('Ctrl Pts',(178.409947754537,25.1969691506768,154.433928342043));
#96663=CARTESIAN_POINT('Ctrl Pts',(177.81394122412,24.8757620423259,152.596186324432));
#96664=CARTESIAN_POINT('Ctrl Pts',(178.241859855773,24.8757620423256,152.628925287436));
#96665=CARTESIAN_POINT('Ctrl Pts',(178.536663099516,25.1868384529694,152.651479916099));
#96666=CARTESIAN_POINT('Ctrl Pts',(177.813017113379,24.8757620423259,152.608250755187));
#96667=CARTESIAN_POINT('Ctrl Pts',(177.765987296558,24.8757620423259,153.221513948998));
#96668=CARTESIAN_POINT('Ctrl Pts',(177.710582914372,24.8757620423259,153.834376894056));
#96669=CARTESIAN_POINT('Ctrl Pts',(177.645263460167,24.8757620423259,154.44568556563));
#96670=CARTESIAN_POINT('Ctrl Pts',(177.586074917099,24.875762042326,154.999616551044));
#96671=CARTESIAN_POINT('Ctrl Pts',(177.51874600106,24.8757620423259,155.552273151529));
#96672=CARTESIAN_POINT('Ctrl Pts',(177.442095277715,24.8757620423273,156.102812608023));
#96673=CARTESIAN_POINT('Ctrl Pts',(177.36544455437,24.8757620423287,156.653352064516));
#96674=CARTESIAN_POINT('Ctrl Pts',(177.279473222263,24.8757620423312,157.201775687774));
#96675=CARTESIAN_POINT('Ctrl Pts',(177.182947814112,24.8757620423413,157.747235454427));
#96676=CARTESIAN_POINT('Ctrl Pts',(177.17583178297,24.875762042342,157.787447754595));
#96677=CARTESIAN_POINT('Ctrl Pts',(177.168658563601,24.8757620423432,157.827643161308));
#96678=CARTESIAN_POINT('Ctrl Pts',(177.161427682835,24.8757620423448,157.867821154608));
#96679=CARTESIAN_POINT('Ctrl Pts',(176.979848702746,24.8757620423849,158.87675482138));
#96680=CARTESIAN_POINT('Ctrl Pts',(176.761269560344,24.8757620439143,159.876604034587));
#96681=CARTESIAN_POINT('Ctrl Pts',(176.496786965883,24.8757620450215,160.864992501382));
#96682=CARTESIAN_POINT('Ctrl Pts',(176.328407801087,24.8757620457263,161.494236270229));
#96683=CARTESIAN_POINT('Ctrl Pts',(176.141424196877,24.8757620449383,162.118834667825));
#96684=CARTESIAN_POINT('Ctrl Pts',(175.933549890014,24.8757620433657,162.738171134661));
#96685=CARTESIAN_POINT('Ctrl Pts',(175.906871882401,24.8757620431639,162.817655046003));
#96686=CARTESIAN_POINT('Ctrl Pts',(175.879852392006,24.8757620430266,162.89704875974));
#96687=CARTESIAN_POINT('Ctrl Pts',(175.852486142522,24.8757620429244,162.976352314521));
#96688=CARTESIAN_POINT('Ctrl Pts',(175.708576843098,24.8757620423867,163.393381290935));
#96689=CARTESIAN_POINT('Ctrl Pts',(175.555168053394,24.8757620425669,163.807939748437));
#96690=CARTESIAN_POINT('Ctrl Pts',(175.391763439743,24.8757620426241,164.22009905024));
#96691=CARTESIAN_POINT('Ctrl Pts',(175.267447937342,24.8757620426675,164.533662966999));
#96692=CARTESIAN_POINT('Ctrl Pts',(175.137061255448,24.8757620426762,164.846446523615));
#96693=CARTESIAN_POINT('Ctrl Pts',(175.001324262928,24.8757620425231,165.156599195375));
#96694=CARTESIAN_POINT('Ctrl Pts',(174.958712271164,24.875762042475,165.253965601166));
#96695=CARTESIAN_POINT('Ctrl Pts',(174.915584685987,24.8757620424422,165.351048867319));
#96696=CARTESIAN_POINT('Ctrl Pts',(174.871964753249,24.875762042418,165.447791729611));
#96697=CARTESIAN_POINT('Ctrl Pts',(174.663058628572,24.875762042302,165.911116067434));
#96698=CARTESIAN_POINT('Ctrl Pts',(174.442901928491,24.875762042331,166.366783640181));
#96699=CARTESIAN_POINT('Ctrl Pts',(174.211821876959,24.8757620423295,166.815301616639));
#96700=CARTESIAN_POINT('Ctrl Pts',(174.097014960134,24.8757620423288,167.038137667074));
#96701=CARTESIAN_POINT('Ctrl Pts',(173.979511062044,24.875762042329,167.259208456611));
#96702=CARTESIAN_POINT('Ctrl Pts',(173.859346408156,24.8757620423283,167.478573498444));
#96703=CARTESIAN_POINT('Ctrl Pts',(173.798526854331,24.8757620423279,167.589601854432));
#96704=CARTESIAN_POINT('Ctrl Pts',(173.737029744405,24.8757620423276,167.700185927368));
#96705=CARTESIAN_POINT('Ctrl Pts',(173.674861839331,24.8757620423274,167.810330136494));
#96706=CARTESIAN_POINT('Ctrl Pts',(172.89367803685,24.8757620423246,169.194370213202));
#96707=CARTESIAN_POINT('Ctrl Pts',(172.007181861288,24.8757620420351,170.509352277933));
#96708=CARTESIAN_POINT('Ctrl Pts',(171.025691357068,24.8757620426587,171.762020930194));
#96709=CARTESIAN_POINT('Ctrl Pts',(170.92109883156,24.8757620427251,171.895511552264));
#96710=CARTESIAN_POINT('Ctrl Pts',(170.815442443059,24.8757620427619,172.028272940729));
#96711=CARTESIAN_POINT('Ctrl Pts',(170.708726570032,24.8757620427661,172.160325430636));
#96712=CARTESIAN_POINT('Ctrl Pts',(170.431637643182,24.8757620427769,172.503201159225));
#96713=CARTESIAN_POINT('Ctrl Pts',(170.147366737827,24.8757620425845,172.841271863791));
#96714=CARTESIAN_POINT('Ctrl Pts',(169.855890926735,24.8757620424782,173.174829191376));
#96715=CARTESIAN_POINT('Ctrl Pts',(169.691001898707,24.8757620424181,173.363523901001));
#96716=CARTESIAN_POINT('Ctrl Pts',(169.523598843296,24.8757620423814,173.550986300062));
#96717=CARTESIAN_POINT('Ctrl Pts',(169.354192863934,24.8757620423652,173.73672056851));
#96718=CARTESIAN_POINT('Ctrl Pts',(169.224305057717,24.8757620423528,173.879127682821));
#96719=CARTESIAN_POINT('Ctrl Pts',(169.093313104621,24.875762042345,174.020437340781));
#96720=CARTESIAN_POINT('Ctrl Pts',(168.96145390585,24.8757620423398,174.160423899149));
#96721=CARTESIAN_POINT('Ctrl Pts',(168.603675690039,24.8757620423257,174.540254366473));
#96722=CARTESIAN_POINT('Ctrl Pts',(168.239240001171,24.8757620423256,174.910770992204));
#96723=CARTESIAN_POINT('Ctrl Pts',(167.86832608009,24.875762042332,175.272717283235));
#96724=CARTESIAN_POINT('Ctrl Pts',(167.76110110206,24.8757620423338,175.377349870198));
#96725=CARTESIAN_POINT('Ctrl Pts',(167.653334541672,24.8757620423368,175.481265972554));
#96726=CARTESIAN_POINT('Ctrl Pts',(167.545030251731,24.8757620423426,175.584482916587));
#96727=CARTESIAN_POINT('Ctrl Pts',(167.391414817332,24.875762042351,175.73088261787));
#96728=CARTESIAN_POINT('Ctrl Pts',(167.236735452103,24.8757620423595,175.875857359385));
#96729=CARTESIAN_POINT('Ctrl Pts',(167.081018835541,24.8757620423659,176.019442844285));
#96730=CARTESIAN_POINT('Ctrl Pts',(165.977690059272,24.8757620424114,177.036816589251));
#96731=CARTESIAN_POINT('Ctrl Pts',(164.822456353684,24.8757620418276,177.984667554233));
#96732=CARTESIAN_POINT('Ctrl Pts',(163.622189357779,24.8757620429691,178.872211607));
#96733=CARTESIAN_POINT('Ctrl Pts',(163.418575347589,24.8757620431627,179.022775110304));
#96734=CARTESIAN_POINT('Ctrl Pts',(163.213663170986,24.8757620433069,179.171600306124));
#96735=CARTESIAN_POINT('Ctrl Pts',(163.007486724642,24.8757620433668,179.318732333689));
#96736=CARTESIAN_POINT('Ctrl Pts',(161.826761409925,24.8757620437098,180.161323777245));
#96737=CARTESIAN_POINT('Ctrl Pts',(160.604478799181,24.8757620422148,180.948253563706));
#96738=CARTESIAN_POINT('Ctrl Pts',(159.345247936767,24.8757620424794,181.685692517432));
#96739=CARTESIAN_POINT('Ctrl Pts',(159.088411572373,24.8757620425333,181.836102696765));
#96740=CARTESIAN_POINT('Ctrl Pts',(158.830038252835,24.8757620426851,181.984456843645));
#96741=CARTESIAN_POINT('Ctrl Pts',(158.570168232156,24.8757620431183,182.130802398217));
#96742=CARTESIAN_POINT('Ctrl Pts',(157.463233311892,24.8757620449639,182.754171744003));
#96743=CARTESIAN_POINT('Ctrl Pts',(156.32723882416,24.8757620554769,183.341433737248));
#96744=CARTESIAN_POINT('Ctrl Pts',(155.17857190235,24.8757620474239,183.890265373549));
#96745=CARTESIAN_POINT('Ctrl Pts',(155.043897412595,24.8757620464797,183.954612678392));
#96746=CARTESIAN_POINT('Ctrl Pts',(154.909048771853,24.8757620454079,184.018431744722));
#96747=CARTESIAN_POINT('Ctrl Pts',(154.774052417606,24.8757620444565,184.081718857687));
#96748=CARTESIAN_POINT('Origin',(-205.7,23.8757620423259,152.608250755187));
#96749=CARTESIAN_POINT('',(178.303739692644,24.8757620423259,152.608250755187));
#96750=CARTESIAN_POINT('',(-178.303739692644,23.8757620423259,151.608250755187));
#96751=CARTESIAN_POINT('Ctrl Pts',(111.133322854733,1.83216991269566,151.608250755187));
#96752=CARTESIAN_POINT('Ctrl Pts',(111.270341463106,0.841601439060684,151.608250755187));
#96753=CARTESIAN_POINT('Ctrl Pts',(111.270341463106,0.841601439060711,150.608250755187));
#96754=CARTESIAN_POINT('Ctrl Pts',(106.548434494274,1.19797344937741,151.608250755187));
#96755=CARTESIAN_POINT('Ctrl Pts',(106.671764202407,0.205511483093893,151.608250755379));
#96756=CARTESIAN_POINT('Ctrl Pts',(106.671764202405,0.205511483112742,150.608250755315));
#96757=CARTESIAN_POINT('Ctrl Pts',(101.948195700743,0.65791952309158,151.608250755187));
#96758=CARTESIAN_POINT('Ctrl Pts',(102.059566500144,-0.335917557920184,
151.608250755122));
#96759=CARTESIAN_POINT('Ctrl Pts',(102.059566500147,-0.335917557951168,
150.608250755122));
#96760=CARTESIAN_POINT('Ctrl Pts',(92.723767631763,-0.275480355398272,151.608250755187));
#96761=CARTESIAN_POINT('Ctrl Pts',(92.8137443254523,-1.27148225958765,151.608250755251));
#96762=CARTESIAN_POINT('Ctrl Pts',(92.8137443254492,-1.27148225955667,150.608250755251));
#96763=CARTESIAN_POINT('Ctrl Pts',(88.0977465730908,-0.668756637725884,
151.608250755187));
#96764=CARTESIAN_POINT('Ctrl Pts',(88.1782833145606,-1.66554450169544,151.608250755187));
#96765=CARTESIAN_POINT('Ctrl Pts',(88.1782833146266,-1.66554450171365,150.608250755187));
#96766=CARTESIAN_POINT('Ctrl Pts',(74.2033680985811,-1.6726098062369,151.608250755187));
#96767=CARTESIAN_POINT('Ctrl Pts',(74.2584777381936,-2.67123474963045,151.608250755187));
#96768=CARTESIAN_POINT('Ctrl Pts',(74.2584777380615,-2.67123474959403,150.608250755187));
#96769=CARTESIAN_POINT('Ctrl Pts',(64.9347005236076,-2.10826818027943,151.608250755187));
#96770=CARTESIAN_POINT('Ctrl Pts',(64.9766672764937,-3.10744308241369,151.608250755187));
#96771=CARTESIAN_POINT('Ctrl Pts',(64.9766672764947,-3.10744308244679,150.608250755187));
#96772=CARTESIAN_POINT('Ctrl Pts',(46.3902608861325,-2.69091503172259,151.608250755187));
#96773=CARTESIAN_POINT('Ctrl Pts',(46.411101044151,-3.69075370931775,151.608250755187));
#96774=CARTESIAN_POINT('Ctrl Pts',(46.41110104415,-3.69075370928465,150.608250755187));
#96775=CARTESIAN_POINT('Ctrl Pts',(37.1144344070604,-2.83569245393131,151.608250755187));
#96776=CARTESIAN_POINT('Ctrl Pts',(37.1273040291325,-3.83562452408217,151.6082507548));
#96777=CARTESIAN_POINT('Ctrl Pts',(37.1273040291327,-3.83562452423629,150.608250754929));
#96778=CARTESIAN_POINT('Ctrl Pts',(18.5590407294506,-2.97325419480569,151.608250755187));
#96779=CARTESIAN_POINT('Ctrl Pts',(18.5609978432699,-3.97326716587542,151.608250755573));
#96780=CARTESIAN_POINT('Ctrl Pts',(18.5609978432698,-3.9732671657213,150.608250755444));
#96781=CARTESIAN_POINT('Ctrl Pts',(9.27942897160271,-2.96262874564539,151.608250755187));
#96782=CARTESIAN_POINT('Ctrl Pts',(9.27841046030881,-3.9626287456454,151.608250755187));
#96783=CARTESIAN_POINT('Ctrl Pts',(9.27841046030894,-3.96262874552467,150.608250755187));
#96784=CARTESIAN_POINT('Ctrl Pts',(7.59225281309826E-15,-2.96262874552467,
151.608250755187));
#96785=CARTESIAN_POINT('Ctrl Pts',(7.71069817591099E-15,-3.96262874552467,
151.608250755187));
#96786=CARTESIAN_POINT('Ctrl Pts',(7.71069817591099E-15,-3.96262874552467,
150.608250755187));
#96787=CARTESIAN_POINT('Ctrl Pts',(110.612002249452,0.751198971720865,150.608250755187));
#96788=CARTESIAN_POINT('Ctrl Pts',(106.050488567514,0.129377001469773,150.608250755187));
#96789=CARTESIAN_POINT('Ctrl Pts',(101.47400078582,-0.400723078925373,150.608250755187));
#96790=CARTESIAN_POINT('Ctrl Pts',(92.2976017204801,-1.31744564164295,150.608250755187));
#96791=CARTESIAN_POINT('Ctrl Pts',(87.6963246266761,-1.70397824638163,150.608250755187));
#96792=CARTESIAN_POINT('Ctrl Pts',(73.8738846253088,-2.69123907257862,150.608250755187));
#96793=CARTESIAN_POINT('Ctrl Pts',(64.6442699267499,-3.12078579779498,150.608250755187));
#96794=CARTESIAN_POINT('Ctrl Pts',(46.1823666336506,-3.69495161107092,150.608250755187));
#96795=CARTESIAN_POINT('Ctrl Pts',(36.9474605582068,-3.83767561637138,150.608250755187));
#96796=CARTESIAN_POINT('Ctrl Pts',(18.4738883141652,-3.97318469247364,150.608250755187));
#96797=CARTESIAN_POINT('Ctrl Pts',(9.23693273607507,-3.96262874552467,150.608250755187));
#96798=CARTESIAN_POINT('Ctrl Pts',(7.71069817591099E-15,-3.96262874552467,
150.608250755187));
#96799=CARTESIAN_POINT('Origin',(-205.7,-9.35236728728476,151.608250755187));
#96800=CARTESIAN_POINT('Origin',(-205.7,24.8757620423259,209.282162333937));
#96801=CARTESIAN_POINT('Ctrl Pts',(96.5581428144939,29.1702255611255,195.428125979215));
#96802=CARTESIAN_POINT('Ctrl Pts',(96.7311023279802,27.510923329495,195.422864721506));
#96803=CARTESIAN_POINT('Ctrl Pts',(96.8973711956851,25.8618521564905,195.232745022291));
#96804=CARTESIAN_POINT('Ctrl Pts',(92.4415169449766,28.7565333888699,195.553349675513));
#96805=CARTESIAN_POINT('Ctrl Pts',(92.5976675800192,27.0947339894513,195.549474400368));
#96806=CARTESIAN_POINT('Ctrl Pts',(92.7481683291537,25.4431914874834,195.360541294257));
#96807=CARTESIAN_POINT('Ctrl Pts',(88.3520507412781,28.4030914565636,195.64700268798));
#96808=CARTESIAN_POINT('Ctrl Pts',(88.4934425831405,26.7395278446426,195.64402437791));
#96809=CARTESIAN_POINT('Ctrl Pts',(88.6300070463228,25.0862367508384,195.455861695539));
#96810=CARTESIAN_POINT('Ctrl Pts',(80.2076413227381,27.7915957659344,195.794185887528));
#96811=CARTESIAN_POINT('Ctrl Pts',(80.3223216239699,26.125270179941,195.792536551935));
#96812=CARTESIAN_POINT('Ctrl Pts',(80.4335599248988,24.4692428089101,195.605516960837));
#96813=CARTESIAN_POINT('Ctrl Pts',(76.1526889733453,27.5336304760513,195.847553658596));
#96814=CARTESIAN_POINT('Ctrl Pts',(76.2554887724622,25.8663249070321,195.846327241293));
#96815=CARTESIAN_POINT('Ctrl Pts',(76.3554012815499,24.2093261329018,195.659672537072));
#96816=CARTESIAN_POINT('Ctrl Pts',(68.0652206896679,27.0943461905063,195.928468679087));
#96817=CARTESIAN_POINT('Ctrl Pts',(68.1465044178566,25.4255294368387,195.927853344985));
#96818=CARTESIAN_POINT('Ctrl Pts',(68.2258303093629,23.7670327953681,195.741726502934));
#96819=CARTESIAN_POINT('Ctrl Pts',(64.03279795575,26.9130916763118,195.955933585121));
#96820=CARTESIAN_POINT('Ctrl Pts',(64.1044855996088,25.2437500578336,195.955502808343));
#96821=CARTESIAN_POINT('Ctrl Pts',(64.1745855046219,23.5847329161387,195.769535871164));
#96822=CARTESIAN_POINT('Ctrl Pts',(55.9832533396131,26.6122137200978,195.994697701943));
#96823=CARTESIAN_POINT('Ctrl Pts',(56.0376446038494,24.9420845379358,195.994521322064));
#96824=CARTESIAN_POINT('Ctrl Pts',(56.0910584623061,23.282286359139,195.808775043));
#96825=CARTESIAN_POINT('Ctrl Pts',(51.9661782517966,26.4926340937108,196.005952434106));
#96826=CARTESIAN_POINT('Ctrl Pts',(52.0128883060383,24.8222448356165,196.005844390051));
#96827=CARTESIAN_POINT('Ctrl Pts',(52.0588588944913,23.1621886081543,195.820157585625));
#96828=CARTESIAN_POINT('Ctrl Pts',(39.9311373606373,26.2070303356449,196.025623827227));
#96829=CARTESIAN_POINT('Ctrl Pts',(39.9573441152576,24.5360837036126,196.025644384184));
#96830=CARTESIAN_POINT('Ctrl Pts',(39.9833816094678,22.8754744091628,195.840069630165));
#96831=CARTESIAN_POINT('Ctrl Pts',(31.9288875819601,26.1142952297546,196.020515138928));
#96832=CARTESIAN_POINT('Ctrl Pts',(31.9447866062045,24.4432653675089,196.020526192105));
#96833=CARTESIAN_POINT('Ctrl Pts',(31.9607025010364,22.7825732665138,195.834943371232));
#96834=CARTESIAN_POINT('Ctrl Pts',(15.947733524435,26.0285644344409,196.007873194612));
#96835=CARTESIAN_POINT('Ctrl Pts',(15.9497758197389,24.3574643678052,196.007876333974));
#96836=CARTESIAN_POINT('Ctrl Pts',(15.9519837644084,22.6967024452114,195.822286623132));
#96837=CARTESIAN_POINT('Ctrl Pts',(7.96912902423969,26.0373712549187,196.));
#96838=CARTESIAN_POINT('Ctrl Pts',(7.96761387059107,24.3662859578773,196.000000000019));
#96839=CARTESIAN_POINT('Ctrl Pts',(7.96622304565945,22.7055386933791,195.814407453179));
#96840=CARTESIAN_POINT('Ctrl Pts',(1.578508351368E-14,26.0373712544753,
196.));
#96841=CARTESIAN_POINT('Ctrl Pts',(1.58962544981566E-14,24.3662859574616,
196.));
#96842=CARTESIAN_POINT('Ctrl Pts',(1.59444394375923E-14,22.7055386929907,
195.814407453146));
#96843=CARTESIAN_POINT('Ctrl Pts',(1.4210854715202E-14,26.0373712544753,
196.));
#96844=CARTESIAN_POINT('Ctrl Pts',(3.98999039555811,26.0373712544753,196.));
#96845=CARTESIAN_POINT('Ctrl Pts',(7.98016079670639,26.0351684189602,196.001973114377));
#96846=CARTESIAN_POINT('Ctrl Pts',(11.9700380568879,26.0383329718934,196.004732891428));
#96847=CARTESIAN_POINT('Ctrl Pts',(15.4357914559827,26.0410818183792,196.00713013477));
#96848=CARTESIAN_POINT('Ctrl Pts',(18.9013236137276,26.0478805596461,196.010120892553));
#96849=CARTESIAN_POINT('Ctrl Pts',(22.3663201987643,26.0636449968344,196.012933146671));
#96850=CARTESIAN_POINT('Ctrl Pts',(22.8903296073034,26.0660290434573,196.013358442218));
#96851=CARTESIAN_POINT('Ctrl Pts',(23.414326759107,26.0686180422282,196.013779667672));
#96852=CARTESIAN_POINT('Ctrl Pts',(23.9383105582663,26.071428887833,196.014194166774));
#96853=CARTESIAN_POINT('Ctrl Pts',(23.9724687182037,26.071612125013,196.014221187698));
#96854=CARTESIAN_POINT('Ctrl Pts',(24.0066268159181,26.0717962720147,196.014248186252));
#96855=CARTESIAN_POINT('Ctrl Pts',(24.0407848516479,26.0719813325248,196.014275161106));
#96856=CARTESIAN_POINT('Ctrl Pts',(27.1918482515225,26.0890530811696,196.016763579223));
#96857=CARTESIAN_POINT('Ctrl Pts',(30.3424154561325,26.1139030681914,196.019049376945));
#96858=CARTESIAN_POINT('Ctrl Pts',(33.492298128033,26.1494014787918,196.020095240139));
#96859=CARTESIAN_POINT('Ctrl Pts',(36.4310110091503,26.1825200572776,196.021070988114));
#96860=CARTESIAN_POINT('Ctrl Pts',(39.369128099848,26.2249073749037,196.020967358996));
#96861=CARTESIAN_POINT('Ctrl Pts',(42.3064876248667,26.2788516104082,196.018953311004));
#96862=CARTESIAN_POINT('Ctrl Pts',(44.1894841856694,26.3134326036659,196.017662204004));
#96863=CARTESIAN_POINT('Ctrl Pts',(46.0721692493293,26.3527620049448,196.015586250003));
#96864=CARTESIAN_POINT('Ctrl Pts',(47.9544979792259,26.3974318154924,196.012509565106));
#96865=CARTESIAN_POINT('Ctrl Pts',(47.9907577661141,26.3982923016472,196.012450298127));
#96866=CARTESIAN_POINT('Ctrl Pts',(48.0270174302833,26.3991547660561,196.012390648295));
#96867=CARTESIAN_POINT('Ctrl Pts',(48.0632769722344,26.4000192132909,196.012330613117));
#96868=CARTESIAN_POINT('Ctrl Pts',(50.5137145742306,26.4584389807552,196.008273406405));
#96869=CARTESIAN_POINT('Ctrl Pts',(52.963664586409,26.5259196423555,196.002454852829));
#96870=CARTESIAN_POINT('Ctrl Pts',(55.4128930506474,26.6038431345442,195.994113042992));
#96871=CARTESIAN_POINT('Ctrl Pts',(56.944906486256,26.6525849480279,195.988895169309));
#96872=CARTESIAN_POINT('Ctrl Pts',(58.4766373725112,26.7054118064935,195.982690335751));
#96873=CARTESIAN_POINT('Ctrl Pts',(60.0080256579301,26.7626524267857,195.975315643483));
#96874=CARTESIAN_POINT('Ctrl Pts',(62.218848643179,26.8452891298589,195.964669003875));
#96875=CARTESIAN_POINT('Ctrl Pts',(64.4289443566986,26.9371137869464,195.951596468763));
#96876=CARTESIAN_POINT('Ctrl Pts',(66.6383460860964,27.0392640263435,195.935316684546));
#96877=CARTESIAN_POINT('Ctrl Pts',(68.4417010588521,27.1226409603496,195.92202882049));
#96878=CARTESIAN_POINT('Ctrl Pts',(70.2445934657614,27.2128963010836,195.906604522875));
#96879=CARTESIAN_POINT('Ctrl Pts',(72.0470329001817,27.3106267279901,195.888629690922));
#96880=CARTESIAN_POINT('Ctrl Pts',(72.0676736114691,27.3117458921002,195.888423851375));
#96881=CARTESIAN_POINT('Ctrl Pts',(72.0883142769542,27.3128660370197,195.888217677336));
#96882=CARTESIAN_POINT('Ctrl Pts',(72.1089548960627,27.3139871636003,195.888011168196));
#96883=CARTESIAN_POINT('Ctrl Pts',(73.9322669317684,27.4130231264906,195.86976895369));
#96884=CARTESIAN_POINT('Ctrl Pts',(75.7551996644265,27.5197096363461,195.848926770467));
#96885=CARTESIAN_POINT('Ctrl Pts',(77.577565779252,27.6347862725935,195.824854974109));
#96886=CARTESIAN_POINT('Ctrl Pts',(79.326413066646,27.7452204282258,195.801754294493));
#96887=CARTESIAN_POINT('Ctrl Pts',(81.0747386415879,27.8633814946748,195.775679190743));
#96888=CARTESIAN_POINT('Ctrl Pts',(82.8223589117719,27.9898836032052,195.746094692498));
#96889=CARTESIAN_POINT('Ctrl Pts',(83.3082440207675,28.0250545678822,195.737869411869));
#96890=CARTESIAN_POINT('Ctrl Pts',(83.7940744942396,28.060870038313,195.729372997879));
#96891=CARTESIAN_POINT('Ctrl Pts',(84.2798461077883,28.0973426261767,195.720594286385));
#96892=CARTESIAN_POINT('Ctrl Pts',(85.8745187030419,28.2170734517788,195.691775865854));
#96893=CARTESIAN_POINT('Ctrl Pts',(87.4685601335887,28.343875044827,195.659938145996));
#96894=CARTESIAN_POINT('Ctrl Pts',(89.0620397243112,28.4783563924592,195.624449393539));
#96895=CARTESIAN_POINT('Ctrl Pts',(90.6059337456486,28.608652977241,195.590064972765));
#96896=CARTESIAN_POINT('Ctrl Pts',(92.149300428614,28.7461588482606,195.552253116234));
#96897=CARTESIAN_POINT('Ctrl Pts',(93.6921811470376,28.8913921093023,195.510464455059));
#96898=CARTESIAN_POINT('Ctrl Pts',(94.4512527163619,28.9628444504072,195.489905131037));
#96899=CARTESIAN_POINT('Ctrl Pts',(95.2102063150246,29.0361666270266,195.468383631185));
#96900=CARTESIAN_POINT('Ctrl Pts',(95.969044764986,29.1114169499324,195.445836982328));
#96901=CARTESIAN_POINT('Ctrl Pts',(7.71069817591099E-15,-3.96262874552467,
150.608250755187));
#96902=CARTESIAN_POINT('Ctrl Pts',(7.71069817591099E-15,-3.96262874552467,
19.0783498489627));
#96903=CARTESIAN_POINT('Ctrl Pts',(32.8608169036053,-3.96262874552466,150.608250755187));
#96904=CARTESIAN_POINT('Ctrl Pts',(32.8608169036053,-3.96262874552466,19.0783498489627));
#96905=CARTESIAN_POINT('Ctrl Pts',(74.5903827540722,-4.15923996764941,150.608250755187));
#96906=CARTESIAN_POINT('Ctrl Pts',(74.5903827540722,-4.15923996764941,19.0783498489627));
#96907=CARTESIAN_POINT('Ctrl Pts',(110.612002249464,0.751198971722513,150.608250755187));
#96908=CARTESIAN_POINT('Ctrl Pts',(110.612002249464,0.751198971722513,19.0783498489627));
#96909=CARTESIAN_POINT('Ctrl Pts',(1.58070730646102E-14,25.8648855730305,
196.));
#96910=CARTESIAN_POINT('Ctrl Pts',(1.14416717392176E-14,60.1070228853939,
196.));
#96911=CARTESIAN_POINT('Ctrl Pts',(53.668246544272,25.8648855730305,196.));
#96912=CARTESIAN_POINT('Ctrl Pts',(53.668246544272,60.1070228853939,196.));
#96913=CARTESIAN_POINT('Ctrl Pts',(92.2273133188686,25.8648855730305,196.338082381737));
#96914=CARTESIAN_POINT('Ctrl Pts',(92.2273133188686,60.1070228853939,196.338082381737));
#96915=CARTESIAN_POINT('Ctrl Pts',(119.928096709094,25.8648855730305,194.270533336501));
#96916=CARTESIAN_POINT('Ctrl Pts',(119.928096709094,60.1070228853939,194.270533336501));
#96917=CARTESIAN_POINT('Origin',(-205.7,23.8757620423259,152.608250755187));
#96918=CARTESIAN_POINT('',(178.303739692644,24.8757620423259,152.608250755187));
#96919=CARTESIAN_POINT('Origin',(-205.7,23.8757620423259,152.608250755187));
#96920=CARTESIAN_POINT('',(178.303739692644,24.8757620423259,152.608250755187));
#96921=CARTESIAN_POINT('Origin',(-205.7,23.8757620423259,152.608250755187));
#96922=CARTESIAN_POINT('',(178.303739692644,24.8757620423259,152.608250755187));
#96923=CARTESIAN_POINT('Origin',(-205.7,23.8757620423259,152.608250755187));
#96924=CARTESIAN_POINT('',(178.303739692644,24.8757620423259,152.608250755187));
#96925=CARTESIAN_POINT('Origin',(-205.7,24.8757620423259,209.282162333937));
#130895=UNCERTAINTY_MEASURE_WITH_UNIT(LENGTH_MEASURE(0.01),#130911,
'DISTANCE_ACCURACY_VALUE',
'Maximum model space distance between geometric entities at asserted c
onnectivities');
#130900=UNCERTAINTY_MEASURE_WITH_UNIT(LENGTH_MEASURE(0.01),#130911,
'DISTANCE_ACCURACY_VALUE',
'Maximum model space distance between geometric entities at asserted c
onnectivities');
#130905=(
GEOMETRIC_REPRESENTATION_CONTEXT(3)
GLOBAL_UNCERTAINTY_ASSIGNED_CONTEXT((#130895))
GLOBAL_UNIT_ASSIGNED_CONTEXT((#130911,#130913,#130914))
REPRESENTATION_CONTEXT('','3D')
);
#130910=(
GEOMETRIC_REPRESENTATION_CONTEXT(3)
GLOBAL_UNCERTAINTY_ASSIGNED_CONTEXT((#130900))
GLOBAL_UNIT_ASSIGNED_CONTEXT((#130911,#130913,#130914))
REPRESENTATION_CONTEXT('','3D')
);
#130911=(
LENGTH_UNIT()
NAMED_UNIT(*)
SI_UNIT(.MILLI.,.METRE.)
);
#130913=(
NAMED_UNIT(*)
PLANE_ANGLE_UNIT()
SI_UNIT($,.RADIAN.)
);
#130914=(
NAMED_UNIT(*)
SI_UNIT($,.STERADIAN.)
SOLID_ANGLE_UNIT()
);
#130919=SHAPE_DEFINITION_REPRESENTATION(#130928,#130945);
#130928=PRODUCT_DEFINITION_SHAPE('',$,#130955);
#130945=SHAPE_REPRESENTATION('',(#48162),#130905);
#130950=PRODUCT_DEFINITION_CONTEXT('part definition',#130979,'design');
#130955=PRODUCT_DEFINITION('2026-10-06-10-46-07-206','Component4',#130964,
#130950);
#130964=PRODUCT_DEFINITION_FORMATION('',$,#130985);
#130979=APPLICATION_CONTEXT(
'Core Data for Automotive Mechanical Design Process');
#130980=PRODUCT_CONTEXT('part definition',#130979,'mechanical');
#130985=PRODUCT('2026-10-06-10-46-07-206','Component4',$,(#130980));
#130991=PRESENTATION_STYLE_ASSIGNMENT((#130993));
#130993=SURFACE_STYLE_USAGE(.BOTH.,#130995);
#130995=SURFACE_SIDE_STYLE('',(#130997));
#130997=SURFACE_STYLE_FILL_AREA(#130999);
#130999=FILL_AREA_STYLE('Opaque(202,209,238)',(#131001));
#131001=FILL_AREA_STYLE_COLOUR('Opaque(202,209,238)',#131003);
#131003=COLOUR_RGB('Opaque(202,209,238)', 0.40784314, 0.44705882, 0.49803922);
ENDSEC;
END-ISO-10303-21;
